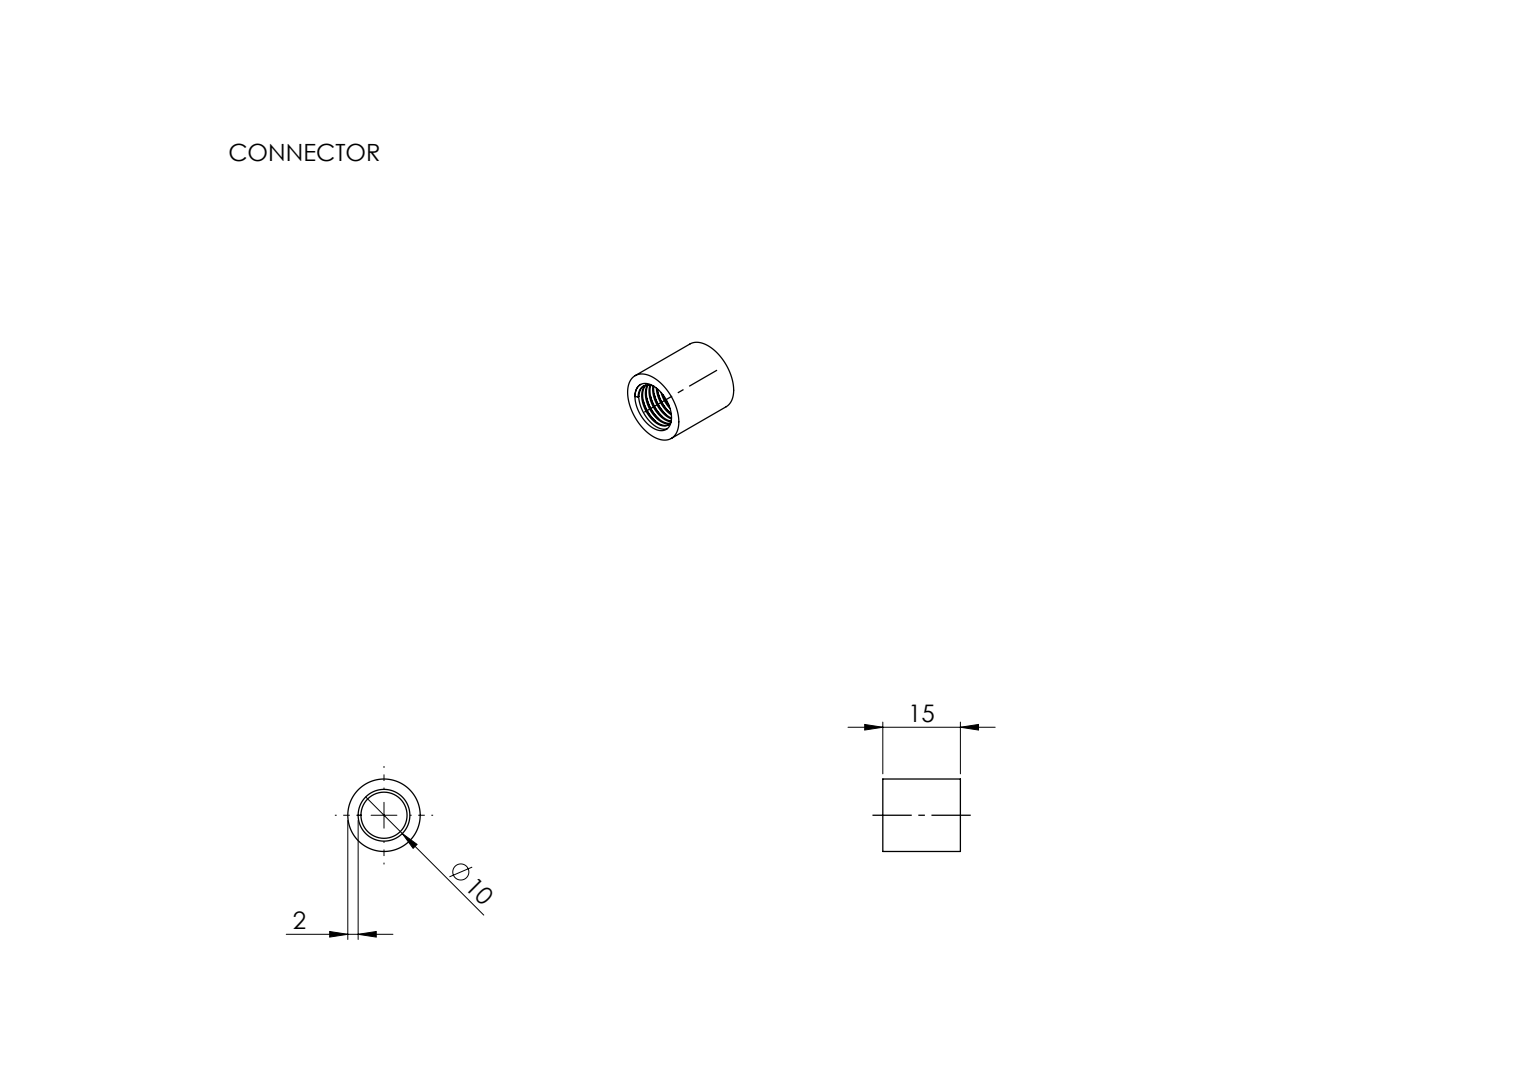
ISO-10303-21;
HEADER;
FILE_DESCRIPTION (('STEP AP214'),
    '1' );
FILE_NAME ('connector.step',
    '2026-10-01T14:18:43',
    ( '' ),
    ( '' ),
    'SwSTEP 2.0',
    'SolidWorks 2026',
    '' );
FILE_SCHEMA (( 'AUTOMOTIVE_DESIGN' ));
ENDSEC;

DATA;
#9=CARTESIAN_POINT ( 'NONE',  ( 101.8468681455906903, 4.458734125000016313, 4.375000001365592084 ) ) ;
#16=CARTESIAN_POINT ( 'NONE',  ( 94.99999999999995737, 1.387778780781445676E-14, 4.999999999999999112 ) ) ;
#25=CARTESIAN_POINT ( 'NONE',  ( 95.54126587499996504, 1.387778780781445676E-14, 10.68750000136559208 ) ) ;
#27=CARTESIAN_POINT ( 'NONE',  ( 99.99999999999995737, -4.458734124999988779, 1.687500001365591418 ) ) ;
#43=CARTESIAN_POINT ( 'NONE',  ( 104.4587341249999781, -1.846868145590721655, 14.12500000136559208 ) ) ;
#52=APPLICATION_CONTEXT ( 'automotive_design' ) ;
#61=CARTESIAN_POINT ( 'NONE',  ( 103.1528011352953342, -3.152801135295355106, 10.06250000136559386 ) ) ;
#74=CARTESIAN_POINT ( 'NONE',  ( 99.99999999999995737, -4.999999999999990230, 1.375000002731184612 ) ) ;
#80=EDGE_CURVE ( 'NONE', #16509, #7689, #8629, .T. ) ;
#91=CARTESIAN_POINT ( 'NONE',  ( 98.15313185440925281, 4.458734125000016313, 7.250000001365591196 ) ) ;
#94=CARTESIAN_POINT ( 'NONE',  ( 101.8468681455906903, -4.458734124999987891, 10.75000000136559208 ) ) ;
#102=CARTESIAN_POINT ( 'NONE',  ( 103.5355339059327093, 3.535533905932755072, 11.62500000000000000 ) ) ;
#104=CARTESIAN_POINT ( 'NONE',  ( 95.54126587499996504, 1.387778780781445676E-14, 0.6875000013655923059 ) ) ;
#107=DIRECTION ( 'NONE',  ( -1.000000000000000000, 0.000000000000000000, 0.000000000000000000 ) ) ;
#115=CARTESIAN_POINT ( 'NONE',  ( 102.0710678118654329, 5.000000000000018652, 4.687500000000000000 ) ) ;
#119=VECTOR ( 'NONE', #9370, 1000.000000000000000 ) ;
#132=CARTESIAN_POINT ( 'NONE',  ( 104.4587341249999781, 1.846868145590750521, 4.000000001365592084 ) ) ;
#150=CARTESIAN_POINT ( 'NONE',  ( 101.8468681455906903, -4.458734124999987891, 3.000000001365592528 ) ) ;
#162=VERTEX_POINT ( 'NONE', #19320 ) ;
#167=CARTESIAN_POINT ( 'NONE',  ( 96.84719886470459471, -3.152801135295355994, 12.81250000136559208 ) ) ;
#170=CARTESIAN_POINT ( 'NONE',  ( 103.1528011352953342, -3.152801135295355106, 0.8125000013655924169 ) ) ;
#172=CARTESIAN_POINT ( 'NONE',  ( 103.1528011352953342, -3.152801135295355106, 1.062500001365592528 ) ) ;
#177=ORIENTED_EDGE ( 'NONE', *, *, #19574, .T. ) ;
#201=CARTESIAN_POINT ( 'NONE',  ( 104.4587341249999781, -1.846868145590721655, 11.12500000136559208 ) ) ;
#207=CARTESIAN_POINT ( 'NONE',  ( 103.5355339059327093, -3.535533905932726206, 12.37499999999999822 ) ) ;
#219=FILL_AREA_STYLE ('',( #13008 ) ) ;
#227=VECTOR ( 'NONE', #13588, 1000.000000000000000 ) ;
#229=CARTESIAN_POINT ( 'NONE',  ( 95.54126587499995082, 1.846868145590750077, 10.37500000136559208 ) ) ;
#231=CARTESIAN_POINT ( 'NONE',  ( 95.54126587499995082, -1.846868145590724986, 13.50000000136559208 ) ) ;
#274=CARTESIAN_POINT ( 'NONE',  ( 99.99999999999995737, -4.458734124999988779, 1.687500001365591418 ) ) ;
#282=ORIENTED_EDGE ( 'NONE', *, *, #1152, .F. ) ;
#293=CARTESIAN_POINT ( 'NONE',  ( 101.8468681455906903, 4.458734125000016313, 3.375000001365592972 ) ) ;
#295=EDGE_LOOP ( 'NONE', ( #18742, #1157, #17267, #23427 ) ) ;
#309=CARTESIAN_POINT ( 'NONE',  ( 101.8468681455906903, -4.458734124999987891, 13.00000000136559386 ) ) ;
#311=CARTESIAN_POINT ( 'NONE',  ( 95.54126587499995082, -1.846868145590724986, 0.5000000013655920839 ) ) ;
#313=CARTESIAN_POINT ( 'NONE',  ( 104.9999999999999716, 1.449011120738813565E-14, 5.625000002731185056 ) ) ;
#328=CARTESIAN_POINT ( 'NONE',  ( 104.4587341249999781, -1.846868145590721655, 13.12500000136559208 ) ) ;
#345=CARTESIAN_POINT ( 'NONE',  ( 98.15313185440923860, -4.458734124999987891, 12.87500000136559208 ) ) ;
#374=ORIENTED_EDGE ( 'NONE', *, *, #22029, .T. ) ;
#375=CARTESIAN_POINT ( 'NONE',  ( 95.54126587499996504, 1.387778780781445676E-14, 7.437500001365592084 ) ) ;
#378=CARTESIAN_POINT ( 'NONE',  ( 95.54126587499995082, 1.846868145590750077, 7.375000001365592084 ) ) ;
#396=CARTESIAN_POINT ( 'NONE',  ( 99.99999999999995737, -4.999999999999990230, 10.37500000273118594 ) ) ;
#418=CARTESIAN_POINT ( 'NONE',  ( 101.8468681455907046, -4.458734124999987891, 3.750000001365591640 ) ) ;
#433=ORIENTED_EDGE ( 'NONE', *, *, #23597, .T. ) ;
#435=CARTESIAN_POINT ( 'NONE',  ( 96.46446609406721961, 3.535533905932755072, 11.87500000000000000 ) ) ;
#442=CARTESIAN_POINT ( 'NONE',  ( 99.99999999999995737, 1.387778780781445676E-14, 34.79898987322334136 ) ) ;
#452=CARTESIAN_POINT ( 'NONE',  ( 103.1528011352953342, 3.152801135295383084, 11.31250000136559386 ) ) ;
#454=CARTESIAN_POINT ( 'NONE',  ( 96.84719886470459471, -3.152801135295355994, 0.5625000013655921949 ) ) ;
#456=CARTESIAN_POINT ( 'NONE',  ( 101.8468681455907046, -4.458734124999987891, 1.000000001365592528 ) ) ;
#469=CARTESIAN_POINT ( 'NONE',  ( 104.4587341249999781, -1.846868145590721655, 12.12500000136559208 ) ) ;
#489=CARTESIAN_POINT ( 'NONE',  ( 98.15313185440923860, -4.458734124999987891, 11.87500000136559208 ) ) ;
#502=ORIENTED_EDGE ( 'NONE', *, *, #15207, .F. ) ;
#507=CARTESIAN_POINT ( 'NONE',  ( 94.99999999999995737, 1.387778780781445676E-14, 34.79898987322334136 ) ) ;
#509=CARTESIAN_POINT ( 'NONE',  ( 99.99999999999995737, -4.999999999999990230, 1.375000002731184612 ) ) ;
#514=DIRECTION ( 'NONE',  ( -1.000000000000000000, 0.000000000000000000, 0.000000000000000000 ) ) ;
#517=CARTESIAN_POINT ( 'NONE',  ( 95.54126587499995082, -1.846868145590724986, 3.500000001365591196 ) ) ;
#520=CARTESIAN_POINT ( 'NONE',  ( 95.54126587499995082, 1.846868145590750077, 9.375000001365592084 ) ) ;
#528=CARTESIAN_POINT ( 'NONE',  ( 104.9999999999999716, 1.449011120738813565E-14, 34.79898987322334136 ) ) ;
#532=ORIENTED_EDGE ( 'NONE', *, *, #5026, .F. ) ;
#537=CARTESIAN_POINT ( 'NONE',  ( 97.92893218813451028, -4.999999999999989342, 8.312500002731185944 ) ) ;
#579=( BOUNDED_SURFACE ( )  B_SPLINE_SURFACE ( 1, 2, ( 
 ( #14484, #7804, #25599, #1404, #3808, #3950, #3385, #8074, #3536, #18775, #16634, #25327, #10196, #25188, #14203, #7938, #27346, #18906, #19188, #18641, #12055, #16494, #27890, #10335, #5676, #23201, #25740, #23333, #27482, #12610, #10063, #23472, #8351, #5813, #14341, #23058, #6085, #12468, #12192, #16770, #12339, #3676, #20921, #27617, #1678, #5949, #25470, #21193, #14616, #9926, #19044, #20781, #1263, #27752, #8213, #16902, #1815, #10480, #17037, #6772, #21759, #11035, #19745, #26021, #26310, #229, #15029, #4507, #1950, #6629, #17754, #23747, #15458, #10757, #24172, #4649, #10620, #17327, #9059, #6223, #10898, #23610, #8915, #14890, #19469, #28029, #17604, #28168, #6492, #21903, #12882, #4087, #8636, #19325, #13164, #21612, #2377, #2088, #12751, #15168, #23887, #4365, #13308, #22035, #2511, #11172, #19606, #19891, #13022, #21474, #8495, #2236, #375, #17180, #4223, #91, #8772, #17461, #26163, #25886, #6355, #15314, #24029, #22176, #948, #26888, #2927, #15602, #3078, #6911, #2792, #20038, #11743, #11459, #18028, #13882, #4935, #24305, #20178, #11316, #24736, #13598, #5217, #22321, #1092, #662, #9335, #26742, #18324, #5359, #24880, #14025, #11597, #9619, #7184, #4791, #9759, #13738, #27031, #22750, #7046, #24598, #15882, #20319, #15744, #26457, #13449, #9475, #7477, #2655, #16172, #7334, #3216, #5077, #18177, #517, #9198, #17892, #11882, #22608, #22462, #20607, #807, #26600, #16023, #24449, #20469, #4163, #12025, #7904, #5778, #15100, #14967, #9896, #23686, #20749, #12688, #12958, #18607, #27442, #2165, #27965, #23026, #17258, #14305, #28103, #4300, #10031, #1233, #27312, #10692, #17111, #7769, #21413, #16599, #18743, #16456, #4022, #6290, #10556, #25151, #8421, #5641, #14170, #12160 ),
 ( #25815, #19398, #14447, #12823, #21549, #25291, #8567, #2023, #3496, #25958, #22888, #19266, #18469, #20886, #6431, #1370, #23822, #21692, #3353, #23545, #27176, #7628, #1892, #16320, #25021, #5502, #9133, #309, #2449, #6702, #167, #15823, #2593, #13095, #24529, #17969, #26243, #13385, #20116, #9273, #8849, #13240, #23964, #11397, #21836, #22257, #17687, #6845, #4872, #11254, #2732, #19973, #2312, #10969, #452, #21972, #4725, #26678, #11110, #4443, #594, #15390, #17826, #7126, #25, #22113, #17539, #24102, #19824, #8994, #26392, #19681, #10828, #4580, #15535, #24243, #5014, #15243, #19544, #26531, #6987, #15682, #24383, #13536, #13679, #22396, #8707, #17399, #26098, #6563, #14386, #7704, #12098, #5720, #9412, #16107, #16253, #7559, #18683, #20402, #5582, #25096, #7413, #22685, #2865, #1030, #24952, #15961, #3431, #20689, #18111, #1172, #24676, #887, #26825, #14247, #9701, #27386, #7271, #5438, #16398, #14106, #20548, #22969, #22829, #3296, #20825, #11966, #5154, #18402, #11535, #13959, #20251, #1302, #9971, #18544, #3155, #9837, #24811, #5295, #9558, #27248, #7845, #16540, #27108, #11825, #738, #25230, #13816, #22539, #3007, #11679, #18260, #26968, #27796, #7977, #23653, #12655, #10103, #21380, #16676, #12378, #18815, #6259, #21237, #10659, #1445, #8253, #27931, #6124, #12508, #14932, #14790, #23513, #4128, #3992, #27522, #1719, #25926, #5990, #3577, #8390, #1992, #10523, #23375, #1859, #8119, #27657, #1585, #19230, #16940, #17076, #10381, #25510, #23103, #25781, #19088, #12794, #25375, #21512, #25641, #5855, #19366, #28069, #14655, #18948, #21097, #8535, #17221, #14525, #6400, #12234, #10239, #20962, #23240, #3717, #16813, #3848, #16312, #15650, #26063, #26498, #21942, #11078, #9101 ) ),
 .UNSPECIFIED., .F., .F., .F. ) 
 B_SPLINE_SURFACE_WITH_KNOTS ( ( 2, 2 ),
 ( 3, 2, 2, 2, 2, 2, 2, 2, 2, 2, 2, 2, 2, 2, 2, 2, 2, 2, 2, 2, 2, 2, 2, 2, 2, 2, 2, 2, 2, 2, 2, 2, 2, 2, 2, 2, 2, 2, 2, 2, 2, 2, 2, 2, 2, 2, 2, 2, 2, 2, 2, 2, 2, 2, 2, 2, 2, 2, 2, 2, 2, 2, 2, 2, 2, 2, 2, 2, 2, 2, 2, 2, 2, 2, 2, 2, 2, 2, 2, 2, 2, 2, 2, 2, 2, 2, 2, 2, 2, 2, 2, 2, 2, 2, 2, 2, 2, 2, 2, 2, 2, 2, 2, 2, 2, 2, 2, 2, 2, 2, 2, 2, 3 ),
 ( 0.000000000000000000, 1.000000000000000000 ),
 ( 0.000000000000000000, 0.008928571428571428076, 0.01785714285714285615, 0.02678571428571428423, 0.03571428571428571230, 0.04464285714285714385, 0.05357142857142856845, 0.06250000000000000000, 0.07142857142857142461, 0.08035714285714286309, 0.08928571428571428770, 0.09821428571428571230, 0.1071428571428571369, 0.1160714285714285754, 0.1250000000000000000, 0.1339285714285714246, 0.1428571428571428492, 0.1517857142857142738, 0.1607142857142857262, 0.1696428571428571508, 0.1785714285714285754, 0.1875000000000000000, 0.1964285714285714246, 0.2053571428571428492, 0.2142857142857142738, 0.2232142857142857262, 0.2321428571428571508, 0.2410714285714285754, 0.2500000000000000000, 0.2589285714285714524, 0.2678571428571428492, 0.2767857142857143016, 0.2857142857142856984, 0.2946428571428571508, 0.3035714285714285476, 0.3125000000000000000, 0.3214285714285714524, 0.3303571428571428492, 0.3392857142857143016, 0.3482142857142856984, 0.3571428571428571508, 0.3660714285714285476, 0.3750000000000000000, 0.3839285714285714524, 0.3928571428571428492, 0.4017857142857143016, 0.4107142857142856984, 0.4196428571428571508, 0.4285714285714285476, 0.4375000000000000000, 0.4464285714285714524, 0.4553571428571428492, 0.4642857142857143016, 0.4732142857142856984, 0.4821428571428571508, 0.4910714285714285476, 0.5000000000000000000, 0.5089285714285713969, 0.5178571428571429047, 0.5267857142857143016, 0.5357142857142856984, 0.5446428571428570953, 0.5535714285714286031, 0.5625000000000000000, 0.5714285714285713969, 0.5803571428571429047, 0.5892857142857143016, 0.5982142857142856984, 0.6071428571428570953, 0.6160714285714286031, 0.6250000000000000000, 0.6339285714285713969, 0.6428571428571429047, 0.6517857142857143016, 0.6607142857142856984, 0.6696428571428570953, 0.6785714285714286031, 0.6875000000000000000, 0.6964285714285713969, 0.7053571428571429047, 0.7142857142857143016, 0.7232142857142856984, 0.7321428571428570953, 0.7410714285714286031, 0.7500000000000000000, 0.7589285714285713969, 0.7678571428571429047, 0.7767857142857143016, 0.7857142857142856984, 0.7946428571428570953, 0.8035714285714286031, 0.8125000000000000000, 0.8214285714285713969, 0.8303571428571429047, 0.8392857142857143016, 0.8482142857142856984, 0.8571428571428570953, 0.8660714285714286031, 0.8750000000000000000, 0.8839285714285713969, 0.8928571428571429047, 0.9017857142857143016, 0.9107142857142856984, 0.9196428571428570953, 0.9285714285714286031, 0.9375000000000000000, 0.9464285714285713969, 0.9553571428571429047, 0.9642857142857143016, 0.9732142857142856984, 0.9821428571428570953, 0.9910714285714286031, 1.000000000000000000 ),
 .UNSPECIFIED. ) 
 GEOMETRIC_REPRESENTATION_ITEM ( )  RATIONAL_B_SPLINE_SURFACE ( (
 ( 1.000000000000000000, 0.9238795325112867385, 1.000000000000000000, 0.9238795325112867385, 1.000000000000000000, 0.9238795325112867385, 1.000000000000000000, 0.9238795325112867385, 1.000000000000000000, 0.9238795325112867385, 1.000000000000000000, 0.9238795325112867385, 1.000000000000000000, 0.9238795325112867385, 1.000000000000000000, 0.9238795325112867385, 1.000000000000000000, 0.9238795325112867385, 1.000000000000000000, 0.9238795325112867385, 1.000000000000000000, 0.9238795325112867385, 1.000000000000000000, 0.9238795325112867385, 1.000000000000000000, 0.9238795325112867385, 1.000000000000000000, 0.9238795325112867385, 1.000000000000000000, 0.9238795325112867385, 1.000000000000000000, 0.9238795325112867385, 1.000000000000000000, 0.9238795325112867385, 1.000000000000000000, 0.9238795325112867385, 1.000000000000000000, 0.9238795325112867385, 1.000000000000000000, 0.9238795325112867385, 1.000000000000000000, 0.9238795325112867385, 1.000000000000000000, 0.9238795325112867385, 1.000000000000000000, 0.9238795325112867385, 1.000000000000000000, 0.9238795325112867385, 1.000000000000000000, 0.9238795325112867385, 1.000000000000000000, 0.9238795325112867385, 1.000000000000000000, 0.9238795325112867385, 1.000000000000000000, 0.9238795325112867385, 1.000000000000000000, 0.9238795325112867385, 1.000000000000000000, 0.9238795325112867385, 1.000000000000000000, 0.9238795325112867385, 1.000000000000000000, 0.9238795325112867385, 1.000000000000000000, 0.9238795325112867385, 1.000000000000000000, 0.9238795325112867385, 1.000000000000000000, 0.9238795325112867385, 1.000000000000000000, 0.9238795325112867385, 1.000000000000000000, 0.9238795325112867385, 1.000000000000000000, 0.9238795325112867385, 1.000000000000000000, 0.9238795325112867385, 1.000000000000000000, 0.9238795325112867385, 1.000000000000000000, 0.9238795325112867385, 1.000000000000000000, 0.9238795325112867385, 1.000000000000000000, 0.9238795325112867385, 1.000000000000000000, 0.9238795325112867385, 1.000000000000000000, 0.9238795325112867385, 1.000000000000000000, 0.9238795325112867385, 1.000000000000000000, 0.9238795325112867385, 1.000000000000000000, 0.9238795325112867385, 1.000000000000000000, 0.9238795325112867385, 1.000000000000000000, 0.9238795325112867385, 1.000000000000000000, 0.9238795325112867385, 1.000000000000000000, 0.9238795325112867385, 1.000000000000000000, 0.9238795325112867385, 1.000000000000000000, 0.9238795325112867385, 1.000000000000000000, 0.9238795325112867385, 1.000000000000000000, 0.9238795325112867385, 1.000000000000000000, 0.9238795325112867385, 1.000000000000000000, 0.9238795325112867385, 1.000000000000000000, 0.9238795325112867385, 1.000000000000000000, 0.9238795325112867385, 1.000000000000000000, 0.9238795325112867385, 1.000000000000000000, 0.9238795325112867385, 1.000000000000000000, 0.9238795325112867385, 1.000000000000000000, 0.9238795325112867385, 1.000000000000000000, 0.9238795325112867385, 1.000000000000000000, 0.9238795325112867385, 1.000000000000000000, 0.9238795325112867385, 1.000000000000000000, 0.9238795325112867385, 1.000000000000000000, 0.9238795325112867385, 1.000000000000000000, 0.9238795325112867385, 1.000000000000000000, 0.9238795325112867385, 1.000000000000000000, 0.9238795325112867385, 1.000000000000000000, 0.9238795325112867385, 1.000000000000000000, 0.9238795325112867385, 1.000000000000000000, 0.9238795325112867385, 1.000000000000000000, 0.9238795325112867385, 1.000000000000000000, 0.9238795325112867385, 1.000000000000000000, 0.9238795325112867385, 1.000000000000000000, 0.9238795325112867385, 1.000000000000000000, 0.9238795325112867385, 1.000000000000000000, 0.9238795325112867385, 1.000000000000000000, 0.9238795325112867385, 1.000000000000000000, 0.9238795325112867385, 1.000000000000000000, 0.9238795325112867385, 1.000000000000000000, 0.9238795325112867385, 1.000000000000000000, 0.9238795325112867385, 1.000000000000000000, 0.9238795325112867385, 1.000000000000000000, 0.9238795325112867385, 1.000000000000000000, 0.9238795325112867385, 1.000000000000000000, 0.9238795325112867385, 1.000000000000000000, 0.9238795325112867385, 1.000000000000000000, 0.9238795325112867385, 1.000000000000000000, 0.9238795325112867385, 1.000000000000000000, 0.9238795325112867385, 1.000000000000000000, 0.9238795325112867385, 1.000000000000000000, 0.9238795325112867385, 1.000000000000000000, 0.9238795325112867385, 1.000000000000000000, 0.9238795325112867385, 1.000000000000000000, 0.9238795325112867385, 1.000000000000000000, 0.9238795325112867385, 1.000000000000000000, 0.9238795325112867385, 1.000000000000000000, 0.9238795325112867385, 1.000000000000000000, 0.9238795325112867385, 1.000000000000000000, 0.9238795325112867385, 1.000000000000000000, 0.9238795325112867385, 1.000000000000000000, 0.9238795325112867385, 1.000000000000000000, 0.9238795325112867385, 1.000000000000000000, 0.9238795325112867385, 1.000000000000000000, 0.9238795325112867385, 1.000000000000000000, 0.9238795325112867385, 1.000000000000000000, 0.9238795325112867385, 1.000000000000000000, 0.9238795325112867385, 1.000000000000000000),
 ( 1.000000000000000000, 0.9238795325112867385, 1.000000000000000000, 0.9238795325112867385, 1.000000000000000000, 0.9238795325112867385, 1.000000000000000000, 0.9238795325112867385, 1.000000000000000000, 0.9238795325112867385, 1.000000000000000000, 0.9238795325112867385, 1.000000000000000000, 0.9238795325112867385, 1.000000000000000000, 0.9238795325112867385, 1.000000000000000000, 0.9238795325112867385, 1.000000000000000000, 0.9238795325112867385, 1.000000000000000000, 0.9238795325112867385, 1.000000000000000000, 0.9238795325112867385, 1.000000000000000000, 0.9238795325112867385, 1.000000000000000000, 0.9238795325112867385, 1.000000000000000000, 0.9238795325112867385, 1.000000000000000000, 0.9238795325112867385, 1.000000000000000000, 0.9238795325112867385, 1.000000000000000000, 0.9238795325112867385, 1.000000000000000000, 0.9238795325112867385, 1.000000000000000000, 0.9238795325112867385, 1.000000000000000000, 0.9238795325112867385, 1.000000000000000000, 0.9238795325112867385, 1.000000000000000000, 0.9238795325112867385, 1.000000000000000000, 0.9238795325112867385, 1.000000000000000000, 0.9238795325112867385, 1.000000000000000000, 0.9238795325112867385, 1.000000000000000000, 0.9238795325112867385, 1.000000000000000000, 0.9238795325112867385, 1.000000000000000000, 0.9238795325112867385, 1.000000000000000000, 0.9238795325112867385, 1.000000000000000000, 0.9238795325112867385, 1.000000000000000000, 0.9238795325112867385, 1.000000000000000000, 0.9238795325112867385, 1.000000000000000000, 0.9238795325112867385, 1.000000000000000000, 0.9238795325112867385, 1.000000000000000000, 0.9238795325112867385, 1.000000000000000000, 0.9238795325112867385, 1.000000000000000000, 0.9238795325112867385, 1.000000000000000000, 0.9238795325112867385, 1.000000000000000000, 0.9238795325112867385, 1.000000000000000000, 0.9238795325112867385, 1.000000000000000000, 0.9238795325112867385, 1.000000000000000000, 0.9238795325112867385, 1.000000000000000000, 0.9238795325112867385, 1.000000000000000000, 0.9238795325112867385, 1.000000000000000000, 0.9238795325112867385, 1.000000000000000000, 0.9238795325112867385, 1.000000000000000000, 0.9238795325112867385, 1.000000000000000000, 0.9238795325112867385, 1.000000000000000000, 0.9238795325112867385, 1.000000000000000000, 0.9238795325112867385, 1.000000000000000000, 0.9238795325112867385, 1.000000000000000000, 0.9238795325112867385, 1.000000000000000000, 0.9238795325112867385, 1.000000000000000000, 0.9238795325112867385, 1.000000000000000000, 0.9238795325112867385, 1.000000000000000000, 0.9238795325112867385, 1.000000000000000000, 0.9238795325112867385, 1.000000000000000000, 0.9238795325112867385, 1.000000000000000000, 0.9238795325112867385, 1.000000000000000000, 0.9238795325112867385, 1.000000000000000000, 0.9238795325112867385, 1.000000000000000000, 0.9238795325112867385, 1.000000000000000000, 0.9238795325112867385, 1.000000000000000000, 0.9238795325112867385, 1.000000000000000000, 0.9238795325112867385, 1.000000000000000000, 0.9238795325112867385, 1.000000000000000000, 0.9238795325112867385, 1.000000000000000000, 0.9238795325112867385, 1.000000000000000000, 0.9238795325112867385, 1.000000000000000000, 0.9238795325112867385, 1.000000000000000000, 0.9238795325112867385, 1.000000000000000000, 0.9238795325112867385, 1.000000000000000000, 0.9238795325112867385, 1.000000000000000000, 0.9238795325112867385, 1.000000000000000000, 0.9238795325112867385, 1.000000000000000000, 0.9238795325112867385, 1.000000000000000000, 0.9238795325112867385, 1.000000000000000000, 0.9238795325112867385, 1.000000000000000000, 0.9238795325112867385, 1.000000000000000000, 0.9238795325112867385, 1.000000000000000000, 0.9238795325112867385, 1.000000000000000000, 0.9238795325112867385, 1.000000000000000000, 0.9238795325112867385, 1.000000000000000000, 0.9238795325112867385, 1.000000000000000000, 0.9238795325112867385, 1.000000000000000000, 0.9238795325112867385, 1.000000000000000000, 0.9238795325112867385, 1.000000000000000000, 0.9238795325112867385, 1.000000000000000000, 0.9238795325112867385, 1.000000000000000000, 0.9238795325112867385, 1.000000000000000000, 0.9238795325112867385, 1.000000000000000000, 0.9238795325112867385, 1.000000000000000000, 0.9238795325112867385, 1.000000000000000000, 0.9238795325112867385, 1.000000000000000000, 0.9238795325112867385, 1.000000000000000000, 0.9238795325112867385, 1.000000000000000000, 0.9238795325112867385, 1.000000000000000000, 0.9238795325112867385, 1.000000000000000000, 0.9238795325112867385, 1.000000000000000000, 0.9238795325112867385, 1.000000000000000000, 0.9238795325112867385, 1.000000000000000000, 0.9238795325112867385, 1.000000000000000000, 0.9238795325112867385, 1.000000000000000000, 0.9238795325112867385, 1.000000000000000000, 0.9238795325112867385, 1.000000000000000000, 0.9238795325112867385, 1.000000000000000000, 0.9238795325112867385, 1.000000000000000000, 0.9238795325112867385, 1.000000000000000000, 0.9238795325112867385, 1.000000000000000000, 0.9238795325112867385, 1.000000000000000000, 0.9238795325112867385, 1.000000000000000000) ) ) 
 REPRESENTATION_ITEM ( '' )  SURFACE ( )  );
#582=CARTESIAN_POINT ( 'NONE',  ( 102.0710678118654329, -4.999999999999989342, 12.31249999999999822 ) ) ;
#594=CARTESIAN_POINT ( 'NONE',  ( 99.99999999999995737, -4.458734124999988779, 10.93750000136559208 ) ) ;
#596=CARTESIAN_POINT ( 'NONE',  ( 98.15313185440923860, 4.458734125000016313, 14.25000000136559208 ) ) ;
#599=FACE_OUTER_BOUND ( 'NONE', #17431, .T. ) ;
#612=CARTESIAN_POINT ( 'NONE',  ( 101.8468681455906903, -4.458734124999987891, 9.000000001365593860 ) ) ;
#630=CARTESIAN_POINT ( 'NONE',  ( 99.99999999999995737, -4.458734124999988779, 7.937500001365592084 ) ) ;
#632=ADVANCED_FACE ( 'NONE', ( #6014 ), #27956, .F. ) ;
#651=CARTESIAN_POINT ( 'NONE',  ( 96.46446609406721961, 3.535533905932755072, 11.00000000273118594 ) ) ;
#653=CARTESIAN_POINT ( 'NONE',  ( 99.99999999999995737, -4.999999999999990230, 5.375000002731185056 ) ) ;
#662=CARTESIAN_POINT ( 'NONE',  ( 95.54126587499995082, 1.846868145590750077, 5.375000001365592972 ) ) ;
#665=CARTESIAN_POINT ( 'NONE',  ( 95.54126587499995082, 1.846868145590750077, 6.375000001365592084 ) ) ;
#668=CYLINDRICAL_SURFACE ( 'NONE', #16059, 5.000000000000004441 ) ;
#682=CARTESIAN_POINT ( 'NONE',  ( 104.9999999999999716, 1.449011120738813565E-14, 9.625000002731184168 ) ) ;
#687=CARTESIAN_POINT ( 'NONE',  ( 99.99999999999995737, 5.000000000000018652, 2.749999999999999112 ) ) ;
#725=CARTESIAN_POINT ( 'NONE',  ( 104.9999999999999716, 1.449011120738813565E-14, 11.50000000000000000 ) ) ;
#738=CARTESIAN_POINT ( 'NONE',  ( 96.84719886470459471, 3.152801135295383084, 5.562500001365592972 ) ) ;
#740=CARTESIAN_POINT ( 'NONE',  ( 96.84719886470459471, 3.152801135295383084, 11.31250000136559208 ) ) ;
#755=CARTESIAN_POINT ( 'NONE',  ( 101.8468681455906903, -4.458734124999987891, 10.00000000136559386 ) ) ;
#773=CARTESIAN_POINT ( 'NONE',  ( 101.8468681455907046, 4.458734125000016313, 6.375000001365592084 ) ) ;
#777=CARTESIAN_POINT ( 'NONE',  ( 94.99999999999994316, -2.071067811865454633, 14.06249999999999645 ) ) ;
#803=FACE_OUTER_BOUND ( 'NONE', #4700, .T. ) ;
#807=CARTESIAN_POINT ( 'NONE',  ( 103.1528011352953342, 3.152801135295383084, 3.062500001365592528 ) ) ;
#810=CARTESIAN_POINT ( 'NONE',  ( 104.4587341249999781, 1.846868145590750299, 10.00000000136559208 ) ) ;
#829=CARTESIAN_POINT ( 'NONE',  ( 97.92893218813451028, -4.999999999999989342, 9.312500002731184168 ) ) ;
#835=CARTESIAN_POINT ( 'NONE',  ( 102.0710678118654329, 5.000000000000018652, 1.687499999999999778 ) ) ;
#843=DIRECTION ( 'NONE',  ( 0.000000000000000000, 0.000000000000000000, 1.000000000000000000 ) ) ;
#844=CARTESIAN_POINT ( 'NONE',  ( 94.99999999999995737, 1.387778780781445676E-14, 34.79898987322334136 ) ) ;
#874=CARTESIAN_POINT ( 'NONE',  ( 103.5355339059327093, -3.535533905932726206, 13.37500000000000000 ) ) ;
#875=EDGE_LOOP ( 'NONE', ( #22304, #6186, #9476, #20532 ) ) ;
#887=CARTESIAN_POINT ( 'NONE',  ( 95.54126587499995082, 1.846868145590750077, 7.625000001365592084 ) ) ;
#889=CARTESIAN_POINT ( 'NONE',  ( 99.99999999999995737, 4.458734125000016313, 9.187500001365592084 ) ) ;
#896=VERTEX_POINT ( 'NONE', #16 ) ;
#901=ORIENTED_EDGE ( 'NONE', *, *, #24657, .T. ) ;
#903=CARTESIAN_POINT ( 'NONE',  ( 99.99999999999995737, -4.458734124999988779, 8.937500001365592084 ) ) ;
#918=CARTESIAN_POINT ( 'NONE',  ( 98.15313185440923860, 4.458734125000016313, 6.500000001365592084 ) ) ;
#929=ORIENTED_EDGE ( 'NONE', *, *, #10839, .T. ) ;
#943=CARTESIAN_POINT ( 'NONE',  ( 96.46446609406721961, -3.535533905932727539, 7.124999999999999112 ) ) ;
#946=AXIS2_PLACEMENT_3D ( 'NONE', #27552, #14136, #5889 ) ;
#948=CARTESIAN_POINT ( 'NONE',  ( 99.99999999999995737, -4.458734124999988779, 6.687500001365592084 ) ) ;
#949=VERTEX_POINT ( 'NONE', #9403 ) ;
#951=CARTESIAN_POINT ( 'NONE',  ( 101.8468681455906903, 4.458734125000016313, 9.125000001365592084 ) ) ;
#965=CARTESIAN_POINT ( 'NONE',  ( 94.99999999999995737, 1.387778780781445676E-14, 8.000000000000000000 ) ) ;
#969=CARTESIAN_POINT ( 'NONE',  ( 99.99999999999995737, -4.999999999999990230, 8.375000002731185944 ) ) ;
#982=CARTESIAN_POINT ( 'NONE',  ( 104.9999999999999716, 1.449011120738813565E-14, 5.625000002731185056 ) ) ;
#1015=DIRECTION ( 'NONE',  ( -0.000000000000000000, -0.000000000000000000, -1.000000000000000000 ) ) ;
#1017=CARTESIAN_POINT ( 'NONE',  ( 103.5355339059327093, 3.535533905932755072, 13.62500000000000000 ) ) ;
#1022=CARTESIAN_POINT ( 'NONE',  ( 94.99999999999995737, 1.387778780781445676E-14, 13.12500000273118417 ) ) ;
#1023=CARTESIAN_POINT ( 'NONE',  ( 97.92893218813451028, -4.999999999999989342, 3.187499999999999556 ) ) ;
#1030=CARTESIAN_POINT ( 'NONE',  ( 104.4587341249999781, -1.846868145590721655, 8.125000001365592084 ) ) ;
#1032=CARTESIAN_POINT ( 'NONE',  ( 103.1528011352953342, 3.152801135295383084, 10.06250000136559208 ) ) ;
#1034=CARTESIAN_POINT ( 'NONE',  ( 104.9999999999999716, 1.449011120738813565E-14, 4.499999999999999112 ) ) ;
#1038=ORIENTED_EDGE ( 'NONE', *, *, #17393, .T. ) ;
#1043=ORIENTED_EDGE ( 'NONE', *, *, #5070, .F. ) ;
#1045=CARTESIAN_POINT ( 'NONE',  ( 98.15313185440925281, 4.458734125000016313, 12.50000000136559208 ) ) ;
#1057=VECTOR ( 'NONE', #15274, 1000.000000000000000 ) ;
#1061=CARTESIAN_POINT ( 'NONE',  ( 101.8468681455907046, 4.458734125000016313, 5.375000001365592972 ) ) ;
#1066=ORIENTED_EDGE ( 'NONE', *, *, #26446, .F. ) ;
#1078=AXIS2_PLACEMENT_3D ( 'NONE', #23281, #14280, #24991 ) ;
#1092=CARTESIAN_POINT ( 'NONE',  ( 95.54126587499996504, 1.387778780781445676E-14, 5.437500001365591196 ) ) ;
#1093=CARTESIAN_POINT ( 'NONE',  ( 102.0710678118654329, 5.000000000000018652, 12.81250000273118772 ) ) ;
#1094=CARTESIAN_POINT ( 'NONE',  ( 101.8468681455906903, -4.458734124999987891, 2.750000001365592084 ) ) ;
#1111=CARTESIAN_POINT ( 'NONE',  ( 99.99999999999995737, -4.999999999999990230, 5.375000002731185056 ) ) ;
#1114=CARTESIAN_POINT ( 'NONE',  ( 104.9999999999999858, 2.071067811865485719, 14.56249999999999822 ) ) ;
#1132=ADVANCED_FACE ( 'NONE', ( #5008 ), #13671, .F. ) ;
#1146=ORIENTED_EDGE ( 'NONE', *, *, #5026, .T. ) ;
#1152=EDGE_CURVE ( 'NONE', #6963, #2879, #8797, .T. ) ;
#1157=ORIENTED_EDGE ( 'NONE', *, *, #6712, .F. ) ;
#1158=CARTESIAN_POINT ( 'NONE',  ( 96.46446609406721961, 3.535533905932755072, 7.875000000000000000 ) ) ;
#1162=CARTESIAN_POINT ( 'NONE',  ( 104.9999999999999858, 2.071067811865485719, 13.68750000273118417 ) ) ;
#1163=CARTESIAN_POINT ( 'NONE',  ( 96.46446609406721961, 3.535533905932755072, 14.00000000273118594 ) ) ;
#1169=ADVANCED_FACE ( 'NONE', ( #7696 ), #11699, .F. ) ;
#1172=CARTESIAN_POINT ( 'NONE',  ( 95.54126587499995082, -1.846868145590724986, 7.750000001365592084 ) ) ;
#1173=CARTESIAN_POINT ( 'NONE',  ( 94.99999999999995737, 1.387778780781445676E-14, 15.00000000000000000 ) ) ;
#1174=CARTESIAN_POINT ( 'NONE',  ( 95.54126587499996504, -1.846868145590724986, 11.50000000136559208 ) ) ;
#1180=EDGE_CURVE ( 'NONE', #27294, #8379, #26712, .T. ) ;
#1181=ORIENTED_EDGE ( 'NONE', *, *, #10839, .F. ) ;
#1188=CARTESIAN_POINT ( 'NONE',  ( 98.15313185440925281, -4.458734124999987891, 5.875000001365591196 ) ) ;
#1202=CARTESIAN_POINT ( 'NONE',  ( 96.84719886470459471, -3.152801135295355994, 5.812500001365591196 ) ) ;
#1204=CARTESIAN_POINT ( 'NONE',  ( 104.9999999999999716, 1.449011120738813565E-14, 6.625000002731185944 ) ) ;
#1212=CARTESIAN_POINT ( 'NONE',  ( 94.99999999999995737, -2.071067811865466624, 3.187500002731184612 ) ) ;
#1219=CARTESIAN_POINT ( 'NONE',  ( 94.99999999999995737, 1.387778780781445676E-14, 0.1250000027311851669 ) ) ;
#1233=CARTESIAN_POINT ( 'NONE',  ( 95.54126587499996504, 1.387778780781445676E-14, 1.437500001365591196 ) ) ;
#1248=CARTESIAN_POINT ( 'NONE',  ( 104.9999999999999574, 2.071067811865491937, 3.687500002731185056 ) ) ;
#1263=CARTESIAN_POINT ( 'NONE',  ( 99.99999999999995737, 4.458734125000016313, 11.18750000136559208 ) ) ;
#1270=CARTESIAN_POINT ( 'NONE',  ( 104.9999999999999716, 1.449011120738813565E-14, 2.625000002731185500 ) ) ;
#1288=CARTESIAN_POINT ( 'NONE',  ( 96.46446609406721961, -3.535533905932727539, 10.12499999999999822 ) ) ;
#1292=CARTESIAN_POINT ( 'NONE',  ( 103.5355339059327093, 3.535533905932755072, 13.75000000273118594 ) ) ;
#1293=CARTESIAN_POINT ( 'NONE',  ( 96.46446609406721961, -3.535533905932727539, 13.25000000273118417 ) ) ;
#1302=CARTESIAN_POINT ( 'NONE',  ( 101.8468681455906903, 4.458734125000016313, 6.375000001365592084 ) ) ;
#1304=CARTESIAN_POINT ( 'NONE',  ( 103.1528011352953342, 3.152801135295383084, 9.062500001365592084 ) ) ;
#1307=CARTESIAN_POINT ( 'NONE',  ( 96.46446609406721961, -3.535533905932727539, 4.124999999999998224 ) ) ;
#1320=CARTESIAN_POINT ( 'NONE',  ( 95.54126587499995082, 1.846868145590750077, 5.625000001365593860 ) ) ;
#1331=VECTOR ( 'NONE', #22313, 1000.000000000000000 ) ;
#1334=EDGE_CURVE ( 'NONE', #22247, #2357, #13649, .T. ) ;
#1338=CARTESIAN_POINT ( 'NONE',  ( 103.1528011352953342, 3.152801135295383084, 2.312500001365592084 ) ) ;
#1347=CARTESIAN_POINT ( 'NONE',  ( 97.92893218813451028, -4.999999999999989342, 3.312500002731184612 ) ) ;
#1350=FACE_OUTER_BOUND ( 'NONE', #4598, .T. ) ;
#1356=CARTESIAN_POINT ( 'NONE',  ( 94.99999999999995737, 1.387778780781445676E-14, 1.999999999999998224 ) ) ;
#1359=ORIENTED_EDGE ( 'NONE', *, *, #24123, .F. ) ;
#1370=CARTESIAN_POINT ( 'NONE',  ( 95.54126587499995082, -1.846868145590724986, 13.75000000136559208 ) ) ;
#1387=CARTESIAN_POINT ( 'NONE',  ( 96.46446609406721961, -3.535533905932727539, 7.250000002731185056 ) ) ;
#1404=CARTESIAN_POINT ( 'NONE',  ( 98.15313185440925281, 4.458734125000016313, 14.25000000136559208 ) ) ;
#1405=CARTESIAN_POINT ( 'NONE',  ( 94.99999999999994316, -2.071067811865454633, 13.18750000273118594 ) ) ;
#1429=CARTESIAN_POINT ( 'NONE',  ( 103.5355339059327093, 3.535533905932755072, 7.624999999999999112 ) ) ;
#1435=CARTESIAN_POINT ( 'NONE',  ( 104.9999999999999716, 1.449011120738813565E-14, 12.62500000273118594 ) ) ;
#1445=CARTESIAN_POINT ( 'NONE',  ( 103.1528011352953342, 3.152801135295383084, 4.312500001365592084 ) ) ;
#1448=CARTESIAN_POINT ( 'NONE',  ( 98.15313185440923860, -4.458734124999987891, 5.625000001365591196 ) ) ;
#1460=CARTESIAN_POINT ( 'NONE',  ( 104.4587341249999639, 1.442382525525748735E-14, 7.187500001365592972 ) ) ;
#1465=CARTESIAN_POINT ( 'NONE',  ( 104.9999999999999716, 1.449011120738813565E-14, 34.79898987322334136 ) ) ;
#1475=CARTESIAN_POINT ( 'NONE',  ( 101.8468681455907046, -4.458734124999987891, 4.000000001365592084 ) ) ;
#1482=EDGE_CURVE ( 'NONE', #4790, #7853, #17201, .T. ) ;
#1489=ORIENTED_EDGE ( 'NONE', *, *, #5307, .T. ) ;
#1501=( BOUNDED_CURVE ( )  B_SPLINE_CURVE ( 2, ( #1852, #10515, #4538, #21934, #6393, #26055, #11071, #23778, #19781 ),
 .UNSPECIFIED., .F., .F. ) 
 B_SPLINE_CURVE_WITH_KNOTS ( ( 3, 2, 2, 2, 3 ),
 ( 0.5714285714285713969, 0.5803571428571429047, 0.5892857142857143016, 0.5982142857142856984, 0.6071428571428570953 ),
 .UNSPECIFIED. ) 
 CURVE ( )  GEOMETRIC_REPRESENTATION_ITEM ( )  RATIONAL_B_SPLINE_CURVE ( ( 1.000000000000000000, 0.9238795325112867385, 1.000000000000000000, 0.9238795325112867385, 1.000000000000000000, 0.9238795325112867385, 1.000000000000000000, 0.9238795325112867385, 1.000000000000000000 ) ) 
 REPRESENTATION_ITEM ( '' )  );
#1507=ORIENTED_EDGE ( 'NONE', *, *, #23758, .T. ) ;
#1521=PRODUCT_DEFINITION_CONTEXT ( 'detailed design', #52, 'design' ) ;
#1525=CARTESIAN_POINT ( 'NONE',  ( 97.92893218813451028, 5.000000000000018652, 5.937500002731185056 ) ) ;
#1544=CARTESIAN_POINT ( 'NONE',  ( 103.5355339059327093, 3.535533905932755072, 12.62499999999999822 ) ) ;
#1552=CARTESIAN_POINT ( 'NONE',  ( 102.0710678118654329, 5.000000000000018652, 2.812500002731185944 ) ) ;
#1571=CARTESIAN_POINT ( 'NONE',  ( 104.9999999999999574, 2.071067811865491937, 9.562499999999998224 ) ) ;
#1578=CARTESIAN_POINT ( 'NONE',  ( 94.99999999999995737, -2.071067811865466624, 11.06250000000000000 ) ) ;
#1580=( BOUNDED_CURVE ( )  B_SPLINE_CURVE ( 2, ( #24727, #5206, #13870, #3204, #7466, #18312, #22597, #22310, #9324 ),
 .UNSPECIFIED., .F., .T. ) 
 B_SPLINE_CURVE_WITH_KNOTS ( ( 3, 2, 2, 2, 3 ),
 ( 0.1071428571428571092, 0.1160714285714285476, 0.1249999999999999861, 0.1339285714285714246, 0.1428571428571428492 ),
 .UNSPECIFIED. ) 
 CURVE ( )  GEOMETRIC_REPRESENTATION_ITEM ( )  RATIONAL_B_SPLINE_CURVE ( ( 1.000000000000000222, 0.9238795325112865164, 1.000000000000000000, 0.9238795325112867385, 1.000000000000000000, 0.9238795325112867385, 1.000000000000000000, 0.9238795325112867385, 1.000000000000000000 ) ) 
 REPRESENTATION_ITEM ( '' )  );
#1585=CARTESIAN_POINT ( 'NONE',  ( 99.99999999999995737, -4.458734124999988779, 2.937500001365592528 ) ) ;
#1587=CARTESIAN_POINT ( 'NONE',  ( 95.54126587499996504, 1.387778780781445676E-14, 4.437500001365592084 ) ) ;
#1599=CARTESIAN_POINT ( 'NONE',  ( 104.4587341249999639, 1.442382525525748735E-14, 8.187500001365592084 ) ) ;
#1613=CARTESIAN_POINT ( 'NONE',  ( 95.54126587499995082, -1.846868145590724986, 5.500000001365591196 ) ) ;
#1615=CARTESIAN_POINT ( 'NONE',  ( 98.15313185440923860, 4.458734125000016313, 2.500000001365592084 ) ) ;
#1624=DIRECTION ( 'NONE',  ( -0.000000000000000000, -0.000000000000000000, -1.000000000000000000 ) ) ;
#1643=CARTESIAN_POINT ( 'NONE',  ( 104.9999999999999716, 1.449011120738813565E-14, 34.79898987322334136 ) ) ;
#1644=CARTESIAN_POINT ( 'NONE',  ( 97.92893218813451028, 5.000000000000018652, 13.81250000000000000 ) ) ;
#1650=CARTESIAN_POINT ( 'NONE',  ( 104.9999999999999716, 1.449011120738813565E-14, 34.79898987322334136 ) ) ;
#1657=CARTESIAN_POINT ( 'NONE',  ( 99.99999999999995737, 5.000000000000018652, 6.875000002731185056 ) ) ;
#1672=CIRCLE ( 'NONE', #19864, 5.000000000000004441 ) ;
#1678=CARTESIAN_POINT ( 'NONE',  ( 99.99999999999995737, -4.458734124999988779, 11.68750000136559208 ) ) ;
#1706=CARTESIAN_POINT ( 'NONE',  ( 104.9999999999999574, 2.071067811865491937, 10.56249999999999822 ) ) ;
#1707=CARTESIAN_POINT ( 'NONE',  ( 103.5355339059327093, 3.535533905932755072, 1.624999999999999778 ) ) ;
#1718=CARTESIAN_POINT ( 'NONE',  ( 94.99999999999995737, -2.071067811865466624, 8.187500002731185944 ) ) ;
#1719=CARTESIAN_POINT ( 'NONE',  ( 95.54126587499995082, 1.846868145590750077, 3.625000001365592972 ) ) ;
#1721=CARTESIAN_POINT ( 'NONE',  ( 103.1528011352953342, 3.152801135295383084, 8.062500001365592084 ) ) ;
#1731=EDGE_LOOP ( 'NONE', ( #25793, #7572, #13083, #7304 ) ) ;
#1736=CARTESIAN_POINT ( 'NONE',  ( 95.54126587499996504, 1.387778780781445676E-14, 5.687500001365591196 ) ) ;
#1752=CARTESIAN_POINT ( 'NONE',  ( 104.4587341249999781, 1.846868145590750299, 6.000000001365591196 ) ) ;
#1754=CARTESIAN_POINT ( 'NONE',  ( 98.15313185440923860, 4.458734125000016313, 4.500000001365592084 ) ) ;
#1774=CARTESIAN_POINT ( 'NONE',  ( 104.9999999999999716, 1.449011120738813565E-14, 3.499999999999999556 ) ) ;
#1791=CARTESIAN_POINT ( 'NONE',  ( 94.99999999999997158, -2.071067811865486608, 6.062500000000000000 ) ) ;
#1798=CARTESIAN_POINT ( 'NONE',  ( 99.99999999999995737, 5.000000000000018652, 1.875000002731185056 ) ) ;
#1802=FACE_OUTER_BOUND ( 'NONE', #21363, .T. ) ;
#1815=CARTESIAN_POINT ( 'NONE',  ( 104.4587341249999639, 1.442382525525748735E-14, 10.93750000136559208 ) ) ;
#1817=DIRECTION ( 'NONE',  ( 0.000000000000000000, 0.000000000000000000, 1.000000000000000000 ) ) ;
#1845=CARTESIAN_POINT ( 'NONE',  ( 99.99999999999995737, 5.000000000000018652, 5.750000000000000000 ) ) ;
#1852=CARTESIAN_POINT ( 'NONE',  ( 94.99999999999995737, 1.387778780781445676E-14, 6.999999999999999112 ) ) ;
#1858=CARTESIAN_POINT ( 'NONE',  ( 96.46446609406721961, -3.535533905932727539, 8.250000002731185944 ) ) ;
#1859=CARTESIAN_POINT ( 'NONE',  ( 104.4587341249999781, -1.846868145590721655, 3.125000001365592528 ) ) ;
#1861=CARTESIAN_POINT ( 'NONE',  ( 104.4587341249999639, 1.442382525525748735E-14, 6.937500001365592972 ) ) ;
#1877=AXIS2_PLACEMENT_3D ( 'NONE', #27298, #24865, #9884 ) ;
#1878=CARTESIAN_POINT ( 'NONE',  ( 101.8468681455906903, -4.458734124999987891, 4.000000001365592084 ) ) ;
#1888=VECTOR ( 'NONE', #18464, 1000.000000000000000 ) ;
#1892=CARTESIAN_POINT ( 'NONE',  ( 103.1528011352953342, 3.152801135295383084, 13.31250000136559386 ) ) ;
#1893=CARTESIAN_POINT ( 'NONE',  ( 104.4587341249999781, -1.846868145590721655, 2.875000001365592084 ) ) ;
#1895=CARTESIAN_POINT ( 'NONE',  ( 95.54126587499996504, -1.846868145590724986, 4.750000001365592084 ) ) ;
#1924=CARTESIAN_POINT ( 'NONE',  ( 104.4587341249999781, -1.846868145590721655, 14.12500000136559208 ) ) ;
#1936=CARTESIAN_POINT ( 'NONE',  ( 104.9999999999999574, 2.071067811865491937, 0.6875000027311858330 ) ) ;
#1950=CARTESIAN_POINT ( 'NONE',  ( 99.99999999999995737, 4.458734125000016313, 10.18750000136559208 ) ) ;
#1954=CARTESIAN_POINT ( 'NONE',  ( 101.8468681455906903, -4.458734124999987891, 11.75000000136559208 ) ) ;
#1965=CARTESIAN_POINT ( 'NONE',  ( 99.99999999999995737, -4.999999999999990230, 11.37500000273118594 ) ) ;
#1977=CARTESIAN_POINT ( 'NONE',  ( 96.46446609406721961, 3.535533905932755072, 4.874999999999999112 ) ) ;
#1984=CARTESIAN_POINT ( 'NONE',  ( 104.9999999999999574, 2.071067811865511032, 4.687500002731188609 ) ) ;
#1987=( BOUNDED_CURVE ( )  B_SPLINE_CURVE ( 2, ( #10735, #19721, #207, #2488, #8892, #28142, #17582, #8609, #17297 ),
 .UNSPECIFIED., .F., .F. ) 
 B_SPLINE_CURVE_WITH_KNOTS ( ( 3, 2, 2, 2, 3 ),
 ( 0.1785714285714286031, 0.1875000000000000000, 0.1964285714285713969, 0.2053571428571428215, 0.2142857142857142183 ),
 .UNSPECIFIED. ) 
 CURVE ( )  GEOMETRIC_REPRESENTATION_ITEM ( )  RATIONAL_B_SPLINE_CURVE ( ( 0.9999999999999997780, 0.9238795325112869605, 1.000000000000000000, 0.9238795325112867385, 1.000000000000000000, 0.9238795325112867385, 1.000000000000000000, 0.9238795325112871826, 0.9999999999999995559 ) ) 
 REPRESENTATION_ITEM ( '' )  );
#1992=CARTESIAN_POINT ( 'NONE',  ( 103.1528011352953342, 3.152801135295383084, 3.312500001365592972 ) ) ;
#1994=CARTESIAN_POINT ( 'NONE',  ( 99.99999999999995737, -4.458734124999988779, 5.687500001365591196 ) ) ;
#2008=CARTESIAN_POINT ( 'NONE',  ( 96.84719886470459471, -3.152801135295355994, 1.812500001365591640 ) ) ;
#2023=CARTESIAN_POINT ( 'NONE',  ( 104.4587341249999781, 1.846868145590750299, 14.25000000136559208 ) ) ;
#2026=CARTESIAN_POINT ( 'NONE',  ( 104.4587341249999781, -1.846868145590721655, 3.875000001365592084 ) ) ;
#2031=CARTESIAN_POINT ( 'NONE',  ( 99.99999999999995737, 5.000000000000018652, 7.875000002731185056 ) ) ;
#2036=( BOUNDED_CURVE ( )  B_SPLINE_CURVE ( 2, ( #5619, #3892, #12554, #27420, #10283, #1347, #27561, #1212, #18447 ),
 .UNSPECIFIED., .F., .F. ) 
 B_SPLINE_CURVE_WITH_KNOTS ( ( 3, 2, 2, 2, 3 ),
 ( 0.7500000000000000000, 0.7589285714285713969, 0.7678571428571429047, 0.7767857142857143016, 0.7857142857142856984 ),
 .UNSPECIFIED. ) 
 CURVE ( )  GEOMETRIC_REPRESENTATION_ITEM ( )  RATIONAL_B_SPLINE_CURVE ( ( 1.000000000000000000, 0.9238795325112867385, 1.000000000000000000, 0.9238795325112867385, 1.000000000000000000, 0.9238795325112867385, 1.000000000000000000, 0.9238795325112867385, 1.000000000000000000 ) ) 
 REPRESENTATION_ITEM ( '' )  );
#2042=CARTESIAN_POINT ( 'NONE',  ( 99.99999999999995737, -4.999999999999990230, 7.375000002731185944 ) ) ;
#2059=CARTESIAN_POINT ( 'NONE',  ( 96.84719886470459471, 3.152801135295383084, 10.56250000136559208 ) ) ;
#2073=CARTESIAN_POINT ( 'NONE',  ( 99.99999999999995737, -4.999999999999990230, 3.375000002731184612 ) ) ;
#2078=CYLINDRICAL_SURFACE ( 'NONE', #4321, 5.000000000000004441 ) ;
#2085=CARTESIAN_POINT ( 'NONE',  ( 99.99999999999995737, 5.000000000000018652, 10.75000000000000000 ) ) ;
#2088=CARTESIAN_POINT ( 'NONE',  ( 95.54126587499995082, 1.846868145590750077, 8.375000001365592084 ) ) ;
#2092=CARTESIAN_POINT ( 'NONE',  ( 99.99999999999995737, -4.458734124999988779, 12.68750000136559208 ) ) ;
#2114=VECTOR ( 'NONE', #17418, 1000.000000000000000 ) ;
#2115=CARTESIAN_POINT ( 'NONE',  ( 94.99999999999995737, 2.071067811865491048, 6.937499999999999112 ) ) ;
#2134=CARTESIAN_POINT ( 'NONE',  ( 104.4587341249999639, 1.442382525525748735E-14, 1.937500001365591640 ) ) ;
#2140=CARTESIAN_POINT ( 'NONE',  ( 94.99999999999995737, 1.387778780781445676E-14, 14.56250000136559208 ) ) ;
#2149=ORIENTED_EDGE ( 'NONE', *, *, #10165, .T. ) ;
#2151=CARTESIAN_POINT ( 'NONE',  ( 104.4587341249999781, 1.846868145590750299, 3.250000001365592528 ) ) ;
#2152=ORIENTED_EDGE ( 'NONE', *, *, #26598, .F. ) ;
#2165=CARTESIAN_POINT ( 'NONE',  ( 104.4587341249999639, 1.442382525525748735E-14, 1.937500001365591640 ) ) ;
#2168=CARTESIAN_POINT ( 'NONE',  ( 99.99999999999995737, -4.458734124999988779, 13.68750000136559208 ) ) ;
#2170=CARTESIAN_POINT ( 'NONE',  ( 98.15313185440923860, -4.458734124999987891, 0.8750000013655925279 ) ) ;
#2181=EDGE_CURVE ( 'NONE', #162, #7211, #22258, .T. ) ;
#2187=CARTESIAN_POINT ( 'NONE',  ( 104.4587341249999781, 1.846868145590750299, 14.25000000136559208 ) ) ;
#2199=VERTEX_POINT ( 'NONE', #7127 ) ;
#2203=CARTESIAN_POINT ( 'NONE',  ( 96.84719886470459471, -3.152801135295355994, 10.81250000136559208 ) ) ;
#2218=CARTESIAN_POINT ( 'NONE',  ( 94.99999999999995737, 2.071067811865491048, 3.062500002731186388 ) ) ;
#2224=SURFACE_SIDE_STYLE ('',( #24019 ) ) ;
#2236=CARTESIAN_POINT ( 'NONE',  ( 95.54126587499995082, -1.846868145590724986, 7.500000001365592084 ) ) ;
#2239=CARTESIAN_POINT ( 'NONE',  ( 101.8468681455906903, 4.458734125000016313, 11.12500000136559386 ) ) ;
#2253=ORIENTED_EDGE ( 'NONE', *, *, #27597, .F. ) ;
#2264=CARTESIAN_POINT ( 'NONE',  ( 97.92893218813451028, -4.999999999999989342, 6.187499999999999112 ) ) ;
#2297=CARTESIAN_POINT ( 'NONE',  ( 96.84719886470459471, 3.152801135295383084, 2.562500001365592084 ) ) ;
#2312=CARTESIAN_POINT ( 'NONE',  ( 99.99999999999995737, 4.458734125000016313, 11.43750000136559208 ) ) ;
#2314=CARTESIAN_POINT ( 'NONE',  ( 103.1528011352953342, -3.152801135295355106, 12.81250000136559208 ) ) ;
#2327=ORIENTED_EDGE ( 'NONE', *, *, #10555, .T. ) ;
#2341=EDGE_LOOP ( 'NONE', ( #8716, #25264, #2913, #16596 ) ) ;
#2347=CARTESIAN_POINT ( 'NONE',  ( 104.4587341249999639, 1.442382525525748735E-14, 11.18750000136559208 ) ) ;
#2357=VERTEX_POINT ( 'NONE', #1173 ) ;
#2360=CARTESIAN_POINT ( 'NONE',  ( 97.92893218813451028, 5.000000000000018652, 2.937500002731185944 ) ) ;
#2377=CARTESIAN_POINT ( 'NONE',  ( 95.54126587499996504, 1.387778780781445676E-14, 8.437500001365592084 ) ) ;
#2378=ORIENTED_EDGE ( 'NONE', *, *, #5307, .F. ) ;
#2380=CARTESIAN_POINT ( 'NONE',  ( 103.1528011352953342, -3.152801135295355106, 13.81250000136559208 ) ) ;
#2395=CARTESIAN_POINT ( 'NONE',  ( 95.54126587499996504, 1.387778780781445676E-14, 0.4375000013655920839 ) ) ;
#2403=CARTESIAN_POINT ( 'NONE',  ( 94.99999999999995737, 1.387778780781445676E-14, 1.999999999999998224 ) ) ;
#2422=CARTESIAN_POINT ( 'NONE',  ( 104.4587341249999781, -1.846868145590721655, 1.875000001365591862 ) ) ;
#2424=CARTESIAN_POINT ( 'NONE',  ( 94.99999999999995737, 1.387778780781445676E-14, 4.999999999999999112 ) ) ;
#2432=MECHANICAL_DESIGN_GEOMETRIC_PRESENTATION_REPRESENTATION('',(#17879),#7891);
#2437=CARTESIAN_POINT ( 'NONE',  ( 95.54126587499995082, 1.846868145590750077, 2.625000001365592084 ) ) ;
#2449=CARTESIAN_POINT ( 'NONE',  ( 99.99999999999995737, -4.458734124999988779, 12.93750000136559208 ) ) ;
#2451=CARTESIAN_POINT ( 'NONE',  ( 101.8468681455907046, -4.458734124999987891, 13.75000000136559208 ) ) ;
#2464=CARTESIAN_POINT ( 'NONE',  ( 104.9999999999999716, -2.071067811865452857, 7.562500002731185944 ) ) ;
#2466=CARTESIAN_POINT ( 'NONE',  ( 98.15313185440925281, 4.458734125000016313, 13.50000000136559208 ) ) ;
#2481=CARTESIAN_POINT ( 'NONE',  ( 104.4587341249999639, 1.442382525525748735E-14, 9.187500001365592084 ) ) ;
#2488=CARTESIAN_POINT ( 'NONE',  ( 102.0710678118654329, -4.999999999999989342, 12.31249999999999822 ) ) ;
#2509=AXIS2_PLACEMENT_3D ( 'NONE', #4496, #13154, #21892 ) ;
#2510=ORIENTED_EDGE ( 'NONE', *, *, #19041, .T. ) ;
#2511=CARTESIAN_POINT ( 'NONE',  ( 104.4587341249999639, 1.442382525525748735E-14, 7.937500001365592084 ) ) ;
#2514=CARTESIAN_POINT ( 'NONE',  ( 98.15313185440925281, -4.458734124999987891, 11.62500000136559031 ) ) ;
#2527=VERTEX_POINT ( 'NONE', #6195 ) ;
#2532=CARTESIAN_POINT ( 'NONE',  ( 99.99999999999995737, -4.999999999999990230, 9.375000002731184168 ) ) ;
#2538=( BOUNDED_CURVE ( )  B_SPLINE_CURVE ( 2, ( #25619, #18520, #9945, #23352, #12629, #3692, #3969, #25347, #14361 ),
 .UNSPECIFIED., .F., .F. ) 
 B_SPLINE_CURVE_WITH_KNOTS ( ( 3, 2, 2, 2, 3 ),
 ( 0.4999999999999998890, 0.5089285714285712858, 0.5178571428571427937, 0.5267857142857143016, 0.5357142857142856984 ),
 .UNSPECIFIED. ) 
 CURVE ( )  GEOMETRIC_REPRESENTATION_ITEM ( )  RATIONAL_B_SPLINE_CURVE ( ( 1.000000000000000888, 0.9238795325112857393, 1.000000000000000000, 0.9238795325112867385, 1.000000000000000000, 0.9238795325112867385, 1.000000000000000000, 0.9238795325112867385, 1.000000000000000000 ) ) 
 REPRESENTATION_ITEM ( '' )  );
#2560=CARTESIAN_POINT ( 'NONE',  ( 104.4587341249999781, -1.846868145590721655, 3.875000001365591640 ) ) ;
#2580=CARTESIAN_POINT ( 'NONE',  ( 99.99999999999995737, 5.000000000000018652, 13.75000000000000000 ) ) ;
#2593=CARTESIAN_POINT ( 'NONE',  ( 95.54126587499996504, 1.387778780781445676E-14, 12.68750000136559208 ) ) ;
#2595=CARTESIAN_POINT ( 'NONE',  ( 99.99999999999995737, 4.458734125000016313, 12.18750000136559208 ) ) ;
#2609=CARTESIAN_POINT ( 'NONE',  ( 99.99999999999995737, 4.458734125000016313, 11.43750000136559208 ) ) ;
#2627=CARTESIAN_POINT ( 'NONE',  ( 104.4587341249999781, 1.846868145590750521, 12.25000000136559208 ) ) ;
#2650=LINE ( 'NONE', #24876, #1888 ) ;
#2652=PRODUCT_DEFINITION ( 'UNKNOWN', '', #23155, #1521 ) ;
#2655=CARTESIAN_POINT ( 'NONE',  ( 104.4587341249999781, -1.846868145590721655, 3.875000001365592084 ) ) ;
#2658=CARTESIAN_POINT ( 'NONE',  ( 104.4587341249999639, 1.442382525525748735E-14, 6.937500001365592972 ) ) ;
#2669=CARTESIAN_POINT ( 'NONE',  ( 104.9999999999999716, 1.449011120738813565E-14, 7.500000000000000000 ) ) ;
#2676=CARTESIAN_POINT ( 'NONE',  ( 97.92893218813451028, -4.999999999999989342, 11.31250000273118594 ) ) ;
#2682=CARTESIAN_POINT ( 'NONE',  ( 104.9999999999999574, -2.071067811865462627, 2.437499999999998668 ) ) ;
#2690=DIRECTION ( 'NONE',  ( -0.000000000000000000, -0.000000000000000000, -1.000000000000000000 ) ) ;
#2691=CARTESIAN_POINT ( 'NONE',  ( 96.46446609406721961, 3.535533905932755072, 12.87500000000000000 ) ) ;
#2699=CARTESIAN_POINT ( 'NONE',  ( 99.99999999999995737, -4.999999999999990230, 4.375000002731185056 ) ) ;
#2703=CARTESIAN_POINT ( 'NONE',  ( 95.54126587499996504, 1.846868145590750077, 3.375000001365592972 ) ) ;
#2705=ORIENTED_EDGE ( 'NONE', *, *, #2887, .F. ) ;
#2709=ORIENTED_EDGE ( 'NONE', *, *, #23068, .F. ) ;
#2721=CARTESIAN_POINT ( 'NONE',  ( 94.99999999999995737, 2.071067811865491048, 13.93749999999999822 ) ) ;
#2732=CARTESIAN_POINT ( 'NONE',  ( 96.84719886470459471, 3.152801135295383084, 11.56250000136559208 ) ) ;
#2733=DIRECTION ( 'NONE',  ( -0.000000000000000000, -0.000000000000000000, -1.000000000000000000 ) ) ;
#2734=CARTESIAN_POINT ( 'NONE',  ( 98.15313185440925281, -4.458734124999987891, 0.6250000013655921949 ) ) ;
#2737=CYLINDRICAL_SURFACE ( 'NONE', #5278, 5.000000000000004441 ) ;
#2745=CARTESIAN_POINT ( 'NONE',  ( 94.99999999999995737, 1.387778780781445676E-14, 4.125000002731185056 ) ) ;
#2746=CARTESIAN_POINT ( 'NONE',  ( 99.99999999999995737, -4.999999999999990230, 1.249999999999999334 ) ) ;
#2750=CARTESIAN_POINT ( 'NONE',  ( 96.84719886470459471, -3.152801135295355994, 11.81250000136559208 ) ) ;
#2752=EDGE_LOOP ( 'NONE', ( #12074, #21349, #19696, #18924 ) ) ;
#2767=CARTESIAN_POINT ( 'NONE',  ( 103.1528011352953342, -3.152801135295355106, 7.062500001365592972 ) ) ;
#2786=CARTESIAN_POINT ( 'NONE',  ( 104.9999999999999858, -2.071067811865442643, 1.562500002731185722 ) ) ;
#2792=CARTESIAN_POINT ( 'NONE',  ( 96.84719886470459471, 3.152801135295383084, 6.312500001365592084 ) ) ;
#2795=CARTESIAN_POINT ( 'NONE',  ( 95.54126587499995082, 1.846868145590750077, 8.375000001365592084 ) ) ;
#2803=LINE ( 'NONE', #528, #6630 ) ;
#2805=DIRECTION ( 'NONE',  ( 0.000000000000000000, 0.000000000000000000, 1.000000000000000000 ) ) ;
#2811=CARTESIAN_POINT ( 'NONE',  ( 104.9999999999999716, 1.449011120738813565E-14, 10.62500000273118594 ) ) ;
#2814=EDGE_CURVE ( 'NONE', #3701, #16509, #21793, .T. ) ;
#2817=CARTESIAN_POINT ( 'NONE',  ( 94.99999999999995737, -2.071067811865466624, 2.062499999999998668 ) ) ;
#2853=CARTESIAN_POINT ( 'NONE',  ( 94.99999999999995737, 2.071067811865491048, 14.93750000000000000 ) ) ;
#2865=CARTESIAN_POINT ( 'NONE',  ( 104.4587341249999639, 1.442382525525748735E-14, 8.187500001365592084 ) ) ;
#2867=CARTESIAN_POINT ( 'NONE',  ( 103.1528011352953342, -3.152801135295355106, 9.812500001365593860 ) ) ;
#2873=COLOUR_RGB ( '', 0.09019608, 0.27058824, 0.51372549) ;
#2879=VERTEX_POINT ( 'NONE', #4910 ) ;
#2880=EDGE_CURVE ( 'NONE', #5815, #6644, #16145, .T. ) ;
#2882=CARTESIAN_POINT ( 'NONE',  ( 101.8468681455906903, -4.458734124999987891, 11.00000000136559208 ) ) ;
#2887=EDGE_CURVE ( 'NONE', #2527, #9281, #14118, .T. ) ;
#2900=CARTESIAN_POINT ( 'NONE',  ( 103.1528011352953342, -3.152801135295355106, 9.062500001365592084 ) ) ;
#2904=CARTESIAN_POINT ( 'NONE',  ( 96.46446609406721961, -3.535533905932727539, 14.12499999999999822 ) ) ;
#2913=ORIENTED_EDGE ( 'NONE', *, *, #11909, .T. ) ;
#2918=CARTESIAN_POINT ( 'NONE',  ( 103.5355339059327093, 3.535533905932755072, 10.75000000273118594 ) ) ;
#2927=CARTESIAN_POINT ( 'NONE',  ( 96.84719886470459471, -3.152801135295355994, 6.562500001365592084 ) ) ;
#2929=CARTESIAN_POINT ( 'NONE',  ( 99.99999999999995737, 5.000000000000018652, 12.87500000273118594 ) ) ;
#2930=CARTESIAN_POINT ( 'NONE',  ( 96.84719886470459471, 3.152801135295383084, 7.312500001365592084 ) ) ;
#2937=VECTOR ( 'NONE', #3164, 1000.000000000000000 ) ;
#2947=CARTESIAN_POINT ( 'NONE',  ( 104.9999999999999574, -2.071067811865462627, 10.56250000273118594 ) ) ;
#2953=CARTESIAN_POINT ( 'NONE',  ( 102.0710678118654329, 5.000000000000018652, 2.687499999999999112 ) ) ;
#2960=CARTESIAN_POINT ( 'NONE',  ( 103.5355339059327093, -3.535533905932726206, 10.50000000273118594 ) ) ;
#2961=CARTESIAN_POINT ( 'NONE',  ( 97.92893218813451028, 5.000000000000018652, 12.81250000000000000 ) ) ;
#2968=CARTESIAN_POINT ( 'NONE',  ( 103.5355339059327093, -3.535533905932726206, 4.500000002731185944 ) ) ;
#2993=CARTESIAN_POINT ( 'NONE',  ( 102.0710678118654329, 5.000000000000018652, 14.68749999999999822 ) ) ;
#3007=CARTESIAN_POINT ( 'NONE',  ( 103.1528011352953342, 3.152801135295383084, 5.312500001365592972 ) ) ;
#3010=CARTESIAN_POINT ( 'NONE',  ( 98.15313185440923860, 4.458734125000016313, 8.250000001365592084 ) ) ;
#3025=CARTESIAN_POINT ( 'NONE',  ( 99.99999999999995737, 4.458734125000016313, 9.437500001365593860 ) ) ;
#3029=VECTOR ( 'NONE', #12708, 1000.000000000000000 ) ;
#3035=EDGE_CURVE ( 'NONE', #2357, #22244, #23661, .T. ) ;
#3042=CARTESIAN_POINT ( 'NONE',  ( 99.99999999999995737, -4.458734124999988779, 8.937500001365592084 ) ) ;
#3061=CARTESIAN_POINT ( 'NONE',  ( 99.99999999999995737, -4.999999999999990230, 0.3750000027311853890 ) ) ;
#3078=CARTESIAN_POINT ( 'NONE',  ( 95.54126587499996504, 1.387778780781445676E-14, 6.437500001365592084 ) ) ;
#3081=CARTESIAN_POINT ( 'NONE',  ( 96.84719886470459471, 3.152801135295383084, 9.312500001365593860 ) ) ;
#3097=CARTESIAN_POINT ( 'NONE',  ( 96.46446609406721961, -3.535533905932727539, 10.25000000273118594 ) ) ;
#3101=CARTESIAN_POINT ( 'NONE',  ( 94.99999999999995737, 2.071067811865491493, 14.93749999999999822 ) ) ;
#3111=CARTESIAN_POINT ( 'NONE',  ( 94.99999999999995737, 1.387778780781445676E-14, 10.12500000273118594 ) ) ;
#3113=CARTESIAN_POINT ( 'NONE',  ( 94.99999999999995737, 2.071067811865491493, 12.93750000000000000 ) ) ;
#3125=CARTESIAN_POINT ( 'NONE',  ( 95.27063293749995410, 1.387778780781445676E-14, 14.84375000068279604 ) ) ;
#3132=VERTEX_POINT ( 'NONE', #15259 ) ;
#3140=AXIS2_PLACEMENT_3D ( 'NONE', #24486, #843, #9516 ) ;
#3144=CARTESIAN_POINT ( 'NONE',  ( 94.99999999999995737, 1.387778780781445676E-14, 12.00000000000000000 ) ) ;
#3150=CARTESIAN_POINT ( 'NONE',  ( 97.92893218813451028, 5.000000000000018652, 0.9375000027311859441 ) ) ;
#3155=CARTESIAN_POINT ( 'NONE',  ( 104.4587341249999639, 1.442382525525748735E-14, 6.187500001365592084 ) ) ;
#3157=CARTESIAN_POINT ( 'NONE',  ( 95.54126587499996504, 1.846868145590750077, 11.37500000136559208 ) ) ;
#3164=DIRECTION ( 'NONE',  ( -0.000000000000000000, -0.000000000000000000, -1.000000000000000000 ) ) ;
#3168=CARTESIAN_POINT ( 'NONE',  ( 104.9999999999999716, 1.449011120738813565E-14, 34.79898987322334136 ) ) ;
#3169=CARTESIAN_POINT ( 'NONE',  ( 104.4587341249999639, 1.442382525525748735E-14, 11.18750000136559208 ) ) ;
#3186=CARTESIAN_POINT ( 'NONE',  ( 99.99999999999995737, -4.458734124999988779, 5.937500001365592084 ) ) ;
#3204=CARTESIAN_POINT ( 'NONE',  ( 102.0710678118654329, -4.999999999999989342, 13.31250000000000000 ) ) ;
#3216=CARTESIAN_POINT ( 'NONE',  ( 99.99999999999995737, -4.458734124999988779, 3.687500001365591640 ) ) ;
#3217=EDGE_LOOP ( 'NONE', ( #4056, #18192, #15839, #9906 ) ) ;
#3218=CARTESIAN_POINT ( 'NONE',  ( 99.99999999999995737, 4.458734125000016313, 5.187500001365592972 ) ) ;
#3235=CARTESIAN_POINT ( 'NONE',  ( 99.99999999999995737, 5.000000000000018652, 5.875000002731185056 ) ) ;
#3281=CARTESIAN_POINT ( 'NONE',  ( 96.46446609406721961, -3.535533905932727539, 9.125000000000000000 ) ) ;
#3287=CARTESIAN_POINT ( 'NONE',  ( 102.0710678118654329, 5.000000000000018652, 11.81250000273118772 ) ) ;
#3290=( BOUNDED_CURVE ( )  B_SPLINE_CURVE ( 2, ( #3682, #23478, #5684, #3393, #8358, #12346, #25607, #3958, #14350 ),
 .UNSPECIFIED., .F., .F. ) 
 B_SPLINE_CURVE_WITH_KNOTS ( ( 3, 2, 2, 2, 3 ),
 ( 0.8571428571428570953, 0.8660714285714286031, 0.8750000000000000000, 0.8839285714285712858, 0.8928571428571427937 ),
 .UNSPECIFIED. ) 
 CURVE ( )  GEOMETRIC_REPRESENTATION_ITEM ( )  RATIONAL_B_SPLINE_CURVE ( ( 1.000000000000000000, 0.9238795325112867385, 1.000000000000000000, 0.9238795325112867385, 1.000000000000000000, 0.9238795325112867385, 1.000000000000000000, 0.9238795325112877377, 0.9999999999999990008 ) ) 
 REPRESENTATION_ITEM ( '' )  );
#3291=CARTESIAN_POINT ( 'NONE',  ( 94.99999999999995737, 1.387778780781445676E-14, 12.12500000273118594 ) ) ;
#3296=CARTESIAN_POINT ( 'NONE',  ( 98.15313185440925281, -4.458734124999987891, 6.875000001365592972 ) ) ;
#3298=CARTESIAN_POINT ( 'NONE',  ( 96.84719886470459471, -3.152801135295355994, 8.562500001365592084 ) ) ;
#3301=CARTESIAN_POINT ( 'NONE',  ( 94.99999999999995737, 1.387778780781445676E-14, 9.000000000000000000 ) ) ;
#3304=ORIENTED_EDGE ( 'NONE', *, *, #1152, .T. ) ;
#3311=CARTESIAN_POINT ( 'NONE',  ( 101.8468681455906903, -4.458734124999987891, 6.000000001365591196 ) ) ;
#3324=CARTESIAN_POINT ( 'NONE',  ( 103.1528011352953342, -3.152801135295355106, 6.062500001365592084 ) ) ;
#3347=CARTESIAN_POINT ( 'NONE',  ( 94.99999999999995737, 1.387778780781445676E-14, 5.125000002731184168 ) ) ;
#3353=CARTESIAN_POINT ( 'NONE',  ( 96.84719886470459471, 3.152801135295383084, 13.56250000136559386 ) ) ;
#3368=CARTESIAN_POINT ( 'NONE',  ( 102.0710678118654329, 5.000000000000018652, 3.812500002731184612 ) ) ;
#3385=CARTESIAN_POINT ( 'NONE',  ( 103.1528011352953342, 3.152801135295383084, 14.06250000136559208 ) ) ;
#3393=CARTESIAN_POINT ( 'NONE',  ( 97.92893218813451028, 5.000000000000018652, 2.812499999999999112 ) ) ;
#3415=ORIENTED_EDGE ( 'NONE', *, *, #18830, .F. ) ;
#3416=CARTESIAN_POINT ( 'NONE',  ( 104.9999999999999716, 1.449011120738813565E-14, 9.500000000000000000 ) ) ;
#3422=CARTESIAN_POINT ( 'NONE',  ( 104.9999999999999574, -2.071067811865462627, 12.56250000273118772 ) ) ;
#3431=CARTESIAN_POINT ( 'NONE',  ( 99.99999999999995737, -4.458734124999988779, 7.937500001365592084 ) ) ;
#3434=CARTESIAN_POINT ( 'NONE',  ( 99.99999999999995737, -4.458734124999988779, 9.687500001365593860 ) ) ;
#3443=EDGE_CURVE ( 'NONE', #7689, #10159, #21963, .T. ) ;
#3450=CARTESIAN_POINT ( 'NONE',  ( 95.54126587499995082, 1.846868145590750077, 7.625000001365592084 ) ) ;
#3464=CARTESIAN_POINT ( 'NONE',  ( 99.99999999999995737, 4.458734125000016313, 4.437500001365592084 ) ) ;
#3478=VECTOR ( 'NONE', #14868, 1000.000000000000000 ) ;
#3491=CARTESIAN_POINT ( 'NONE',  ( 94.99999999999995737, -2.071067811865466624, 7.062499999999999112 ) ) ;
#3496=CARTESIAN_POINT ( 'NONE',  ( 104.4587341249999639, 1.442382525525748735E-14, 14.18750000136559208 ) ) ;
#3506=CARTESIAN_POINT ( 'NONE',  ( 104.9999999999999716, -2.071067811865462627, 6.437499999999999112 ) ) ;
#3516=CARTESIAN_POINT ( 'NONE',  ( 104.9999999999999716, 1.449011120738813565E-14, 4.625000002731185944 ) ) ;
#3536=CARTESIAN_POINT ( 'NONE',  ( 104.4587341249999639, 1.442382525525748735E-14, 13.93750000136559208 ) ) ;
#3537=CARTESIAN_POINT ( 'NONE',  ( 104.9999999999999716, 1.449011120738813565E-14, 13.62500000273118417 ) ) ;
#3538=ORIENTED_EDGE ( 'NONE', *, *, #9856, .T. ) ;
#3561=CARTESIAN_POINT ( 'NONE',  ( 102.0710678118654329, -4.999999999999989342, 8.312500000000000000 ) ) ;
#3562=EDGE_LOOP ( 'NONE', ( #1507, #10424, #14446, #1359, #25329 ) ) ;
#3567=CARTESIAN_POINT ( 'NONE',  ( 94.99999999999995737, 2.071067811865491048, 13.06250000273118772 ) ) ;
#3570=EDGE_CURVE ( 'NONE', #15231, #896, #20412, .T. ) ;
#3571=CARTESIAN_POINT ( 'NONE',  ( 104.9999999999999716, 1.449011120738813565E-14, 11.50000000000000000 ) ) ;
#3577=CARTESIAN_POINT ( 'NONE',  ( 99.99999999999995737, 4.458734125000016313, 3.437500001365592972 ) ) ;
#3579=CARTESIAN_POINT ( 'NONE',  ( 103.1528011352953342, -3.152801135295355106, 5.812500001365591196 ) ) ;
#3594=CARTESIAN_POINT ( 'NONE',  ( 99.99999999999995737, 4.458734125000016313, 7.437500001365592084 ) ) ;
#3610=CARTESIAN_POINT ( 'NONE',  ( 103.1528011352953342, 3.152801135295383084, 3.312500001365592972 ) ) ;
#3647=LINE ( 'NONE', #25859, #24405 ) ;
#3658=CARTESIAN_POINT ( 'NONE',  ( 94.99999999999995737, 1.387778780781445676E-14, 7.125000002731185056 ) ) ;
#3661=ORIENTED_EDGE ( 'NONE', *, *, #2880, .F. ) ;
#3676=CARTESIAN_POINT ( 'NONE',  ( 104.4587341249999781, -1.846868145590721655, 11.87500000136559031 ) ) ;
#3680=CARTESIAN_POINT ( 'NONE',  ( 96.46446609406721961, 3.535533905932755072, 8.875000000000000000 ) ) ;
#3682=CARTESIAN_POINT ( 'NONE',  ( 94.99999999999995737, 1.387778780781445676E-14, 2.999999999999999112 ) ) ;
#3692=CARTESIAN_POINT ( 'NONE',  ( 102.0710678118654329, 5.000000000000018652, 7.687499999999999112 ) ) ;
#3701=VERTEX_POINT ( 'NONE', #24965 ) ;
#3702=CARTESIAN_POINT ( 'NONE',  ( 94.99999999999995737, -2.071067811865466624, 11.06250000000000000 ) ) ;
#3704=( BOUNDED_CURVE ( )  B_SPLINE_CURVE ( 2, ( #19039, #23469, #14888, #21901, #10756, #22033, #10896, #15456, #23746 ),
 .UNSPECIFIED., .F., .F. ) 
 B_SPLINE_CURVE_WITH_KNOTS ( ( 3, 2, 2, 2, 3 ),
 ( 0.3214285714285713969, 0.3303571428571427937, 0.3392857142857143016, 0.3482142857142856984, 0.3571428571428572063 ),
 .UNSPECIFIED. ) 
 CURVE ( )  GEOMETRIC_REPRESENTATION_ITEM ( )  RATIONAL_B_SPLINE_CURVE ( ( 1.000000000000000444, 0.9238795325112862944, 1.000000000000000000, 0.9238795325112867385, 1.000000000000000000, 0.9238795325112867385, 1.000000000000000000, 0.9238795325112862944, 1.000000000000000444 ) ) 
 REPRESENTATION_ITEM ( '' )  );
#3717=CARTESIAN_POINT ( 'NONE',  ( 104.4587341249999781, 1.846868145590750299, 1.250000001365592750 ) ) ;
#3719=CARTESIAN_POINT ( 'NONE',  ( 99.99999999999995737, -4.458734124999988779, 4.687500001365592084 ) ) ;
#3723=CARTESIAN_POINT ( 'NONE',  ( 99.99999999999995737, 1.387778780781445676E-14, 34.79898987322334136 ) ) ;
#3732=CARTESIAN_POINT ( 'NONE',  ( 99.99999999999995737, -4.458734124999988779, 4.937500001365592972 ) ) ;
#3746=CARTESIAN_POINT ( 'NONE',  ( 98.15313185440925281, 4.458734125000016313, 2.250000001365591640 ) ) ;
#3748=CARTESIAN_POINT ( 'NONE',  ( 95.54126587499996504, 1.846868145590750077, 3.625000001365592528 ) ) ;
#3761=DIRECTION ( 'NONE',  ( 0.000000000000000000, 0.000000000000000000, 1.000000000000000000 ) ) ;
#3769=DIRECTION ( 'NONE',  ( -0.000000000000000000, -0.000000000000000000, -1.000000000000000000 ) ) ;
#3778=CARTESIAN_POINT ( 'NONE',  ( 98.15313185440923860, 4.458734125000016313, 13.50000000136559386 ) ) ;
#3791=CARTESIAN_POINT ( 'NONE',  ( 94.99999999999995737, 1.387778780781445676E-14, 4.125000002731185056 ) ) ;
#3807=DIRECTION ( 'NONE',  ( -0.000000000000000000, -0.000000000000000000, -1.000000000000000000 ) ) ;
#3808=CARTESIAN_POINT ( 'NONE',  ( 99.99999999999995737, 4.458734125000016313, 14.18750000136559208 ) ) ;
#3833=CARTESIAN_POINT ( 'NONE',  ( 103.5355339059327093, -3.535533905932726206, 8.375000000000000000 ) ) ;
#3847=CARTESIAN_POINT ( 'NONE',  ( 104.9999999999999716, -2.071067811865462627, 8.562500002731185944 ) ) ;
#3848=CARTESIAN_POINT ( 'NONE',  ( 104.4587341249999781, -1.846868145590721655, 1.125000001365592750 ) ) ;
#3850=CARTESIAN_POINT ( 'NONE',  ( 95.54126587499996504, 1.387778780781445676E-14, 7.437500001365592084 ) ) ;
#3856=ORIENTED_EDGE ( 'NONE', *, *, #7501, .T. ) ;
#3865=CARTESIAN_POINT ( 'NONE',  ( 99.99999999999995737, 4.458734125000016313, 6.437500001365592084 ) ) ;
#3881=CARTESIAN_POINT ( 'NONE',  ( 99.99999999999995737, -4.458734124999988779, 5.687500001365591196 ) ) ;
#3883=CARTESIAN_POINT ( 'NONE',  ( 98.15313185440923860, -4.458734124999987891, 1.875000001365591862 ) ) ;
#3892=CARTESIAN_POINT ( 'NONE',  ( 104.9999999999999716, -2.071067811865462627, 3.562500002731184612 ) ) ;
#3894=CIRCLE ( 'NONE', #23465, 7.000000000000006217 ) ;
#3896=VERTEX_POINT ( 'NONE', #19241 ) ;
#3916=SURFACE_STYLE_FILL_AREA ( #25572 ) ;
#3917=LINE ( 'NONE', #1643, #8440 ) ;
#3920=CARTESIAN_POINT ( 'NONE',  ( 103.5355339059327093, 3.535533905932755072, 13.62500000000000000 ) ) ;
#3922=CARTESIAN_POINT ( 'NONE',  ( 94.99999999999995737, 1.387778780781445676E-14, 34.79898987322334136 ) ) ;
#3925=CARTESIAN_POINT ( 'NONE',  ( 104.9999999999999716, 1.449011120738813565E-14, 6.499999999999999112 ) ) ;
#3932=CARTESIAN_POINT ( 'NONE',  ( 97.92893218813451028, -4.999999999999989342, 3.312500002731184612 ) ) ;
#3950=CARTESIAN_POINT ( 'NONE',  ( 101.8468681455906903, 4.458734125000016313, 14.12500000136559208 ) ) ;
#3958=CARTESIAN_POINT ( 'NONE',  ( 104.9999999999999574, 2.071067811865511032, 2.562499999999999556 ) ) ;
#3964=LINE ( 'NONE', #14903, #24861 ) ;
#3969=CARTESIAN_POINT ( 'NONE',  ( 103.5355339059327093, 3.535533905932755072, 7.624999999999999112 ) ) ;
#3977=CARTESIAN_POINT ( 'NONE',  ( 97.92893218813451028, 5.000000000000018652, 6.812499999999999112 ) ) ;
#3990=SHAPE_DEFINITION_REPRESENTATION ( #8986, #17883 ) ;
#3991=CARTESIAN_POINT ( 'NONE',  ( 104.9999999999999716, 1.449011120738813565E-14, 8.625000002731185944 ) ) ;
#3992=CARTESIAN_POINT ( 'NONE',  ( 95.54126587499995082, -1.846868145590724986, 3.750000001365591640 ) ) ;
#3994=CARTESIAN_POINT ( 'NONE',  ( 96.84719886470459471, 3.152801135295383084, 4.312500001365592084 ) ) ;
#4008=CARTESIAN_POINT ( 'NONE',  ( 98.15313185440925281, 4.458734125000016313, 3.500000001365592528 ) ) ;
#4022=CARTESIAN_POINT ( 'NONE',  ( 104.4587341249999781, -1.846868145590721655, 0.8750000013655926390 ) ) ;
#4024=CARTESIAN_POINT ( 'NONE',  ( 98.15313185440925281, 4.458734125000016313, 3.250000001365592528 ) ) ;
#4027=CARTESIAN_POINT ( 'NONE',  ( 95.54126587499996504, 1.387778780781445676E-14, 4.687500001365592084 ) ) ;
#4035=CARTESIAN_POINT ( 'NONE',  ( 102.0710678118654329, 5.000000000000018652, 5.687500000000000000 ) ) ;
#4045=CARTESIAN_POINT ( 'NONE',  ( 94.99999999999995737, 1.387778780781445676E-14, 34.79898987322334136 ) ) ;
#4056=ORIENTED_EDGE ( 'NONE', *, *, #1334, .T. ) ;
#4058=CARTESIAN_POINT ( 'NONE',  ( 95.54126587499996504, 1.387778780781445676E-14, 14.68750000136559208 ) ) ;
#4069=ORIENTED_EDGE ( 'NONE', *, *, #16974, .F. ) ;
#4072=CARTESIAN_POINT ( 'NONE',  ( 103.5355339059327093, -3.535533905932726206, 1.500000002731184612 ) ) ;
#4079=DIRECTION ( 'NONE',  ( -1.000000000000000000, 0.000000000000000000, 0.000000000000000000 ) ) ;
#4087=CARTESIAN_POINT ( 'NONE',  ( 101.8468681455906903, -4.458734124999987891, 8.750000001365592084 ) ) ;
#4090=CARTESIAN_POINT ( 'NONE',  ( 95.54126587499996504, 1.387778780781445676E-14, 10.43750000136559208 ) ) ;
#4093=AXIS2_PLACEMENT_3D ( 'NONE', #23003, #8022, #18584 ) ;
#4114=CARTESIAN_POINT ( 'NONE',  ( 99.99999999999995737, 5.000000000000018652, 3.750000000000000000 ) ) ;
#4128=CARTESIAN_POINT ( 'NONE',  ( 96.84719886470459471, -3.152801135295355994, 3.812500001365591640 ) ) ;
#4131=CARTESIAN_POINT ( 'NONE',  ( 104.4587341249999781, -1.846868145590721655, 5.875000001365592084 ) ) ;
#4134=CYLINDRICAL_SURFACE ( 'NONE', #9349, 5.000000000000004441 ) ;
#4149=CARTESIAN_POINT ( 'NONE',  ( 101.8468681455906903, 4.458734125000016313, 2.375000001365592084 ) ) ;
#4150=ORIENTED_EDGE ( 'NONE', *, *, #23532, .T. ) ;
#4162=CARTESIAN_POINT ( 'NONE',  ( 97.92893218813451028, 5.000000000000018652, 9.812499999999998224 ) ) ;
#4163=CARTESIAN_POINT ( 'NONE',  ( 101.8468681455906903, -4.458734124999987891, 2.750000001365592084 ) ) ;
#4165=CARTESIAN_POINT ( 'NONE',  ( 98.15313185440925281, -4.458734124999987891, 5.625000001365591196 ) ) ;
#4193=ORIENTED_EDGE ( 'NONE', *, *, #10447, .F. ) ;
#4207=CARTESIAN_POINT ( 'NONE',  ( 96.46446609406721961, 3.535533905932755072, 3.000000002731185944 ) ) ;
#4223=CARTESIAN_POINT ( 'NONE',  ( 96.84719886470459471, 3.152801135295383084, 7.312500001365592084 ) ) ;
#4227=CARTESIAN_POINT ( 'NONE',  ( 96.84719886470459471, 3.152801135295383084, 13.31250000136559386 ) ) ;
#4237=CARTESIAN_POINT ( 'NONE',  ( 97.92893218813451028, -4.999999999999989342, 11.31250000273118772 ) ) ;
#4249=CARTESIAN_POINT ( 'NONE',  ( 104.9999999999999574, -2.071067811865462627, 4.437500000000000000 ) ) ;
#4267=CARTESIAN_POINT ( 'NONE',  ( 103.1528011352953342, 3.152801135295383084, 3.062500001365592528 ) ) ;
#4284=CARTESIAN_POINT ( 'NONE',  ( 98.15313185440925281, 4.458734125000016313, 4.500000001365592084 ) ) ;
#4300=CARTESIAN_POINT ( 'NONE',  ( 96.84719886470459471, -3.152801135295355994, 1.562500001365591418 ) ) ;
#4303=CARTESIAN_POINT ( 'NONE',  ( 99.99999999999995737, 4.458734125000016313, 13.18750000136559208 ) ) ;
#4310=EDGE_CURVE ( 'NONE', #2357, #2527, #14284, .T. ) ;
#4321=AXIS2_PLACEMENT_3D ( 'NONE', #26443, #23594, #13007 ) ;
#4334=CARTESIAN_POINT ( 'NONE',  ( 104.4587341249999781, 1.846868145590750521, 11.25000000136559386 ) ) ;
#4344=ORIENTED_EDGE ( 'NONE', *, *, #18830, .T. ) ;
#4349=CARTESIAN_POINT ( 'NONE',  ( 94.99999999999995737, -2.071067811865466624, 2.187500002731185500 ) ) ;
#4355=CARTESIAN_POINT ( 'NONE',  ( 104.9999999999999716, 1.449011120738813565E-14, 34.79898987322334136 ) ) ;
#4365=CARTESIAN_POINT ( 'NONE',  ( 101.8468681455906903, 4.458734125000016313, 8.125000001365592084 ) ) ;
#4369=CARTESIAN_POINT ( 'NONE',  ( 98.15313185440925281, 4.458734125000016313, 13.25000000136559208 ) ) ;
#4392=CARTESIAN_POINT ( 'NONE',  ( 99.99999999999995737, -4.999999999999990230, 6.249999999999998224 ) ) ;
#4410=CARTESIAN_POINT ( 'NONE',  ( 99.99999999999995737, -4.458734124999988779, 3.687500001365591640 ) ) ;
#4419=VERTEX_POINT ( 'NONE', #18491 ) ;
#4429=CARTESIAN_POINT ( 'NONE',  ( 95.54126587499995082, 1.846868145590750077, 1.625000001365592972 ) ) ;
#4443=CARTESIAN_POINT ( 'NONE',  ( 101.8468681455906903, -4.458734124999987891, 11.00000000136559208 ) ) ;
#4445=CARTESIAN_POINT ( 'NONE',  ( 95.54126587499996504, 1.387778780781445676E-14, 13.43750000136559386 ) ) ;
#4447=DIRECTION ( 'NONE',  ( 1.000000000000000000, 0.000000000000000000, 0.000000000000000000 ) ) ;
#4461=CARTESIAN_POINT ( 'NONE',  ( 103.1528011352953342, 3.152801135295383084, 13.31250000136559386 ) ) ;
#4478=CARTESIAN_POINT ( 'NONE',  ( 95.54126587499996504, 1.387778780781445676E-14, 9.687500001365593860 ) ) ;
#4479=( BOUNDED_CURVE ( )  B_SPLINE_CURVE ( 2, ( #25280, #20738, #25012, #25562, #14576, #7758, #14710, #18861, #27710 ),
 .UNSPECIFIED., .F., .T. ) 
 B_SPLINE_CURVE_WITH_KNOTS ( ( 3, 2, 2, 2, 3 ),
 ( 0.8571428571428570953, 0.8660714285714286031, 0.8750000000000000000, 0.8839285714285712858, 0.8928571428571427937 ),
 .UNSPECIFIED. ) 
 CURVE ( )  GEOMETRIC_REPRESENTATION_ITEM ( )  RATIONAL_B_SPLINE_CURVE ( ( 1.000000000000000000, 0.9238795325112867385, 1.000000000000000000, 0.9238795325112867385, 1.000000000000000000, 0.9238795325112867385, 1.000000000000000000, 0.9238795325112877377, 0.9999999999999990008 ) ) 
 REPRESENTATION_ITEM ( '' )  );
#4491=CARTESIAN_POINT ( 'NONE',  ( 97.92893218813451028, -4.999999999999989342, 1.312500002731184612 ) ) ;
#4495=ORIENTED_EDGE ( 'NONE', *, *, #3570, .T. ) ;
#4496=CARTESIAN_POINT ( 'NONE',  ( 84.99999999999998579, -14.99999999999999467, 15.00000000000000000 ) ) ;
#4507=CARTESIAN_POINT ( 'NONE',  ( 98.15313185440925281, 4.458734125000016313, 10.25000000136559386 ) ) ;
#4510=CARTESIAN_POINT ( 'NONE',  ( 99.99999999999995737, -4.458734124999988779, 11.68750000136559208 ) ) ;
#4531=CARTESIAN_POINT ( 'NONE',  ( 103.5355339059327093, 3.535533905932755072, 6.624999999999999112 ) ) ;
#4538=CARTESIAN_POINT ( 'NONE',  ( 96.46446609406721961, 3.535533905932755072, 6.874999999999999112 ) ) ;
#4549=CARTESIAN_POINT ( 'NONE',  ( 103.1528011352953342, -3.152801135295355106, 1.812500001365591640 ) ) ;
#4565=CARTESIAN_POINT ( 'NONE',  ( 98.15313185440925281, -4.458734124999987891, 1.875000001365591862 ) ) ;
#4580=CARTESIAN_POINT ( 'NONE',  ( 104.4587341249999781, -1.846868145590721655, 10.12500000136559386 ) ) ;
#4582=CARTESIAN_POINT ( 'NONE',  ( 104.4587341249999781, 1.846868145590750299, 2.000000001365591640 ) ) ;
#4585=CARTESIAN_POINT ( 'NONE',  ( 99.99999999999995737, 1.387778780781445676E-14, 34.79898987322334136 ) ) ;
#4595=CARTESIAN_POINT ( 'NONE',  ( 104.9999999999999716, 1.449011120738813565E-14, 7.625000002731185056 ) ) ;
#4597=FACE_OUTER_BOUND ( 'NONE', #20007, .T. ) ;
#4598=EDGE_LOOP ( 'NONE', ( #3415, #23865, #7640, #25561 ) ) ;
#4616=CARTESIAN_POINT ( 'NONE',  ( 104.4587341249999781, 1.846868145590750521, 10.25000000136559031 ) ) ;
#4624=LINE ( 'NONE', #13281, #3478 ) ;
#4628=ORIENTED_EDGE ( 'NONE', *, *, #9306, .T. ) ;
#4637=FACE_OUTER_BOUND ( 'NONE', #3217, .T. ) ;
#4649=CARTESIAN_POINT ( 'NONE',  ( 101.8468681455906903, -4.458734124999987891, 9.750000001365593860 ) ) ;
#4652=CARTESIAN_POINT ( 'NONE',  ( 98.15313185440925281, 4.458734125000016313, 11.25000000136559031 ) ) ;
#4653=CARTESIAN_POINT ( 'NONE',  ( 104.9999999999999574, 2.071067811865501263, 8.562499999999998224 ) ) ;
#4665=ADVANCED_FACE ( 'NONE', ( #1802 ), #25589, .T. ) ;
#4670=CARTESIAN_POINT ( 'NONE',  ( 97.92893218813451028, 5.000000000000018652, 9.937500002731184168 ) ) ;
#4694=CARTESIAN_POINT ( 'NONE',  ( 103.1528011352953342, -3.152801135295355106, 2.812500001365592528 ) ) ;
#4700=EDGE_LOOP ( 'NONE', ( #16748, #15031, #19357, #25768 ) ) ;
#4711=CARTESIAN_POINT ( 'NONE',  ( 102.0710678118654329, 5.000000000000018652, 11.68750000000000000 ) ) ;
#4725=CARTESIAN_POINT ( 'NONE',  ( 104.4587341249999639, 1.442382525525748735E-14, 11.18750000136559208 ) ) ;
#4728=CARTESIAN_POINT ( 'NONE',  ( 95.54126587499996504, 1.846868145590750077, 12.37500000136559208 ) ) ;
#4735=EDGE_LOOP ( 'NONE', ( #23153, #27580, #17982, #2378 ) ) ;
#4738=CARTESIAN_POINT ( 'NONE',  ( 102.0710678118654329, -4.999999999999989342, 12.43750000273118950 ) ) ;
#4751=ORIENTED_EDGE ( 'NONE', *, *, #11675, .T. ) ;
#4760=CARTESIAN_POINT ( 'NONE',  ( 95.54126587499996504, 1.387778780781445676E-14, 12.68750000136559208 ) ) ;
#4770=AXIS2_PLACEMENT_3D ( 'NONE', #19877, #26300, #15445 ) ;
#4790=VERTEX_POINT ( 'NONE', #21600 ) ;
#4791=CARTESIAN_POINT ( 'NONE',  ( 101.8468681455906903, -4.458734124999987891, 4.750000001365592084 ) ) ;
#4794=CARTESIAN_POINT ( 'NONE',  ( 104.4587341249999639, 1.442382525525748735E-14, 9.937500001365592084 ) ) ;
#4803=VECTOR ( 'NONE', #27473, 1000.000000000000000 ) ;
#4805=CARTESIAN_POINT ( 'NONE',  ( 104.9999999999999716, 1.449011120738813565E-14, 11.62500000273118417 ) ) ;
#4812=CARTESIAN_POINT ( 'NONE',  ( 102.0710678118654329, -4.999999999999989342, 9.437500002731182391 ) ) ;
#4815=ADVANCED_FACE ( 'NONE', ( #10609 ), #2078, .F. ) ;
#4828=ADVANCED_FACE ( 'NONE', ( #17742 ), #11162, .F. ) ;
#4842=CARTESIAN_POINT ( 'NONE',  ( 95.54126587499996504, 1.846868145590750077, 2.375000001365592084 ) ) ;
#4856=CARTESIAN_POINT ( 'NONE',  ( 96.46446609406721961, 3.535533905932755072, 12.87500000000000000 ) ) ;
#4872=CARTESIAN_POINT ( 'NONE',  ( 95.54126587499996504, 1.387778780781445676E-14, 11.68750000136559208 ) ) ;
#4874=CARTESIAN_POINT ( 'NONE',  ( 96.84719886470459471, -3.152801135295355994, 1.562500001365591418 ) ) ;
#4877=CARTESIAN_POINT ( 'NONE',  ( 99.99999999999995737, 1.387778780781445676E-14, 34.79898987322334136 ) ) ;
#4889=CARTESIAN_POINT ( 'NONE',  ( 103.1528011352953342, 3.152801135295383084, 9.312500001365593860 ) ) ;
#4906=CARTESIAN_POINT ( 'NONE',  ( 104.4587341249999781, 1.846868145590750521, 7.250000001365592084 ) ) ;
#4910=CARTESIAN_POINT ( 'NONE',  ( 104.9999999999999716, 1.449011120738813565E-14, 0.6250000027311856110 ) ) ;
#4912=ADVANCED_FACE ( 'NONE', ( #4637 ), #25873, .T. ) ;
#4913=ORIENTED_EDGE ( 'NONE', *, *, #20584, .F. ) ;
#4924=VERTEX_POINT ( 'NONE', #11021 ) ;
#4927=DIRECTION ( 'NONE',  ( -1.000000000000000000, 0.000000000000000000, 0.000000000000000000 ) ) ;
#4928=LINE ( 'NONE', #7179, #1331 ) ;
#4935=CARTESIAN_POINT ( 'NONE',  ( 104.4587341249999639, 1.442382525525748735E-14, 5.937500001365592084 ) ) ;
#4938=CARTESIAN_POINT ( 'NONE',  ( 104.4587341249999781, -1.846868145590721655, 7.875000001365591196 ) ) ;
#4954=( BOUNDED_CURVE ( )  B_SPLINE_CURVE ( 2, ( #8009, #14559, #11994, #23274, #23689, #19826, #16977, #17114, #6435 ),
 .UNSPECIFIED., .F., .F. ) 
 B_SPLINE_CURVE_WITH_KNOTS ( ( 3, 2, 2, 2, 3 ),
 ( 0.7142857142857141906, 0.7232142857142855874, 0.7321428571428569843, 0.7410714285714286031, 0.7500000000000000000 ),
 .UNSPECIFIED. ) 
 CURVE ( )  GEOMETRIC_REPRESENTATION_ITEM ( )  RATIONAL_B_SPLINE_CURVE ( ( 1.000000000000000888, 0.9238795325112857393, 1.000000000000000000, 0.9238795325112867385, 1.000000000000000000, 0.9238795325112867385, 1.000000000000000000, 0.9238795325112867385, 1.000000000000000000 ) ) 
 REPRESENTATION_ITEM ( '' )  );
#4957=CARTESIAN_POINT ( 'NONE',  ( 102.0710678118654329, -4.999999999999989342, 11.43750000273118772 ) ) ;
#4974=APPLICATION_CONTEXT ( 'automotive_design' ) ;
#4989=ORIENTED_EDGE ( 'NONE', *, *, #21359, .F. ) ;
#4992=CARTESIAN_POINT ( 'NONE',  ( 96.46446609406721961, 3.535533905932755072, 5.875000000000000000 ) ) ;
#4997=ADVANCED_FACE ( 'NONE', ( #8762, #24018 ), #15302, .T. ) ;
#5002=CARTESIAN_POINT ( 'NONE',  ( 104.9999999999999574, 2.071067811865491937, 11.56249999999999822 ) ) ;
#5008=FACE_OUTER_BOUND ( 'NONE', #10724, .T. ) ;
#5014=CARTESIAN_POINT ( 'NONE',  ( 99.99999999999995737, -4.458734124999988779, 9.937500001365593860 ) ) ;
#5016=CARTESIAN_POINT ( 'NONE',  ( 95.54126587499996504, 1.387778780781445676E-14, 8.437500001365592084 ) ) ;
#5026=EDGE_CURVE ( 'NONE', #17053, #13106, #26884, .T. ) ;
#5030=CARTESIAN_POINT ( 'NONE',  ( 103.1528011352953342, -3.152801135295355106, 9.062500001365592084 ) ) ;
#5046=CARTESIAN_POINT ( 'NONE',  ( 104.4587341249999781, 1.846868145590750521, 8.250000001365592084 ) ) ;
#5070=EDGE_CURVE ( 'NONE', #11095, #14819, #20169, .T. ) ;
#5072=CARTESIAN_POINT ( 'NONE',  ( 102.0710678118654329, -4.999999999999989342, 2.437500002731185056 ) ) ;
#5077=CARTESIAN_POINT ( 'NONE',  ( 98.15313185440925281, -4.458734124999987891, 3.625000001365591640 ) ) ;
#5079=CARTESIAN_POINT ( 'NONE',  ( 101.8468681455906903, -4.458734124999987891, 7.750000001365592084 ) ) ;
#5082=CARTESIAN_POINT ( 'NONE',  ( 99.99999999999995737, 1.387778780781445676E-14, 34.79898987322334136 ) ) ;
#5095=CARTESIAN_POINT ( 'NONE',  ( 104.9999999999999574, -2.071067811865462627, 9.562500002731184168 ) ) ;
#5100=CARTESIAN_POINT ( 'NONE',  ( 99.99999999999995737, -4.999999999999990230, 1.249999999999999334 ) ) ;
#5102=EDGE_CURVE ( 'NONE', #4419, #23118, #1580, .T. ) ;
#5135=CARTESIAN_POINT ( 'NONE',  ( 96.46446609406721961, -3.535533905932727539, 9.250000002731184168 ) ) ;
#5137=CARTESIAN_POINT ( 'NONE',  ( 102.0710678118654329, -4.999999999999989342, 14.31249999999999822 ) ) ;
#5145=CARTESIAN_POINT ( 'NONE',  ( 96.46446609406721961, -3.535533905932727539, 3.124999999999999112 ) ) ;
#5151=EDGE_CURVE ( 'NONE', #2199, #27806, #4479, .T. ) ;
#5154=CARTESIAN_POINT ( 'NONE',  ( 95.54126587499996504, 1.387778780781445676E-14, 6.687500001365592084 ) ) ;
#5155=CARTESIAN_POINT ( 'NONE',  ( 103.1528011352953342, -3.152801135295355106, 8.812500001365592084 ) ) ;
#5169=CARTESIAN_POINT ( 'NONE',  ( 101.8468681455906903, 4.458734125000016313, 11.37500000136559386 ) ) ;
#5178=CIRCLE ( 'NONE', #27037, 5.000000000000004441 ) ;
#5187=CARTESIAN_POINT ( 'NONE',  ( 101.8468681455907046, -4.458734124999987891, 8.000000001365592084 ) ) ;
#5206=CARTESIAN_POINT ( 'NONE',  ( 104.9999999999999858, -2.071067811865457298, 13.43749999999999822 ) ) ;
#5209=EDGE_CURVE ( 'NONE', #24544, #3701, #12014, .T. ) ;
#5217=CARTESIAN_POINT ( 'NONE',  ( 96.84719886470459471, -3.152801135295355994, 5.562500001365591196 ) ) ;
#5220=CARTESIAN_POINT ( 'NONE',  ( 103.1528011352953342, -3.152801135295355106, 6.812500001365592084 ) ) ;
#5236=CARTESIAN_POINT ( 'NONE',  ( 104.9999999999999716, 1.449011120738813565E-14, 11.62500000273118417 ) ) ;
#5241=DIRECTION ( 'NONE',  ( -0.000000000000000000, -0.000000000000000000, -1.000000000000000000 ) ) ;
#5242=CARTESIAN_POINT ( 'NONE',  ( 104.9999999999999716, 1.449011120738813565E-14, 1.499999999999999556 ) ) ;
#5247=CARTESIAN_POINT ( 'NONE',  ( 96.46446609406721961, 3.535533905932755072, 6.000000002731185056 ) ) ;
#5277=VECTOR ( 'NONE', #18537, 1000.000000000000000 ) ;
#5278=AXIS2_PLACEMENT_3D ( 'NONE', #4877, #9563, #13541 ) ;
#5281=CARTESIAN_POINT ( 'NONE',  ( 99.99999999999995737, -4.999999999999990230, 13.25000000000000000 ) ) ;
#5286=CARTESIAN_POINT ( 'NONE',  ( 97.92893218813451028, 5.000000000000018652, 12.93750000273118772 ) ) ;
#5287=CARTESIAN_POINT ( 'NONE',  ( 104.9999999999999716, 1.449011120738813565E-14, 34.79898987322334136 ) ) ;
#5295=CARTESIAN_POINT ( 'NONE',  ( 101.8468681455906903, -4.458734124999987891, 6.000000001365591196 ) ) ;
#5297=CARTESIAN_POINT ( 'NONE',  ( 95.54126587499996504, 1.387778780781445676E-14, 11.43750000136559208 ) ) ;
#5307=EDGE_CURVE ( 'NONE', #9633, #9529, #10293, .T. ) ;
#5313=CARTESIAN_POINT ( 'NONE',  ( 103.1528011352953342, 3.152801135295383084, 11.31250000136559386 ) ) ;
#5326=ORIENTED_EDGE ( 'NONE', *, *, #7051, .F. ) ;
#5328=CARTESIAN_POINT ( 'NONE',  ( 104.4587341249999639, 1.442382525525748735E-14, 7.187500001365592972 ) ) ;
#5331=CARTESIAN_POINT ( 'NONE',  ( 103.5355339059327093, 3.535533905932755072, 6.750000002731185056 ) ) ;
#5350=CARTESIAN_POINT ( 'NONE',  ( 94.99999999999995737, 2.071067811865500818, 9.062500002731182391 ) ) ;
#5359=CARTESIAN_POINT ( 'NONE',  ( 101.8468681455906903, 4.458734125000016313, 5.125000001365592972 ) ) ;
#5362=CARTESIAN_POINT ( 'NONE',  ( 103.1528011352953342, 3.152801135295383084, 8.062500001365592084 ) ) ;
#5366=CARTESIAN_POINT ( 'NONE',  ( 94.99999999999997158, -2.071067811865486608, 5.062499999999999112 ) ) ;
#5370=VECTOR ( 'NONE', #7859, 1000.000000000000000 ) ;
#5373=DIRECTION ( 'NONE',  ( 1.000000000000000000, 0.000000000000000000, -0.000000000000000000 ) ) ;
#5379=CARTESIAN_POINT ( 'NONE',  ( 96.46446609406721961, -3.535533905932727539, 6.250000002731185056 ) ) ;
#5382=EDGE_CURVE ( 'NONE', #25436, #23888, #22103, .T. ) ;
#5414=VERTEX_POINT ( 'NONE', #24904 ) ;
#5425=CARTESIAN_POINT ( 'NONE',  ( 96.46446609406721961, 3.535533905932755072, 9.874999999999998224 ) ) ;
#5430=CARTESIAN_POINT ( 'NONE',  ( 103.5355339059327093, 3.535533905932755072, 11.75000000273118594 ) ) ;
#5438=CARTESIAN_POINT ( 'NONE',  ( 104.4587341249999781, 1.846868145590750299, 7.250000001365591196 ) ) ;
#5440=CARTESIAN_POINT ( 'NONE',  ( 104.4587341249999781, -1.846868145590721655, 8.875000001365592084 ) ) ;
#5453=CARTESIAN_POINT ( 'NONE',  ( 103.1528011352953342, -3.152801135295355106, 12.06250000136559208 ) ) ;
#5467=CYLINDRICAL_SURFACE ( 'NONE', #946, 5.000000000000004441 ) ;
#5468=CARTESIAN_POINT ( 'NONE',  ( 104.4587341249999781, 1.846868145590750521, 6.250000001365592084 ) ) ;
#5502=CARTESIAN_POINT ( 'NONE',  ( 104.4587341249999781, -1.846868145590721655, 13.12500000136559208 ) ) ;
#5520=CARTESIAN_POINT ( 'NONE',  ( 102.0710678118654329, -4.999999999999989342, 4.437500002731185944 ) ) ;
#5540=CARTESIAN_POINT ( 'NONE',  ( 94.99999999999995737, 1.387778780781445676E-14, 13.00000000000000000 ) ) ;
#5549=CARTESIAN_POINT ( 'NONE',  ( 103.5355339059327093, 3.535533905932755072, 2.750000002731185944 ) ) ;
#5569=CARTESIAN_POINT ( 'NONE',  ( 94.99999999999995737, 1.387778780781445676E-14, 9.000000000000000000 ) ) ;
#5574=CARTESIAN_POINT ( 'NONE',  ( 104.9999999999999574, 2.071067811865491937, 11.68750000273118772 ) ) ;
#5577=CARTESIAN_POINT ( 'NONE',  ( 97.92893218813451028, -4.999999999999989342, 11.18750000000000000 ) ) ;
#5582=CARTESIAN_POINT ( 'NONE',  ( 99.99999999999995737, 4.458734125000016313, 8.437500001365592084 ) ) ;
#5584=CARTESIAN_POINT ( 'NONE',  ( 98.15313185440923860, 4.458734125000016313, 11.25000000136559208 ) ) ;
#5590=ORIENTED_EDGE ( 'NONE', *, *, #7501, .F. ) ;
#5595=ORIENTED_EDGE ( 'NONE', *, *, #6007, .F. ) ;
#5597=CARTESIAN_POINT ( 'NONE',  ( 99.99999999999995737, -4.458734124999988779, 7.937500001365592084 ) ) ;
#5610=CARTESIAN_POINT ( 'NONE',  ( 96.84719886470459471, -3.152801135295355994, 4.812500001365592084 ) ) ;
#5619=CARTESIAN_POINT ( 'NONE',  ( 104.9999999999999716, 1.449011120738813565E-14, 3.625000002731184612 ) ) ;
#5625=ORIENTED_EDGE ( 'NONE', *, *, #10165, .F. ) ;
#5634=FACE_OUTER_BOUND ( 'NONE', #15713, .T. ) ;
#5636=CARTESIAN_POINT ( 'NONE',  ( 102.0710678118654329, -4.999999999999989342, 7.312500000000000000 ) ) ;
#5641=CARTESIAN_POINT ( 'NONE',  ( 96.84719886470459471, -3.152801135295355994, 0.5625000013655921949 ) ) ;
#5657=( BOUNDED_CURVE ( )  B_SPLINE_CURVE ( 2, ( #17177, #6350, #15024, #21607, #2085, #11312, #7181, #26450, #8909 ),
 .UNSPECIFIED., .F., .F. ) 
 B_SPLINE_CURVE_WITH_KNOTS ( ( 3, 2, 2, 2, 3 ),
 ( 0.2857142857142856984, 0.2946428571428571508, 0.3035714285714284921, 0.3124999999999999445, 0.3214285714285713969 ),
 .UNSPECIFIED. ) 
 CURVE ( )  GEOMETRIC_REPRESENTATION_ITEM ( )  RATIONAL_B_SPLINE_CURVE ( ( 1.000000000000000000, 0.9238795325112867385, 1.000000000000000000, 0.9238795325112867385, 1.000000000000000000, 0.9238795325112867385, 1.000000000000000000, 0.9238795325112871826, 0.9999999999999995559 ) ) 
 REPRESENTATION_ITEM ( '' )  );
#5658=CARTESIAN_POINT ( 'NONE',  ( 104.9999999999999574, -2.071067811865462627, 6.562500002731185056 ) ) ;
#5676=CARTESIAN_POINT ( 'NONE',  ( 104.4587341249999639, 1.442382525525748735E-14, 12.93750000136559208 ) ) ;
#5678=ORIENTED_EDGE ( 'NONE', *, *, #7373, .T. ) ;
#5684=CARTESIAN_POINT ( 'NONE',  ( 96.46446609406721961, 3.535533905932755072, 2.874999999999999112 ) ) ;
#5705=CARTESIAN_POINT ( 'NONE',  ( 97.92893218813451028, -4.999999999999989342, 11.18749999999999822 ) ) ;
#5711=CARTESIAN_POINT ( 'NONE',  ( 99.99999999999995737, -4.999999999999990230, 13.37500000273118417 ) ) ;
#5720=CARTESIAN_POINT ( 'NONE',  ( 98.15313185440925281, -4.458734124999987891, 8.875000001365593860 ) ) ;
#5723=CARTESIAN_POINT ( 'NONE',  ( 96.84719886470459471, -3.152801135295355994, 5.562500001365591196 ) ) ;
#5736=CARTESIAN_POINT ( 'NONE',  ( 98.15313185440925281, -4.458734124999987891, 8.875000001365593860 ) ) ;
#5750=CARTESIAN_POINT ( 'NONE',  ( 99.99999999999995737, -4.458734124999988779, 4.937500001365592972 ) ) ;
#5755=VERTEX_POINT ( 'NONE', #6575 ) ;
#5773=CARTESIAN_POINT ( 'NONE',  ( 94.99999999999995737, 1.387778780781445676E-14, 34.79898987322334136 ) ) ;
#5778=CARTESIAN_POINT ( 'NONE',  ( 96.84719886470459471, -3.152801135295355994, 2.562500001365592084 ) ) ;
#5780=CARTESIAN_POINT ( 'NONE',  ( 95.54126587499996504, 1.387778780781445676E-14, 13.68750000136559386 ) ) ;
#5797=VECTOR ( 'NONE', #20291, 1000.000000000000000 ) ;
#5798=CARTESIAN_POINT ( 'NONE',  ( 94.99999999999995737, -2.071067811865466624, 6.187500002731184168 ) ) ;
#5813=CARTESIAN_POINT ( 'NONE',  ( 95.54126587499995082, 1.846868145590750077, 12.37500000136559208 ) ) ;
#5815=VERTEX_POINT ( 'NONE', #2745 ) ;
#5818=CARTESIAN_POINT ( 'NONE',  ( 94.99999999999995737, 2.071067811865491493, 8.937500000000000000 ) ) ;
#5839=ORIENTED_EDGE ( 'NONE', *, *, #1180, .T. ) ;
#5840=CARTESIAN_POINT ( 'NONE',  ( 103.5355339059327093, -3.535533905932726206, 9.375000000000000000 ) ) ;
#5844=CARTESIAN_POINT ( 'NONE',  ( 94.99999999999995737, 2.071067811865491493, 14.06250000273118772 ) ) ;
#5846=DIRECTION ( 'NONE',  ( -0.000000000000000000, -0.000000000000000000, -1.000000000000000000 ) ) ;
#5847=CARTESIAN_POINT ( 'NONE',  ( 104.9999999999999716, 1.449011120738813565E-14, 11.62500000273118417 ) ) ;
#5855=CARTESIAN_POINT ( 'NONE',  ( 104.4587341249999781, -1.846868145590721655, 2.125000001365591640 ) ) ;
#5857=CARTESIAN_POINT ( 'NONE',  ( 104.4587341249999781, -1.846868145590721655, 4.875000001365592084 ) ) ;
#5873=CARTESIAN_POINT ( 'NONE',  ( 104.4587341249999781, -1.846868145590721655, 8.125000001365592084 ) ) ;
#5888=CARTESIAN_POINT ( 'NONE',  ( 96.84719886470459471, 3.152801135295383084, 4.312500001365592084 ) ) ;
#5889=DIRECTION ( 'NONE',  ( -1.000000000000000000, 0.000000000000000000, 0.000000000000000000 ) ) ;
#5890=CARTESIAN_POINT ( 'NONE',  ( 104.4587341249999781, -1.846868145590721655, 1.125000001365592750 ) ) ;
#5894=EDGE_CURVE ( 'NONE', #7171, #16160, #14850, .T. ) ;
#5902=LINE ( 'NONE', #16580, #13937 ) ;
#5920=CARTESIAN_POINT ( 'NONE',  ( 104.4587341249999639, 1.442382525525748735E-14, 13.18750000136559208 ) ) ;
#5922=CARTESIAN_POINT ( 'NONE',  ( 99.99999999999995737, 5.000000000000018652, 13.75000000000000000 ) ) ;
#5932=CARTESIAN_POINT ( 'NONE',  ( 94.99999999999995737, -2.071067811865466624, 5.187500002731184168 ) ) ;
#5948=CARTESIAN_POINT ( 'NONE',  ( 99.99999999999995737, 1.387778780781445676E-14, 34.79898987322334136 ) ) ;
#5949=CARTESIAN_POINT ( 'NONE',  ( 98.15313185440925281, -4.458734124999987891, 11.62500000136559031 ) ) ;
#5975=CARTESIAN_POINT ( 'NONE',  ( 104.9999999999999574, 2.071067811865491937, 8.562500000000000000 ) ) ;
#5979=CARTESIAN_POINT ( 'NONE',  ( 97.92893218813451028, 5.000000000000018652, 13.93750000273118772 ) ) ;
#5989=DIRECTION ( 'NONE',  ( -0.000000000000000000, -0.000000000000000000, -1.000000000000000000 ) ) ;
#5990=CARTESIAN_POINT ( 'NONE',  ( 98.15313185440925281, 4.458734125000016313, 3.500000001365592528 ) ) ;
#5992=CARTESIAN_POINT ( 'NONE',  ( 104.4587341249999781, 1.846868145590750521, 8.000000001365592084 ) ) ;
#6006=CARTESIAN_POINT ( 'NONE',  ( 95.54126587499996504, 1.387778780781445676E-14, 8.687500001365592084 ) ) ;
#6007=EDGE_CURVE ( 'NONE', #11095, #10159, #12374, .T. ) ;
#6014=FACE_OUTER_BOUND ( 'NONE', #2341, .T. ) ;
#6023=CARTESIAN_POINT ( 'NONE',  ( 103.1528011352953342, 3.152801135295383084, 2.062500001365591640 ) ) ;
#6025=CARTESIAN_POINT ( 'NONE',  ( 104.4587341249999781, 1.846868145590750521, 3.250000001365592972 ) ) ;
#6057=DIRECTION ( 'NONE',  ( -0.000000000000000000, -0.000000000000000000, -1.000000000000000000 ) ) ;
#6068=CARTESIAN_POINT ( 'NONE',  ( 99.99999999999995737, 4.458734125000016313, 14.18750000136559208 ) ) ;
#6085=CARTESIAN_POINT ( 'NONE',  ( 99.99999999999995737, 4.458734125000016313, 12.18750000136559208 ) ) ;
#6086=CARTESIAN_POINT ( 'NONE',  ( 97.92893218813451028, -4.999999999999989342, 13.31250000273118594 ) ) ;
#6110=CARTESIAN_POINT ( 'NONE',  ( 99.99999999999995737, -4.999999999999990230, 7.249999999999999112 ) ) ;
#6124=CARTESIAN_POINT ( 'NONE',  ( 104.4587341249999781, -1.846868145590721655, 4.125000001365592084 ) ) ;
#6127=CARTESIAN_POINT ( 'NONE',  ( 99.99999999999995737, 4.458734125000016313, 4.187500001365592084 ) ) ;
#6142=CARTESIAN_POINT ( 'NONE',  ( 103.1528011352953342, -3.152801135295355106, 2.062500001365591640 ) ) ;
#6152=VECTOR ( 'NONE', #18596, 1000.000000000000000 ) ;
#6157=CARTESIAN_POINT ( 'NONE',  ( 96.84719886470459471, -3.152801135295355994, 3.562500001365591196 ) ) ;
#6159=CARTESIAN_POINT ( 'NONE',  ( 101.8468681455907046, -4.458734124999987891, 2.000000001365591640 ) ) ;
#6172=DIRECTION ( 'NONE',  ( 1.000000000000000000, 0.000000000000000000, 0.000000000000000000 ) ) ;
#6186=ORIENTED_EDGE ( 'NONE', *, *, #9831, .F. ) ;
#6195=CARTESIAN_POINT ( 'NONE',  ( 104.9999999999999716, 1.449011120738813565E-14, 14.49999999999999822 ) ) ;
#6205=CARTESIAN_POINT ( 'NONE',  ( 96.46446609406721961, 3.535533905932755072, 2.000000002731185056 ) ) ;
#6212=CARTESIAN_POINT ( 'NONE',  ( 99.99999999999995737, 1.387778780781445676E-14, 34.79898987322334136 ) ) ;
#6222=EDGE_LOOP ( 'NONE', ( #28079, #2253, #4495, #177 ) ) ;
#6223=CARTESIAN_POINT ( 'NONE',  ( 95.54126587499995082, -1.846868145590724986, 9.500000001365593860 ) ) ;
#6227=CARTESIAN_POINT ( 'NONE',  ( 104.4587341249999781, 1.846868145590750299, 12.00000000136559208 ) ) ;
#6234=CARTESIAN_POINT ( 'NONE',  ( 94.99999999999995737, 1.387778780781445676E-14, 6.125000002731185056 ) ) ;
#6247=CARTESIAN_POINT ( 'NONE',  ( 94.99999999999995737, -2.071067811865466624, 5.062500000000000888 ) ) ;
#6253=CARTESIAN_POINT ( 'NONE',  ( 94.99999999999997158, 2.071067811865471953, 5.062500002731186832 ) ) ;
#6259=CARTESIAN_POINT ( 'NONE',  ( 98.15313185440925281, 4.458734125000016313, 4.500000001365592084 ) ) ;
#6261=CARTESIAN_POINT ( 'NONE',  ( 99.99999999999995737, 4.458734125000016313, 6.187500001365592084 ) ) ;
#6275=CARTESIAN_POINT ( 'NONE',  ( 103.1528011352953342, 3.152801135295383084, 1.312500001365592750 ) ) ;
#6288=CARTESIAN_POINT ( 'NONE',  ( 94.99999999999995737, 2.071067811865500818, 9.937499999999996447 ) ) ;
#6290=CARTESIAN_POINT ( 'NONE',  ( 103.1528011352953342, -3.152801135295355106, 0.8125000013655924169 ) ) ;
#6292=CARTESIAN_POINT ( 'NONE',  ( 99.99999999999995737, 4.458734125000016313, 2.187500001365592084 ) ) ;
#6310=VECTOR ( 'NONE', #14314, 1000.000000000000000 ) ;
#6324=CARTESIAN_POINT ( 'NONE',  ( 101.8468681455907046, 4.458734125000016313, 14.37500000136559386 ) ) ;
#6338=CARTESIAN_POINT ( 'NONE',  ( 96.46446609406721961, -3.535533905932727539, 0.2500000027311852779 ) ) ;
#6350=CARTESIAN_POINT ( 'NONE',  ( 94.99999999999995737, 2.071067811865491493, 10.93750000000000000 ) ) ;
#6355=CARTESIAN_POINT ( 'NONE',  ( 104.4587341249999639, 1.442382525525748735E-14, 6.937500001365592972 ) ) ;
#6359=CARTESIAN_POINT ( 'NONE',  ( 99.99999999999995737, 4.458734125000016313, 10.18750000136559208 ) ) ;
#6364=CARTESIAN_POINT ( 'NONE',  ( 92.99999999999995737, 1.387778780781445676E-14, 0.000000000000000000 ) ) ;
#6383=CARTESIAN_POINT ( 'NONE',  ( 94.99999999999995737, 2.071067811865491048, 5.937500000000000000 ) ) ;
#6393=CARTESIAN_POINT ( 'NONE',  ( 99.99999999999995737, 5.000000000000018652, 6.749999999999999112 ) ) ;
#6400=CARTESIAN_POINT ( 'NONE',  ( 96.84719886470459471, 3.152801135295383084, 1.562500001365592972 ) ) ;
#6403=CARTESIAN_POINT ( 'NONE',  ( 103.1528011352953342, -3.152801135295355106, 0.8125000013655924169 ) ) ;
#6412=ORIENTED_EDGE ( 'NONE', *, *, #23068, .T. ) ;
#6418=CARTESIAN_POINT ( 'NONE',  ( 103.1528011352953342, 3.152801135295383084, 3.312500001365592972 ) ) ;
#6431=CARTESIAN_POINT ( 'NONE',  ( 96.84719886470459471, -3.152801135295355994, 13.81250000136559208 ) ) ;
#6434=CARTESIAN_POINT ( 'NONE',  ( 95.54126587499995082, 1.846868145590750077, 4.375000001365592084 ) ) ;
#6435=CARTESIAN_POINT ( 'NONE',  ( 104.9999999999999716, 1.449011120738813565E-14, 3.625000002731184612 ) ) ;
#6462=FILL_AREA_STYLE_COLOUR ( '', #12641 ) ;
#6463=CARTESIAN_POINT ( 'NONE',  ( 99.99999999999995737, -4.458734124999988779, 12.93750000136559208 ) ) ;
#6476=CARTESIAN_POINT ( 'NONE',  ( 97.92893218813451028, -4.999999999999989342, 0.3125000027311853890 ) ) ;
#6492=CARTESIAN_POINT ( 'NONE',  ( 104.4587341249999639, 1.442382525525748735E-14, 8.937500001365592084 ) ) ;
#6495=CARTESIAN_POINT ( 'NONE',  ( 103.1528011352953342, 3.152801135295383084, 13.06250000136559208 ) ) ;
#6502=CARTESIAN_POINT ( 'NONE',  ( 94.99999999999995737, 1.387778780781445676E-14, 12.00000000000000000 ) ) ;
#6508=ORIENTED_EDGE ( 'NONE', *, *, #10913, .F. ) ;
#6517=CARTESIAN_POINT ( 'NONE',  ( 97.92893218813451028, 5.000000000000018652, 5.812500000000000000 ) ) ;
#6534=CARTESIAN_POINT ( 'NONE',  ( 96.84719886470459471, -3.152801135295355994, 2.562500001365592084 ) ) ;
#6545=EDGE_CURVE ( 'NONE', #9529, #23888, #3894, .T. ) ;
#6550=CARTESIAN_POINT ( 'NONE',  ( 98.15313185440925281, -4.458734124999987891, 3.875000001365592084 ) ) ;
#6562=CARTESIAN_POINT ( 'NONE',  ( 104.9999999999999716, 2.071067811865491937, 9.562499999999998224 ) ) ;
#6563=CARTESIAN_POINT ( 'NONE',  ( 104.4587341249999781, -1.846868145590721655, 9.125000001365592084 ) ) ;
#6566=CARTESIAN_POINT ( 'NONE',  ( 96.84719886470459471, 3.152801135295383084, 1.312500001365592750 ) ) ;
#6575=CARTESIAN_POINT ( 'NONE',  ( 104.9999999999999716, 1.449011120738813565E-14, 10.49999999999999822 ) ) ;
#6580=CARTESIAN_POINT ( 'NONE',  ( 94.99999999999995737, -2.071067811865466624, 7.187500002731185056 ) ) ;
#6582=CARTESIAN_POINT ( 'NONE',  ( 95.54126587499995082, 1.846868145590750077, 13.62500000136559386 ) ) ;
#6599=CARTESIAN_POINT ( 'NONE',  ( 101.8468681455907046, -4.458734124999987891, 10.00000000136559386 ) ) ;
#6613=CARTESIAN_POINT ( 'NONE',  ( 104.9999999999999716, 1.449011120738813565E-14, 1.625000002731184834 ) ) ;
#6629=CARTESIAN_POINT ( 'NONE',  ( 101.8468681455906903, 4.458734125000016313, 10.12500000136559208 ) ) ;
#6630=VECTOR ( 'NONE', #20480, 1000.000000000000000 ) ;
#6631=ORIENTED_EDGE ( 'NONE', *, *, #9856, .F. ) ;
#6633=CARTESIAN_POINT ( 'NONE',  ( 95.54126587499996504, 1.387778780781445676E-14, 13.43750000136559386 ) ) ;
#6644=VERTEX_POINT ( 'NONE', #24600 ) ;
#6645=CARTESIAN_POINT ( 'NONE',  ( 103.5355339059327093, -3.535533905932726206, 8.375000000000000000 ) ) ;
#6650=ORIENTED_EDGE ( 'NONE', *, *, #18893, .T. ) ;
#6653=CARTESIAN_POINT ( 'NONE',  ( 96.46446609406721961, 3.535533905932755072, 5.875000000000000000 ) ) ;
#6671=CARTESIAN_POINT ( 'NONE',  ( 104.4587341249999781, -1.846868145590721655, 2.875000001365592528 ) ) ;
#6687=CARTESIAN_POINT ( 'NONE',  ( 95.54126587499996504, 1.387778780781445676E-14, 4.687500001365592084 ) ) ;
#6702=CARTESIAN_POINT ( 'NONE',  ( 98.15313185440925281, -4.458734124999987891, 12.87500000136559208 ) ) ;
#6704=CARTESIAN_POINT ( 'NONE',  ( 99.99999999999995737, 4.458734125000016313, 14.18750000136559208 ) ) ;
#6706=CARTESIAN_POINT ( 'NONE',  ( 99.99999999999995737, -4.458734124999988779, 0.9375000013655925279 ) ) ;
#6712=EDGE_CURVE ( 'NONE', #7853, #7171, #15784, .T. ) ;
#6715=DIRECTION ( 'NONE',  ( -0.000000000000000000, -0.000000000000000000, -1.000000000000000000 ) ) ;
#6723=CARTESIAN_POINT ( 'NONE',  ( 101.8468681455906903, -4.458734124999987891, 14.00000000136559208 ) ) ;
#6741=CARTESIAN_POINT ( 'NONE',  ( 101.8468681455907046, 4.458734125000016313, 9.375000001365593860 ) ) ;
#6751=AXIS2_PLACEMENT_3D ( 'NONE', #6212, #17451, #4079 ) ;
#6768=CYLINDRICAL_SURFACE ( 'NONE', #26517, 5.000000000000004441 ) ;
#6772=CARTESIAN_POINT ( 'NONE',  ( 101.8468681455906903, -4.458734124999987891, 10.75000000136559208 ) ) ;
#6774=CARTESIAN_POINT ( 'NONE',  ( 104.4587341249999781, 1.846868145590750299, 13.00000000136559386 ) ) ;
#6784=CARTESIAN_POINT ( 'NONE',  ( 96.46446609406721961, -3.535533905932727539, 11.25000000273118594 ) ) ;
#6791=CARTESIAN_POINT ( 'NONE',  ( 96.46446609406721961, 3.535533905932755072, 9.000000002731184168 ) ) ;
#6797=CARTESIAN_POINT ( 'NONE',  ( 103.5355339059327093, 3.535533905932755072, 1.624999999999999778 ) ) ;
#6815=CARTESIAN_POINT ( 'NONE',  ( 101.8468681455907046, 4.458734125000016313, 1.125000001365592750 ) ) ;
#6818=CARTESIAN_POINT ( 'NONE',  ( 102.0710678118654329, 5.000000000000018652, 4.687500000000000000 ) ) ;
#6832=CARTESIAN_POINT ( 'NONE',  ( 103.5355339059327093, -3.535533905932726206, 12.37499999999999822 ) ) ;
#6845=CARTESIAN_POINT ( 'NONE',  ( 95.54126587499995082, -1.846868145590724986, 11.75000000136559208 ) ) ;
#6848=CARTESIAN_POINT ( 'NONE',  ( 96.84719886470459471, -3.152801135295355994, 12.56250000136559208 ) ) ;
#6857=CARTESIAN_POINT ( 'NONE',  ( 103.5355339059327093, -3.535533905932726206, 12.50000000273118594 ) ) ;
#6867=CARTESIAN_POINT ( 'NONE',  ( 99.99999999999995737, -4.458734124999988779, 12.93750000136559208 ) ) ;
#6868=ORIENTED_EDGE ( 'NONE', *, *, #2814, .F. ) ;
#6884=CARTESIAN_POINT ( 'NONE',  ( 96.84719886470459471, -3.152801135295355994, 12.81250000136559208 ) ) ;
#6887=EDGE_CURVE ( 'NONE', #2879, #22694, #3917, .T. ) ;
#6900=EDGE_CURVE ( 'NONE', #22247, #25944, #22772, .T. ) ;
#6908=CARTESIAN_POINT ( 'NONE',  ( 94.99999999999995737, 1.387778780781445676E-14, 8.125000002731185944 ) ) ;
#6911=CARTESIAN_POINT ( 'NONE',  ( 95.54126587499995082, 1.846868145590750077, 6.375000001365592084 ) ) ;
#6914=CARTESIAN_POINT ( 'NONE',  ( 99.99999999999995737, 4.458734125000016313, 7.187500001365592084 ) ) ;
#6917=CARTESIAN_POINT ( 'NONE',  ( 94.99999999999995737, 2.071067811865491493, 7.062500002731185056 ) ) ;
#6933=CARTESIAN_POINT ( 'NONE',  ( 94.99999999999995737, 1.387778780781445676E-14, 11.12500000273118594 ) ) ;
#6938=CARTESIAN_POINT ( 'NONE',  ( 97.92893218813451028, 5.000000000000018652, 1.812500000000000000 ) ) ;
#6947=CARTESIAN_POINT ( 'NONE',  ( 96.46446609406721961, -3.535533905932727539, 10.25000000273118594 ) ) ;
#6957=CARTESIAN_POINT ( 'NONE',  ( 95.54126587499996504, 1.846868145590750077, 1.375000001365592972 ) ) ;
#6959=EDGE_LOOP ( 'NONE', ( #17524, #21105, #20037, #25056 ) ) ;
#6963=VERTEX_POINT ( 'NONE', #25963 ) ;
#6974=CARTESIAN_POINT ( 'NONE',  ( 103.5355339059327093, -3.535533905932726206, 14.37499999999999822 ) ) ;
#6975=VERTEX_POINT ( 'NONE', #313 ) ;
#6987=CARTESIAN_POINT ( 'NONE',  ( 95.54126587499996504, 1.387778780781445676E-14, 9.687500001365593860 ) ) ;
#6990=CARTESIAN_POINT ( 'NONE',  ( 103.1528011352953342, 3.152801135295383084, 1.062500001365592528 ) ) ;
#7004=CARTESIAN_POINT ( 'NONE',  ( 98.15313185440925281, -4.458734124999987891, 10.87500000136559386 ) ) ;
#7020=CARTESIAN_POINT ( 'NONE',  ( 103.1528011352953342, 3.152801135295383084, 11.31250000136559386 ) ) ;
#7038=CARTESIAN_POINT ( 'NONE',  ( 102.0710678118654329, -4.999999999999989342, 5.437500002731185056 ) ) ;
#7040=CARTESIAN_POINT ( 'NONE',  ( 104.9999999999999716, -2.071067811865462627, 2.562500002731185500 ) ) ;
#7046=CARTESIAN_POINT ( 'NONE',  ( 95.54126587499996504, 1.387778780781445676E-14, 4.437500001365592084 ) ) ;
#7049=CARTESIAN_POINT ( 'NONE',  ( 103.1528011352953342, 3.152801135295383084, 7.062500001365592084 ) ) ;
#7051=EDGE_CURVE ( 'NONE', #23888, #9529, #16819, .T. ) ;
#7070=CARTESIAN_POINT ( 'NONE',  ( 104.9999999999999716, 1.449011120738813565E-14, 8.625000002731185944 ) ) ;
#7076=CARTESIAN_POINT ( 'NONE',  ( 97.92893218813451028, 5.000000000000018652, 2.812499999999999112 ) ) ;
#7080=CARTESIAN_POINT ( 'NONE',  ( 99.99999999999995737, 1.387778780781445676E-14, 15.00000000000000000 ) ) ;
#7095=( BOUNDED_CURVE ( )  B_SPLINE_CURVE ( 2, ( #6502, #21623, #27902, #15178, #12479, #10492, #102, #25481, #8223 ),
 .UNSPECIFIED., .F., .F. ) 
 B_SPLINE_CURVE_WITH_KNOTS ( ( 3, 2, 2, 2, 3 ),
 ( 0.2142857142857142183, 0.2232142857142856707, 0.2321428571428570953, 0.2410714285714285199, 0.2499999999999999445 ),
 .UNSPECIFIED. ) 
 CURVE ( )  GEOMETRIC_REPRESENTATION_ITEM ( )  RATIONAL_B_SPLINE_CURVE ( ( 1.000000000000000444, 0.9238795325112862944, 1.000000000000000000, 0.9238795325112867385, 1.000000000000000000, 0.9238795325112867385, 1.000000000000000000, 0.9238795325112871826, 0.9999999999999995559 ) ) 
 REPRESENTATION_ITEM ( '' )  );
#7111=CARTESIAN_POINT ( 'NONE',  ( 94.99999999999995737, 1.387778780781445676E-14, 13.00000000000000000 ) ) ;
#7119=CARTESIAN_POINT ( 'NONE',  ( 103.5355339059327093, -3.535533905932726206, 3.374999999999999556 ) ) ;
#7126=CARTESIAN_POINT ( 'NONE',  ( 95.54126587499995082, -1.846868145590724986, 10.75000000136559208 ) ) ;
#7127=CARTESIAN_POINT ( 'NONE',  ( 94.99999999999995737, 1.387778780781445676E-14, 2.125000002731185056 ) ) ;
#7128=CARTESIAN_POINT ( 'NONE',  ( 95.54126587499996504, 1.846868145590750077, 13.37500000136559386 ) ) ;
#7131=DIRECTION ( 'NONE',  ( -0.000000000000000000, -0.000000000000000000, -1.000000000000000000 ) ) ;
#7136=VECTOR ( 'NONE', #23795, 1000.000000000000000 ) ;
#7138=CARTESIAN_POINT ( 'NONE',  ( 96.46446609406721961, -3.535533905932727539, 1.124999999999999334 ) ) ;
#7144=CARTESIAN_POINT ( 'NONE',  ( 95.54126587499996504, 1.387778780781445676E-14, 12.68750000136559208 ) ) ;
#7160=CARTESIAN_POINT ( 'NONE',  ( 98.15313185440923860, -4.458734124999987891, 6.875000001365592972 ) ) ;
#7163=CARTESIAN_POINT ( 'NONE',  ( 104.9999999999999716, 1.449011120738813565E-14, 14.49999999999999822 ) ) ;
#7171=VERTEX_POINT ( 'NONE', #19978 ) ;
#7179=CARTESIAN_POINT ( 'NONE',  ( 94.99999999999995737, 1.387778780781445676E-14, 34.79898987322334136 ) ) ;
#7181=CARTESIAN_POINT ( 'NONE',  ( 103.5355339059327093, 3.535533905932755072, 10.62499999999999822 ) ) ;
#7184=CARTESIAN_POINT ( 'NONE',  ( 103.1528011352953342, -3.152801135295355106, 4.812500001365592084 ) ) ;
#7187=CARTESIAN_POINT ( 'NONE',  ( 96.84719886470459471, -3.152801135295355994, 9.562500001365593860 ) ) ;
#7201=ORIENTED_EDGE ( 'NONE', *, *, #13476, .T. ) ;
#7206=CARTESIAN_POINT ( 'NONE',  ( 99.99999999999995737, 5.000000000000018652, 10.87500000273118594 ) ) ;
#7211=VERTEX_POINT ( 'NONE', #1034 ) ;
#7215=CARTESIAN_POINT ( 'NONE',  ( 104.9999999999999574, 2.071067811865491937, 2.562499999999998668 ) ) ;
#7220=CARTESIAN_POINT ( 'NONE',  ( 103.5355339059327093, 3.535533905932755072, 5.750000002731185056 ) ) ;
#7225=CARTESIAN_POINT ( 'NONE',  ( 102.0710678118654329, -4.999999999999989342, 10.43750000273118417 ) ) ;
#7238=ORIENTED_EDGE ( 'NONE', *, *, #19057, .F. ) ;
#7257=CARTESIAN_POINT ( 'NONE',  ( 95.54126587499995082, -1.846868145590724986, 0.7500000013655925279 ) ) ;
#7270=CARTESIAN_POINT ( 'NONE',  ( 94.99999999999995737, 1.387778780781445676E-14, 0.1250000027311851669 ) ) ;
#7271=CARTESIAN_POINT ( 'NONE',  ( 103.1528011352953342, 3.152801135295383084, 7.312500001365592084 ) ) ;
#7273=CARTESIAN_POINT ( 'NONE',  ( 101.8468681455907046, 4.458734125000016313, 10.12500000136559208 ) ) ;
#7283=CARTESIAN_POINT ( 'NONE',  ( 94.99999999999995737, 1.387778780781445676E-14, 0.9999999999999991118 ) ) ;
#7288=CARTESIAN_POINT ( 'NONE',  ( 103.1528011352953342, 3.152801135295383084, 12.31250000136559208 ) ) ;
#7304=ORIENTED_EDGE ( 'NONE', *, *, #6007, .T. ) ;
#7306=CARTESIAN_POINT ( 'NONE',  ( 104.4587341249999639, 1.442382525525748735E-14, 8.187500001365592084 ) ) ;
#7316=EDGE_LOOP ( 'NONE', ( #27150, #532, #901, #4150 ) ) ;
#7326=CARTESIAN_POINT ( 'NONE',  ( 97.92893218813451028, -4.999999999999989342, 5.312500002731184168 ) ) ;
#7334=CARTESIAN_POINT ( 'NONE',  ( 101.8468681455906903, -4.458734124999987891, 3.750000001365591640 ) ) ;
#7337=CARTESIAN_POINT ( 'NONE',  ( 99.99999999999995737, 4.458734125000016313, 6.187500001365592084 ) ) ;
#7346=FACE_OUTER_BOUND ( 'NONE', #20562, .T. ) ;
#7353=CARTESIAN_POINT ( 'NONE',  ( 94.99999999999995737, -2.071067811865466624, 10.18750000273118417 ) ) ;
#7373=EDGE_CURVE ( 'NONE', #26723, #896, #21624, .T. ) ;
#7376=CARTESIAN_POINT ( 'NONE',  ( 94.99999999999995737, 1.387778780781445676E-14, 4.125000002731185056 ) ) ;
#7398=CARTESIAN_POINT ( 'NONE',  ( 94.99999999999995737, 1.387778780781445676E-14, 13.99999999999999822 ) ) ;
#7413=CARTESIAN_POINT ( 'NONE',  ( 103.1528011352953342, 3.152801135295383084, 8.312500001365592084 ) ) ;
#7414=CARTESIAN_POINT ( 'NONE',  ( 95.54126587499996504, -1.846868145590724986, 10.50000000136559208 ) ) ;
#7417=CARTESIAN_POINT ( 'NONE',  ( 104.9999999999999716, 2.071067811865491937, 3.562499999999999556 ) ) ;
#7429=CARTESIAN_POINT ( 'NONE',  ( 101.8468681455906903, 4.458734125000016313, 10.37500000136559208 ) ) ;
#7443=EDGE_LOOP ( 'NONE', ( #21571, #6631, #20758, #23705 ) ) ;
#7446=CARTESIAN_POINT ( 'NONE',  ( 95.54126587499996504, 1.387778780781445676E-14, 5.687500001365591196 ) ) ;
#7451=CARTESIAN_POINT ( 'NONE',  ( 104.9999999999999716, 1.449011120738813565E-14, 2.499999999999998668 ) ) ;
#7466=CARTESIAN_POINT ( 'NONE',  ( 99.99999999999995737, -4.999999999999990230, 13.25000000000000000 ) ) ;
#7472=FACE_OUTER_BOUND ( 'NONE', #2752, .T. ) ;
#7477=CARTESIAN_POINT ( 'NONE',  ( 104.4587341249999639, 1.442382525525748735E-14, 3.937500001365591640 ) ) ;
#7478=ORIENTED_EDGE ( 'NONE', *, *, #2880, .T. ) ;
#7480=CARTESIAN_POINT ( 'NONE',  ( 104.4587341249999781, 1.846868145590750299, 8.000000001365592084 ) ) ;
#7484=CARTESIAN_POINT ( 'NONE',  ( 99.99999999999995737, -4.999999999999990230, 5.249999999999999112 ) ) ;
#7497=CARTESIAN_POINT ( 'NONE',  ( 102.0710678118654329, 5.000000000000018652, 6.812500002731185056 ) ) ;
#7501=EDGE_CURVE ( 'NONE', #27592, #27159, #23444, .T. ) ;
#7502=CARTESIAN_POINT ( 'NONE',  ( 102.0710678118654329, 5.000000000000018652, 14.68749999999999822 ) ) ;
#7526=DIRECTION ( 'NONE',  ( -0.8660254037844404840, 0.000000000000000000, 0.4999999999999967804 ) ) ;
#7545=CARTESIAN_POINT ( 'NONE',  ( 99.99999999999995737, -4.999999999999990230, 9.250000000000000000 ) ) ;
#7551=CARTESIAN_POINT ( 'NONE',  ( 97.92893218813451028, 5.000000000000018652, 11.93750000273118772 ) ) ;
#7553=DIRECTION ( 'NONE',  ( -1.000000000000000000, 0.000000000000000000, 0.000000000000000000 ) ) ;
#7559=CARTESIAN_POINT ( 'NONE',  ( 95.54126587499995082, 1.846868145590750077, 8.625000001365593860 ) ) ;
#7561=CARTESIAN_POINT ( 'NONE',  ( 104.4587341249999781, 1.846868145590750521, 11.00000000136559208 ) ) ;
#7572=ORIENTED_EDGE ( 'NONE', *, *, #21359, .T. ) ;
#7576=CARTESIAN_POINT ( 'NONE',  ( 95.54126587499996504, 1.387778780781445676E-14, 10.68750000136559208 ) ) ;
#7596=CARTESIAN_POINT ( 'NONE',  ( 104.4587341249999781, -1.846868145590721655, 5.125000001365592972 ) ) ;
#7601=CARTESIAN_POINT ( 'NONE',  ( 104.9999999999999858, -2.071067811865442643, 2.437500000000000000 ) ) ;
#7611=ORIENTED_EDGE ( 'NONE', *, *, #20993, .F. ) ;
#7628=CARTESIAN_POINT ( 'NONE',  ( 101.8468681455906903, 4.458734125000016313, 13.37500000136559386 ) ) ;
#7640=ORIENTED_EDGE ( 'NONE', *, *, #21540, .T. ) ;
#7646=CARTESIAN_POINT ( 'NONE',  ( 102.0710678118654329, -4.999999999999989342, 6.437500002731185056 ) ) ;
#7689=VERTEX_POINT ( 'NONE', #12698 ) ;
#7690=CARTESIAN_POINT ( 'NONE',  ( 104.9999999999999716, 1.449011120738813565E-14, 10.49999999999999822 ) ) ;
#7696=FACE_OUTER_BOUND ( 'NONE', #25034, .T. ) ;
#7704=CARTESIAN_POINT ( 'NONE',  ( 101.8468681455906903, -4.458734124999987891, 9.000000001365593860 ) ) ;
#7707=CARTESIAN_POINT ( 'NONE',  ( 95.54126587499996504, -1.846868145590724986, 9.500000001365593860 ) ) ;
#7711=CARTESIAN_POINT ( 'NONE',  ( 99.99999999999995737, -4.999999999999990230, 4.249999999999998224 ) ) ;
#7717=CARTESIAN_POINT ( 'NONE',  ( 94.99999999999995737, 1.387778780781445676E-14, 34.79898987322334136 ) ) ;
#7721=CARTESIAN_POINT ( 'NONE',  ( 103.1528011352953342, 3.152801135295383084, 8.312500001365592084 ) ) ;
#7736=CARTESIAN_POINT ( 'NONE',  ( 95.54126587499996504, 1.846868145590750077, 8.625000001365592084 ) ) ;
#7739=CARTESIAN_POINT ( 'NONE',  ( 94.99999999999995737, 2.071067811865491493, 8.062500002731185944 ) ) ;
#7755=EDGE_CURVE ( 'NONE', #16160, #20673, #26255, .T. ) ;
#7758=CARTESIAN_POINT ( 'NONE',  ( 102.0710678118654329, 5.000000000000018652, 1.812500002731185056 ) ) ;
#7763=CARTESIAN_POINT ( 'NONE',  ( 104.9999999999999716, -2.071067811865462627, 7.437500000000000000 ) ) ;
#7769=CARTESIAN_POINT ( 'NONE',  ( 99.99999999999995737, 4.458734125000016313, 1.187500001365592750 ) ) ;
#7787=CARTESIAN_POINT ( 'NONE',  ( 97.92893218813451028, 5.000000000000018652, 6.937500002731185944 ) ) ;
#7803=FACE_OUTER_BOUND ( 'NONE', #22872, .T. ) ;
#7804=CARTESIAN_POINT ( 'NONE',  ( 95.54126587499995082, 1.846868145590750077, 14.37500000136559386 ) ) ;
#7830=CARTESIAN_POINT ( 'NONE',  ( 103.5355339059327093, 3.535533905932755072, 8.624999999999998224 ) ) ;
#7831=VERTEX_POINT ( 'NONE', #22124 ) ;
#7836=CARTESIAN_POINT ( 'NONE',  ( 94.99999999999995737, 2.071067811865491048, 14.06250000273118772 ) ) ;
#7845=CARTESIAN_POINT ( 'NONE',  ( 96.84719886470459471, -3.152801135295355994, 5.812500001365591196 ) ) ;
#7847=CARTESIAN_POINT ( 'NONE',  ( 95.54126587499996504, -1.846868145590724986, 5.500000001365591196 ) ) ;
#7850=CARTESIAN_POINT ( 'NONE',  ( 97.92893218813451028, -4.999999999999989342, 4.187499999999998224 ) ) ;
#7853=VERTEX_POINT ( 'NONE', #9421 ) ;
#7859=DIRECTION ( 'NONE',  ( -0.000000000000000000, -0.000000000000000000, -1.000000000000000000 ) ) ;
#7860=CARTESIAN_POINT ( 'NONE',  ( 96.84719886470459471, -3.152801135295355994, 7.812500001365592084 ) ) ;
#7873=FACE_OUTER_BOUND ( 'NONE', #7316, .T. ) ;
#7874=CARTESIAN_POINT ( 'NONE',  ( 95.54126587499996504, 1.387778780781445676E-14, 2.687500001365592528 ) ) ;
#7879=ORIENTED_EDGE ( 'NONE', *, *, #17356, .T. ) ;
#7885=CARTESIAN_POINT ( 'NONE',  ( 94.99999999999995737, 1.387778780781445676E-14, 6.125000002731185056 ) ) ;
#7891=( GEOMETRIC_REPRESENTATION_CONTEXT ( 3 ) GLOBAL_UNCERTAINTY_ASSIGNED_CONTEXT ( ( #17530 ) ) GLOBAL_UNIT_ASSIGNED_CONTEXT ( ( #13440, #26151, #22598 ) ) REPRESENTATION_CONTEXT ( 'NONE', 'WORKASPACE' ) );
#7904=CARTESIAN_POINT ( 'NONE',  ( 98.15313185440925281, -4.458734124999987891, 2.625000001365592084 ) ) ;
#7905=CARTESIAN_POINT ( 'NONE',  ( 104.4587341249999781, 1.846868145590750521, 14.25000000136559208 ) ) ;
#7909=CIRCLE ( 'NONE', #18338, 5.000000000000004441 ) ;
#7920=CARTESIAN_POINT ( 'NONE',  ( 104.9999999999999574, 2.071067811865491937, 5.687500002731185056 ) ) ;
#7923=DIRECTION ( 'NONE',  ( -0.000000000000000000, -0.000000000000000000, -1.000000000000000000 ) ) ;
#7937=DIRECTION ( 'NONE',  ( -1.000000000000000000, 0.000000000000000000, 0.000000000000000000 ) ) ;
#7938=CARTESIAN_POINT ( 'NONE',  ( 95.54126587499995082, -1.846868145590724986, 13.50000000136559208 ) ) ;
#7963=CARTESIAN_POINT ( 'NONE',  ( 102.0710678118654329, -4.999999999999989342, 7.312500000000000000 ) ) ;
#7977=CARTESIAN_POINT ( 'NONE',  ( 101.8468681455906903, -4.458734124999987891, 5.000000001365592972 ) ) ;
#7979=VECTOR ( 'NONE', #21231, 1000.000000000000000 ) ;
#7980=CARTESIAN_POINT ( 'NONE',  ( 104.4587341249999639, 1.442382525525748735E-14, 4.937500001365592972 ) ) ;
#7983=CARTESIAN_POINT ( 'NONE',  ( 104.9999999999999716, -2.071067811865462627, 9.437500000000000000 ) ) ;
#7986=ORIENTED_EDGE ( 'NONE', *, *, #11387, .T. ) ;
#7994=CARTESIAN_POINT ( 'NONE',  ( 99.99999999999995737, -4.458734124999988779, 5.937500001365592084 ) ) ;
#8008=CARTESIAN_POINT ( 'NONE',  ( 95.54126587499996504, 1.387778780781445676E-14, 5.437500001365591196 ) ) ;
#8009=CARTESIAN_POINT ( 'NONE',  ( 94.99999999999995737, 1.387778780781445676E-14, 4.125000002731185056 ) ) ;
#8010=CARTESIAN_POINT ( 'NONE',  ( 104.4587341249999781, 1.846868145590750521, 1.250000001365592750 ) ) ;
#8013=CARTESIAN_POINT ( 'NONE',  ( 104.9999999999999716, 1.449011120738813565E-14, 8.625000002731185944 ) ) ;
#8022=DIRECTION ( 'NONE',  ( 0.000000000000000000, 0.000000000000000000, 1.000000000000000000 ) ) ;
#8029=CYLINDRICAL_SURFACE ( 'NONE', #11657, 5.000000000000004441 ) ;
#8042=CARTESIAN_POINT ( 'NONE',  ( 103.1528011352953342, 3.152801135295383084, 13.31250000136559386 ) ) ;
#8053=UNCERTAINTY_MEASURE_WITH_UNIT (LENGTH_MEASURE( 1.000000000000000082E-05 ), #16875, 'distance_accuracy_value', 'NONE');
#8057=CARTESIAN_POINT ( 'NONE',  ( 103.5355339059327093, 3.535533905932755072, 5.750000002731185056 ) ) ;
#8073=CYLINDRICAL_SURFACE ( 'NONE', #10873, 5.000000000000004441 ) ;
#8074=CARTESIAN_POINT ( 'NONE',  ( 104.4587341249999781, 1.846868145590750299, 14.00000000136559208 ) ) ;
#8080=CARTESIAN_POINT ( 'NONE',  ( 99.99999999999995737, 5.000000000000018652, 8.749999999999998224 ) ) ;
#8103=CARTESIAN_POINT ( 'NONE',  ( 102.0710678118654329, -4.999999999999989342, 10.31249999999999822 ) ) ;
#8113=CARTESIAN_POINT ( 'NONE',  ( 97.92893218813451028, -4.999999999999989342, 12.31250000273118950 ) ) ;
#8119=CARTESIAN_POINT ( 'NONE',  ( 103.1528011352953342, -3.152801135295355106, 3.062500001365592528 ) ) ;
#8121=CARTESIAN_POINT ( 'NONE',  ( 104.4587341249999781, -1.846868145590721655, 7.875000001365592084 ) ) ;
#8130=CARTESIAN_POINT ( 'NONE',  ( 95.54126587499996504, -1.846868145590724986, 0.5000000013655920839 ) ) ;
#8137=CARTESIAN_POINT ( 'NONE',  ( 98.15313185440925281, -4.458734124999987891, 6.875000001365592972 ) ) ;
#8147=ORIENTED_EDGE ( 'NONE', *, *, #14871, .T. ) ;
#8148=CIRCLE ( 'NONE', #3140, 7.000000000000006217 ) ;
#8152=CARTESIAN_POINT ( 'NONE',  ( 98.15313185440925281, -4.458734124999987891, 4.625000001365592084 ) ) ;
#8154=CARTESIAN_POINT ( 'NONE',  ( 104.4587341249999781, 1.846868145590750521, 4.250000001365592084 ) ) ;
#8173=CARTESIAN_POINT ( 'NONE',  ( 104.9999999999999716, 1.449011120738813565E-14, 34.79898987322334136 ) ) ;
#8186=CARTESIAN_POINT ( 'NONE',  ( 104.9999999999999716, 1.449011120738813565E-14, 13.50000000000000000 ) ) ;
#8193=ORIENTED_EDGE ( 'NONE', *, *, #5894, .F. ) ;
#8196=CARTESIAN_POINT ( 'NONE',  ( 98.15313185440925281, 4.458734125000016313, 14.25000000136559208 ) ) ;
#8213=CARTESIAN_POINT ( 'NONE',  ( 103.1528011352953342, 3.152801135295383084, 11.06250000136559208 ) ) ;
#8223=CARTESIAN_POINT ( 'NONE',  ( 104.9999999999999716, 1.449011120738813565E-14, 11.50000000000000000 ) ) ;
#8238=CARTESIAN_POINT ( 'NONE',  ( 99.99999999999995737, 5.000000000000018652, 6.749999999999999112 ) ) ;
#8241=EDGE_CURVE ( 'NONE', #12833, #25848, #2538, .T. ) ;
#8246=CARTESIAN_POINT ( 'NONE',  ( 102.0710678118654329, -4.999999999999989342, 11.31249999999999822 ) ) ;
#8253=CARTESIAN_POINT ( 'NONE',  ( 104.4587341249999781, 1.846868145590750299, 4.250000001365592084 ) ) ;
#8255=CARTESIAN_POINT ( 'NONE',  ( 101.8468681455907046, 4.458734125000016313, 6.125000001365592084 ) ) ;
#8270=CARTESIAN_POINT ( 'NONE',  ( 104.4587341249999781, -1.846868145590721655, 5.125000001365592972 ) ) ;
#8285=CARTESIAN_POINT ( 'NONE',  ( 104.4587341249999781, -1.846868145590721655, 5.875000001365591196 ) ) ;
#8287=CARTESIAN_POINT ( 'NONE',  ( 96.84719886470459471, 3.152801135295383084, 3.562500001365592972 ) ) ;
#8300=DIRECTION ( 'NONE',  ( -1.000000000000000000, 0.000000000000000000, 0.000000000000000000 ) ) ;
#8318=ORIENTED_EDGE ( 'NONE', *, *, #20993, .T. ) ;
#8321=CARTESIAN_POINT ( 'NONE',  ( 96.84719886470459471, 3.152801135295383084, 14.56250000136559208 ) ) ;
#8335=CARTESIAN_POINT ( 'NONE',  ( 99.99999999999995737, -4.999999999999990230, 2.375000002731185500 ) ) ;
#8351=CARTESIAN_POINT ( 'NONE',  ( 95.54126587499996504, 1.387778780781445676E-14, 12.43750000136559208 ) ) ;
#8355=CARTESIAN_POINT ( 'NONE',  ( 95.54126587499995082, -1.846868145590724986, 10.50000000136559208 ) ) ;
#8358=CARTESIAN_POINT ( 'NONE',  ( 99.99999999999995737, 5.000000000000018652, 2.749999999999999112 ) ) ;
#8378=CARTESIAN_POINT ( 'NONE',  ( 103.5355339059327093, 3.535533905932755072, 5.625000000000000000 ) ) ;
#8379=VERTEX_POINT ( 'NONE', #2395 ) ;
#8390=CARTESIAN_POINT ( 'NONE',  ( 101.8468681455906903, 4.458734125000016313, 3.375000001365592972 ) ) ;
#8392=CARTESIAN_POINT ( 'NONE',  ( 95.54126587499996504, -1.846868145590724986, 6.500000001365592084 ) ) ;
#8406=LINE ( 'NONE', #25942, #8525 ) ;
#8407=CARTESIAN_POINT ( 'NONE',  ( 96.84719886470459471, -3.152801135295355994, 2.812500001365592528 ) ) ;
#8421=CARTESIAN_POINT ( 'NONE',  ( 98.15313185440925281, -4.458734124999987891, 0.6250000013655921949 ) ) ;
#8422=ADVANCED_FACE ( 'NONE', ( #21775 ), #15047, .F. ) ;
#8424=CARTESIAN_POINT ( 'NONE',  ( 99.99999999999995737, 4.458734125000016313, 4.187500001365592084 ) ) ;
#8426=CARTESIAN_POINT ( 'NONE',  ( 104.4587341249999639, 1.442382525525748735E-14, 4.187500001365592084 ) ) ;
#8440=VECTOR ( 'NONE', #6057, 1000.000000000000000 ) ;
#8454=LINE ( 'NONE', #14715, #1057 ) ;
#8477=CARTESIAN_POINT ( 'NONE',  ( 94.99999999999995737, 1.387778780781445676E-14, 2.125000002731185056 ) ) ;
#8483=DIRECTION ( 'NONE',  ( 0.000000000000000000, -0.000000000000000000, -1.000000000000000000 ) ) ;
#8487=CARTESIAN_POINT ( 'NONE',  ( 102.0710678118654329, 5.000000000000018652, 9.812500002731184168 ) ) ;
#8493=DIRECTION ( 'NONE',  ( -0.000000000000000000, -0.000000000000000000, -1.000000000000000000 ) ) ;
#8495=CARTESIAN_POINT ( 'NONE',  ( 96.84719886470459471, -3.152801135295355994, 7.562500001365592084 ) ) ;
#8499=CARTESIAN_POINT ( 'NONE',  ( 98.15313185440925281, -4.458734124999987891, 10.62500000136559208 ) ) ;
#8510=CARTESIAN_POINT ( 'NONE',  ( 104.9999999999999716, -2.071067811865467956, 11.56250000273118594 ) ) ;
#8521=CARTESIAN_POINT ( 'NONE',  ( 94.99999999999995737, 1.387778780781445676E-14, 5.999999999999998224 ) ) ;
#8522=CARTESIAN_POINT ( 'NONE',  ( 99.99999999999995737, 5.000000000000018652, 1.749999999999999778 ) ) ;
#8525=VECTOR ( 'NONE', #21398, 1000.000000000000000 ) ;
#8529=CARTESIAN_POINT ( 'NONE',  ( 104.9999999999999716, -2.071067811865452857, 10.56250000273118417 ) ) ;
#8535=CARTESIAN_POINT ( 'NONE',  ( 95.54126587499995082, -1.846868145590724986, 1.750000001365591862 ) ) ;
#8537=CARTESIAN_POINT ( 'NONE',  ( 95.54126587499996504, 1.387778780781445676E-14, 1.437500001365591196 ) ) ;
#8552=CARTESIAN_POINT ( 'NONE',  ( 101.8468681455906903, -4.458734124999987891, 1.000000001365592528 ) ) ;
#8563=EDGE_CURVE ( 'NONE', #19876, #12833, #12158, .T. ) ;
#8567=CARTESIAN_POINT ( 'NONE',  ( 103.1528011352953342, 3.152801135295383084, 14.31250000136559208 ) ) ;
#8569=CARTESIAN_POINT ( 'NONE',  ( 101.8468681455906903, -4.458734124999987891, 4.750000001365592084 ) ) ;
#8585=FACE_OUTER_BOUND ( 'NONE', #10412, .T. ) ;
#8603=CARTESIAN_POINT ( 'NONE',  ( 104.4587341249999781, -1.846868145590721655, 10.12500000136559386 ) ) ;
#8609=CARTESIAN_POINT ( 'NONE',  ( 94.99999999999995737, -2.071067811865475949, 12.06249999999999822 ) ) ;
#8610=VECTOR ( 'NONE', #14866, 1000.000000000000000 ) ;
#8617=CARTESIAN_POINT ( 'NONE',  ( 99.99999999999995737, 5.000000000000018652, 0.8750000027311858330 ) ) ;
#8623=FACE_OUTER_BOUND ( 'NONE', #295, .T. ) ;
#8629=( BOUNDED_CURVE ( )  B_SPLINE_CURVE ( 2, ( #10647, #14510, #19353, #28056, #8522, #17208, #1707, #19076, #25913 ),
 .UNSPECIFIED., .F., .T. ) 
 B_SPLINE_CURVE_WITH_KNOTS ( ( 3, 2, 2, 2, 3 ),
 ( 0.9285714285714284921, 0.9374999999999998890, 0.9464285714285712858, 0.9553571428571427937, 0.9642857142857141906 ),
 .UNSPECIFIED. ) 
 CURVE ( )  GEOMETRIC_REPRESENTATION_ITEM ( )  RATIONAL_B_SPLINE_CURVE ( ( 1.000000000000000888, 0.9238795325112857393, 1.000000000000000000, 0.9238795325112867385, 1.000000000000000000, 0.9238795325112867385, 1.000000000000000000, 0.9238795325112877377, 0.9999999999999990008 ) ) 
 REPRESENTATION_ITEM ( '' )  );
#8635=CARTESIAN_POINT ( 'NONE',  ( 0.000000000000000000, 0.000000000000000000, 0.000000000000000000 ) ) ;
#8636=CARTESIAN_POINT ( 'NONE',  ( 99.99999999999995737, -4.458734124999988779, 8.687500001365592084 ) ) ;
#8639=CARTESIAN_POINT ( 'NONE',  ( 98.15313185440925281, 4.458734125000016313, 12.25000000136559208 ) ) ;
#8660=CARTESIAN_POINT ( 'NONE',  ( 103.5355339059327093, 3.535533905932755072, 4.624999999999999112 ) ) ;
#8679=CARTESIAN_POINT ( 'NONE',  ( 95.54126587499996504, 1.387778780781445676E-14, 0.4375000013655920839 ) ) ;
#8685=ORIENTED_EDGE ( 'NONE', *, *, #21200, .F. ) ;
#8689=EDGE_LOOP ( 'NONE', ( #15677, #4344, #2510, #5590 ) ) ;
#8694=CARTESIAN_POINT ( 'NONE',  ( 104.4587341249999639, 1.442382525525748735E-14, 2.187500001365592084 ) ) ;
#8700=CARTESIAN_POINT ( 'NONE',  ( 99.99999999999995737, 1.387778780781445676E-14, 34.79898987322334136 ) ) ;
#8706=CARTESIAN_POINT ( 'NONE',  ( 99.99999999999995737, 5.000000000000018652, 9.749999999999998224 ) ) ;
#8707=CARTESIAN_POINT ( 'NONE',  ( 103.1528011352953342, 3.152801135295383084, 9.312500001365593860 ) ) ;
#8709=CARTESIAN_POINT ( 'NONE',  ( 104.4587341249999639, 1.442382525525748735E-14, 13.93750000136559208 ) ) ;
#8716=ORIENTED_EDGE ( 'NONE', *, *, #5209, .F. ) ;
#8717=CARTESIAN_POINT ( 'NONE',  ( 94.99999999999995737, 1.387778780781445676E-14, 34.79898987322334136 ) ) ;
#8725=DIRECTION ( 'NONE',  ( -1.000000000000000000, 0.000000000000000000, 0.000000000000000000 ) ) ;
#8726=CARTESIAN_POINT ( 'NONE',  ( 95.54126587499996504, 1.387778780781445676E-14, 13.68750000136559386 ) ) ;
#8732=DIRECTION ( 'NONE',  ( -0.000000000000000000, -0.000000000000000000, -1.000000000000000000 ) ) ;
#8742=CARTESIAN_POINT ( 'NONE',  ( 103.1528011352953342, 3.152801135295383084, 12.31250000136559208 ) ) ;
#8755=CARTESIAN_POINT ( 'NONE',  ( 104.9999999999999716, 1.449011120738813565E-14, 3.625000002731184612 ) ) ;
#8762=FACE_BOUND ( 'NONE', #20039, .T. ) ;
#8764=CYLINDRICAL_SURFACE ( 'NONE', #6751, 5.000000000000004441 ) ;
#8772=CARTESIAN_POINT ( 'NONE',  ( 99.99999999999995737, 4.458734125000016313, 7.187500001365592084 ) ) ;
#8775=CARTESIAN_POINT ( 'NONE',  ( 99.99999999999995737, -4.458734124999988779, 10.68750000136559208 ) ) ;
#8777=AXIS2_PLACEMENT_3D ( 'NONE', #24611, #2805, #5373 ) ;
#8789=ORIENTED_EDGE ( 'NONE', *, *, #7373, .F. ) ;
#8797=( BOUNDED_CURVE ( )  B_SPLINE_CURVE ( 2, ( #20953, #9963, #18675, #3150, #11958, #27376, #11817, #20680, #9829 ),
 .UNSPECIFIED., .F., .F. ) 
 B_SPLINE_CURVE_WITH_KNOTS ( ( 3, 2, 2, 2, 3 ),
 ( 0.9285714285714284921, 0.9374999999999998890, 0.9464285714285712858, 0.9553571428571427937, 0.9642857142857141906 ),
 .UNSPECIFIED. ) 
 CURVE ( )  GEOMETRIC_REPRESENTATION_ITEM ( )  RATIONAL_B_SPLINE_CURVE ( ( 1.000000000000000888, 0.9238795325112857393, 1.000000000000000000, 0.9238795325112867385, 1.000000000000000000, 0.9238795325112867385, 1.000000000000000000, 0.9238795325112877377, 0.9999999999999990008 ) ) 
 REPRESENTATION_ITEM ( '' )  );
#8799=CARTESIAN_POINT ( 'NONE',  ( 96.46446609406721961, -3.535533905932727539, 5.124999999999999112 ) ) ;
#8805=ORIENTED_EDGE ( 'NONE', *, *, #5209, .T. ) ;
#8818=CARTESIAN_POINT ( 'NONE',  ( 101.8468681455907046, -4.458734124999987891, 2.750000001365592528 ) ) ;
#8836=CARTESIAN_POINT ( 'NONE',  ( 99.99999999999995737, -4.458734124999988779, 3.937500001365591640 ) ) ;
#8849=CARTESIAN_POINT ( 'NONE',  ( 104.4587341249999639, 1.442382525525748735E-14, 12.18750000136559208 ) ) ;
#8852=CARTESIAN_POINT ( 'NONE',  ( 95.54126587499996504, 1.387778780781445676E-14, 0.4375000013655920839 ) ) ;
#8866=DIRECTION ( 'NONE',  ( -0.000000000000000000, -0.000000000000000000, -1.000000000000000000 ) ) ;
#8868=EDGE_LOOP ( 'NONE', ( #17289, #2152, #3856, #18967 ) ) ;
#8884=CARTESIAN_POINT ( 'NONE',  ( 99.99999999999995737, 4.458734125000016313, 10.43750000136559208 ) ) ;
#8892=CARTESIAN_POINT ( 'NONE',  ( 99.99999999999995737, -4.999999999999990230, 12.25000000000000000 ) ) ;
#8898=VECTOR ( 'NONE', #8732, 1000.000000000000000 ) ;
#8909=CARTESIAN_POINT ( 'NONE',  ( 104.9999999999999716, 1.449011120738813565E-14, 10.49999999999999822 ) ) ;
#8915=CARTESIAN_POINT ( 'NONE',  ( 96.84719886470459471, 3.152801135295383084, 9.312500001365593860 ) ) ;
#8918=CARTESIAN_POINT ( 'NONE',  ( 103.1528011352953342, -3.152801135295355106, 12.81250000136559208 ) ) ;
#8940=CARTESIAN_POINT ( 'NONE',  ( 94.99999999999995737, 2.071067811865491048, 2.937499999999999112 ) ) ;
#8961=CARTESIAN_POINT ( 'NONE',  ( 95.54126587499996504, 1.387778780781445676E-14, 3.437500001365592972 ) ) ;
#8978=CARTESIAN_POINT ( 'NONE',  ( 104.4587341249999781, 1.846868145590750299, 4.250000001365592084 ) ) ;
#8986=PRODUCT_DEFINITION_SHAPE ( 'NONE', 'NONE',  #2652 ) ;
#8994=CARTESIAN_POINT ( 'NONE',  ( 101.8468681455906903, 4.458734125000016313, 10.37500000136559208 ) ) ;
#8995=CARTESIAN_POINT ( 'NONE',  ( 104.9999999999999716, 1.449011120738813565E-14, 34.79898987322334136 ) ) ;
#8996=CARTESIAN_POINT ( 'NONE',  ( 104.4587341249999639, 1.442382525525748735E-14, 12.93750000136559208 ) ) ;
#9004=EDGE_CURVE ( 'NONE', #162, #5815, #13064, .T. ) ;
#9014=CARTESIAN_POINT ( 'NONE',  ( 103.1528011352953342, -3.152801135295355106, 13.06250000136559208 ) ) ;
#9022=( GEOMETRIC_REPRESENTATION_CONTEXT ( 3 ) GLOBAL_UNCERTAINTY_ASSIGNED_CONTEXT ( ( #25449 ) ) GLOBAL_UNIT_ASSIGNED_CONTEXT ( ( #27860, #21159, #10450 ) ) REPRESENTATION_CONTEXT ( 'NONE', 'WORKASPACE' ) );
#9032=CARTESIAN_POINT ( 'NONE',  ( 95.54126587499996504, 1.846868145590750077, 12.62500000136559208 ) ) ;
#9041=ORIENTED_EDGE ( 'NONE', *, *, #5070, .T. ) ;
#9052=( BOUNDED_CURVE ( )  B_SPLINE_CURVE ( 2, ( #15752, #6917, #15610, #20722, #24312, #24455, #5331, #13996, #1204 ),
 .UNSPECIFIED., .F., .F. ) 
 B_SPLINE_CURVE_WITH_KNOTS ( ( 3, 2, 2, 2, 3 ),
 ( 0.5000000000000000000, 0.5089285714285713969, 0.5178571428571429047, 0.5267857142857143016, 0.5357142857142856984 ),
 .UNSPECIFIED. ) 
 CURVE ( )  GEOMETRIC_REPRESENTATION_ITEM ( )  RATIONAL_B_SPLINE_CURVE ( ( 1.000000000000000000, 0.9238795325112867385, 1.000000000000000000, 0.9238795325112867385, 1.000000000000000000, 0.9238795325112867385, 1.000000000000000000, 0.9238795325112867385, 1.000000000000000000 ) ) 
 REPRESENTATION_ITEM ( '' )  );
#9056=CARTESIAN_POINT ( 'NONE',  ( 94.99999999999995737, -2.071067811865466624, 2.187500002731185056 ) ) ;
#9059=CARTESIAN_POINT ( 'NONE',  ( 96.84719886470459471, -3.152801135295355994, 9.562500001365593860 ) ) ;
#9062=CARTESIAN_POINT ( 'NONE',  ( 98.15313185440925281, -4.458734124999987891, 7.625000001365592084 ) ) ;
#9075=CARTESIAN_POINT ( 'NONE',  ( 97.92893218813451028, -4.999999999999989342, 8.187500000000000000 ) ) ;
#9078=CARTESIAN_POINT ( 'NONE',  ( 103.5355339059327093, -3.535533905932726206, 9.500000002731184168 ) ) ;
#9101=CARTESIAN_POINT ( 'NONE',  ( 95.54126587499996504, 1.387778780781445676E-14, 0.6875000013655923059 ) ) ;
#9104=CARTESIAN_POINT ( 'NONE',  ( 103.1528011352953342, 3.152801135295383084, 2.062500001365591640 ) ) ;
#9120=CARTESIAN_POINT ( 'NONE',  ( 96.84719886470459471, -3.152801135295355994, 0.8125000013655924169 ) ) ;
#9130=FACE_OUTER_BOUND ( 'NONE', #16005, .T. ) ;
#9133=CARTESIAN_POINT ( 'NONE',  ( 103.1528011352953342, -3.152801135295355106, 13.06250000136559208 ) ) ;
#9136=CARTESIAN_POINT ( 'NONE',  ( 104.4587341249999639, 1.442382525525748735E-14, 1.937500001365591640 ) ) ;
#9143=ORIENTED_EDGE ( 'NONE', *, *, #6712, .T. ) ;
#9153=CARTESIAN_POINT ( 'NONE',  ( 98.15313185440925281, -4.458734124999987891, 9.875000001365593860 ) ) ;
#9171=CARTESIAN_POINT ( 'NONE',  ( 95.54126587499996504, 1.846868145590750077, 11.62500000136559031 ) ) ;
#9174=CARTESIAN_POINT ( 'NONE',  ( 99.99999999999995737, -4.999999999999990230, 2.249999999999998668 ) ) ;
#9191=EDGE_CURVE ( 'NONE', #15219, #3701, #3290, .T. ) ;
#9198=CARTESIAN_POINT ( 'NONE',  ( 95.54126587499996504, 1.387778780781445676E-14, 3.437500001365592972 ) ) ;
#9201=CARTESIAN_POINT ( 'NONE',  ( 95.54126587499996504, 1.387778780781445676E-14, 7.437500001365592084 ) ) ;
#9220=CARTESIAN_POINT ( 'NONE',  ( 102.0710678118654329, 5.000000000000018652, 8.812500002731182391 ) ) ;
#9234=CARTESIAN_POINT ( 'NONE',  ( 94.99999999999995737, 1.387778780781445676E-14, 10.12500000273118594 ) ) ;
#9260=CARTESIAN_POINT ( 'NONE',  ( 102.0710678118654329, 5.000000000000018652, 13.68750000000000000 ) ) ;
#9273=CARTESIAN_POINT ( 'NONE',  ( 104.4587341249999781, 1.846868145590750299, 12.25000000136559208 ) ) ;
#9276=CARTESIAN_POINT ( 'NONE',  ( 101.8468681455907046, 4.458734125000016313, 14.12500000136559208 ) ) ;
#9281=VERTEX_POINT ( 'NONE', #20789 ) ;
#9288=CARTESIAN_POINT ( 'NONE',  ( 98.15313185440925281, -4.458734124999987891, 12.87500000136559208 ) ) ;
#9305=CARTESIAN_POINT ( 'NONE',  ( 101.8468681455907046, -4.458734124999987891, 9.000000001365592084 ) ) ;
#9306=EDGE_CURVE ( 'NONE', #3132, #24544, #15999, .T. ) ;
#9323=ORIENTED_EDGE ( 'NONE', *, *, #80, .F. ) ;
#9324=CARTESIAN_POINT ( 'NONE',  ( 94.99999999999995737, 1.387778780781445676E-14, 13.00000000000000000 ) ) ;
#9335=CARTESIAN_POINT ( 'NONE',  ( 96.84719886470459471, 3.152801135295383084, 5.312500001365592972 ) ) ;
#9338=CARTESIAN_POINT ( 'NONE',  ( 104.4587341249999781, -1.846868145590721655, 9.875000001365593860 ) ) ;
#9349=AXIS2_PLACEMENT_3D ( 'NONE', #3723, #21243, #23381 ) ;
#9357=CARTESIAN_POINT ( 'NONE',  ( 99.99999999999995737, -4.999999999999990230, 11.37500000273118594 ) ) ;
#9362=CARTESIAN_POINT ( 'NONE',  ( 97.92893218813451028, -4.999999999999989342, 2.187499999999998224 ) ) ;
#9370=DIRECTION ( 'NONE',  ( -0.000000000000000000, -0.000000000000000000, -1.000000000000000000 ) ) ;
#9397=CARTESIAN_POINT ( 'NONE',  ( 104.9999999999999574, -2.071067811865462627, 11.43750000000000000 ) ) ;
#9403=CARTESIAN_POINT ( 'NONE',  ( 104.9999999999999716, 1.449011120738813565E-14, 11.50000000000000000 ) ) ;
#9412=CARTESIAN_POINT ( 'NONE',  ( 96.84719886470459471, -3.152801135295355994, 8.812500001365592084 ) ) ;
#9414=CARTESIAN_POINT ( 'NONE',  ( 104.4587341249999639, 1.442382525525748735E-14, 10.93750000136559208 ) ) ;
#9421=CARTESIAN_POINT ( 'NONE',  ( 94.99999999999995737, 1.387778780781445676E-14, 13.12500000273118417 ) ) ;
#9427=CARTESIAN_POINT ( 'NONE',  ( 101.8468681455906903, -4.458734124999987891, 12.00000000136559208 ) ) ;
#9446=CARTESIAN_POINT ( 'NONE',  ( 95.54126587499996504, 1.387778780781445676E-14, 7.687500001365592084 ) ) ;
#9463=ORIENTED_EDGE ( 'NONE', *, *, #8241, .F. ) ;
#9472=CARTESIAN_POINT ( 'NONE',  ( 99.99999999999995737, 1.387778780781445676E-14, 34.79898987322334136 ) ) ;
#9475=CARTESIAN_POINT ( 'NONE',  ( 104.4587341249999781, 1.846868145590750299, 4.000000001365592084 ) ) ;
#9476=ORIENTED_EDGE ( 'NONE', *, *, #16974, .T. ) ;
#9478=CARTESIAN_POINT ( 'NONE',  ( 96.84719886470459471, 3.152801135295383084, 6.312500001365592084 ) ) ;
#9491=ORIENTED_EDGE ( 'NONE', *, *, #17393, .F. ) ;
#9496=CARTESIAN_POINT ( 'NONE',  ( 97.92893218813451028, 5.000000000000018652, 7.937500002731185056 ) ) ;
#9504=CARTESIAN_POINT ( 'NONE',  ( 96.46446609406721961, -3.535533905932727539, 1.124999999999999334 ) ) ;
#9516=DIRECTION ( 'NONE',  ( 1.000000000000000000, 0.000000000000000000, 0.000000000000000000 ) ) ;
#9529=VERTEX_POINT ( 'NONE', #6364 ) ;
#9544=CYLINDRICAL_SURFACE ( 'NONE', #18156, 5.000000000000004441 ) ;
#9545=CARTESIAN_POINT ( 'NONE',  ( 96.46446609406721961, -3.535533905932727539, 13.12500000000000000 ) ) ;
#9551=CARTESIAN_POINT ( 'NONE',  ( 99.99999999999995737, 5.000000000000018652, 13.87500000273118594 ) ) ;
#9558=CARTESIAN_POINT ( 'NONE',  ( 99.99999999999995737, -4.458734124999988779, 5.937500001365592084 ) ) ;
#9560=CARTESIAN_POINT ( 'NONE',  ( 104.4587341249999639, 1.442382525525748735E-14, 8.937500001365592084 ) ) ;
#9563=DIRECTION ( 'NONE',  ( -0.000000000000000000, -0.000000000000000000, -1.000000000000000000 ) ) ;
#9573=CARTESIAN_POINT ( 'NONE',  ( 103.1528011352953342, 3.152801135295383084, 10.31250000136559208 ) ) ;
#9589=CARTESIAN_POINT ( 'NONE',  ( 98.15313185440923860, 4.458734125000016313, 7.500000001365592084 ) ) ;
#9592=CARTESIAN_POINT ( 'NONE',  ( 96.46446609406721961, -3.535533905932727539, 2.124999999999998224 ) ) ;
#9610=CARTESIAN_POINT ( 'NONE',  ( 97.92893218813451028, 5.000000000000018652, 8.937500002731184168 ) ) ;
#9611=CARTESIAN_POINT ( 'NONE',  ( 97.92893218813451028, -4.999999999999989342, 1.312500002731184612 ) ) ;
#9615=CARTESIAN_POINT ( 'NONE',  ( 99.99999999999995737, 1.387778780781445676E-14, 34.79898987322334136 ) ) ;
#9619=CARTESIAN_POINT ( 'NONE',  ( 104.4587341249999781, -1.846868145590721655, 4.875000001365592084 ) ) ;
#9622=CARTESIAN_POINT ( 'NONE',  ( 96.84719886470459471, -3.152801135295355994, 7.562500001365592084 ) ) ;
#9633=VERTEX_POINT ( 'NONE', #12758 ) ;
#9639=CARTESIAN_POINT ( 'NONE',  ( 99.99999999999995737, 5.000000000000018652, 7.875000002731185056 ) ) ;
#9642=CARTESIAN_POINT ( 'NONE',  ( 99.99999999999995737, 5.000000000000018652, 14.75000000000000000 ) ) ;
#9686=CARTESIAN_POINT ( 'NONE',  ( 96.46446609406721961, -3.535533905932727539, 14.12499999999999822 ) ) ;
#9688=ORIENTED_EDGE ( 'NONE', *, *, #10913, .T. ) ;
#9693=CARTESIAN_POINT ( 'NONE',  ( 103.5355339059327093, -3.535533905932726206, 13.50000000273118417 ) ) ;
#9701=CARTESIAN_POINT ( 'NONE',  ( 99.99999999999995737, 4.458734125000016313, 7.437500001365592084 ) ) ;
#9703=CARTESIAN_POINT ( 'NONE',  ( 101.8468681455907046, -4.458734124999987891, 11.75000000136559208 ) ) ;
#9717=CARTESIAN_POINT ( 'NONE',  ( 101.8468681455906903, 4.458734125000016313, 12.37500000136559208 ) ) ;
#9731=CARTESIAN_POINT ( 'NONE',  ( 103.1528011352953342, 3.152801135295383084, 5.312500001365592972 ) ) ;
#9745=CARTESIAN_POINT ( 'NONE',  ( 104.9999999999999716, 1.449011120738813565E-14, 0.6250000027311856110 ) ) ;
#9746=CYLINDRICAL_SURFACE ( 'NONE', #1877, 5.000000000000004441 ) ;
#9753=CARTESIAN_POINT ( 'NONE',  ( 99.99999999999995737, -4.999999999999990230, 7.249999999999999112 ) ) ;
#9759=CARTESIAN_POINT ( 'NONE',  ( 99.99999999999995737, -4.458734124999988779, 4.687500001365592084 ) ) ;
#9760=CARTESIAN_POINT ( 'NONE',  ( 103.5355339059327093, 3.535533905932755072, 12.75000000273118594 ) ) ;
#9761=CARTESIAN_POINT ( 'NONE',  ( 96.84719886470459471, 3.152801135295383084, 3.312500001365592972 ) ) ;
#9765=CARTESIAN_POINT ( 'NONE',  ( 94.99999999999995737, 1.387778780781445676E-14, 4.999999999999999112 ) ) ;
#9778=CARTESIAN_POINT ( 'NONE',  ( 104.9999999999999574, 2.071067811865491937, 6.687500002731185056 ) ) ;
#9788=VECTOR ( 'NONE', #16310, 1000.000000000000000 ) ;
#9813=ORIENTED_EDGE ( 'NONE', *, *, #14399, .F. ) ;
#9823=CARTESIAN_POINT ( 'NONE',  ( 104.9999999999999716, 1.449011120738813565E-14, 7.500000000000000000 ) ) ;
#9829=CARTESIAN_POINT ( 'NONE',  ( 104.9999999999999716, 1.449011120738813565E-14, 0.6250000027311856110 ) ) ;
#9830=CARTESIAN_POINT ( 'NONE',  ( 104.9999999999999716, 1.449011120738813565E-14, 3.499999999999999556 ) ) ;
#9831=EDGE_CURVE ( 'NONE', #25528, #3896, #9052, .T. ) ;
#9832=CARTESIAN_POINT ( 'NONE',  ( 102.0710678118654329, 5.000000000000018652, 11.81250000273118950 ) ) ;
#9837=CARTESIAN_POINT ( 'NONE',  ( 104.4587341249999781, -1.846868145590721655, 6.125000001365591196 ) ) ;
#9839=CARTESIAN_POINT ( 'NONE',  ( 103.1528011352953342, 3.152801135295383084, 11.06250000136559208 ) ) ;
#9855=CARTESIAN_POINT ( 'NONE',  ( 98.15313185440925281, -4.458734124999987891, 7.875000001365591196 ) ) ;
#9856=EDGE_CURVE ( 'NONE', #23574, #26438, #11956, .T. ) ;
#9857=VERTEX_POINT ( 'NONE', #8013 ) ;
#9870=CARTESIAN_POINT ( 'NONE',  ( 95.54126587499996504, -1.846868145590724986, 7.750000001365592084 ) ) ;
#9884=DIRECTION ( 'NONE',  ( -1.000000000000000000, 0.000000000000000000, 0.000000000000000000 ) ) ;
#9888=CARTESIAN_POINT ( 'NONE',  ( 94.99999999999995737, 1.387778780781445676E-14, 9.125000002731184168 ) ) ;
#9896=CARTESIAN_POINT ( 'NONE',  ( 95.54126587499995082, 1.846868145590750077, 2.375000001365592084 ) ) ;
#9906=ORIENTED_EDGE ( 'NONE', *, *, #16925, .T. ) ;
#9910=CARTESIAN_POINT ( 'NONE',  ( 104.9999999999999716, 1.449011120738813565E-14, 7.625000002731185056 ) ) ;
#9926=CARTESIAN_POINT ( 'NONE',  ( 95.54126587499995082, 1.846868145590750077, 11.37500000136559208 ) ) ;
#9945=CARTESIAN_POINT ( 'NONE',  ( 96.46446609406721961, 3.535533905932755072, 7.875000000000000000 ) ) ;
#9952=AXIS2_PLACEMENT_3D ( 'NONE', #25224, #5846, #7553 ) ;
#9954=AXIS2_PLACEMENT_3D ( 'NONE', #13954, #24525, #20247 ) ;
#9957=CARTESIAN_POINT ( 'NONE',  ( 94.99999999999995737, 1.387778780781445676E-14, 11.00000000000000000 ) ) ;
#9963=CARTESIAN_POINT ( 'NONE',  ( 94.99999999999997158, 2.071067811865471953, 1.062500002731186832 ) ) ;
#9964=FACE_OUTER_BOUND ( 'NONE', #1731, .T. ) ;
#9970=CARTESIAN_POINT ( 'NONE',  ( 104.9999999999999716, 1.449011120738813565E-14, 9.500000000000000000 ) ) ;
#9971=CARTESIAN_POINT ( 'NONE',  ( 103.1528011352953342, 3.152801135295383084, 6.312500001365592084 ) ) ;
#9973=CARTESIAN_POINT ( 'NONE',  ( 95.54126587499996504, 1.387778780781445676E-14, 9.437500001365593860 ) ) ;
#9988=CARTESIAN_POINT ( 'NONE',  ( 101.8468681455906903, 4.458734125000016313, 5.375000001365592972 ) ) ;
#10002=CARTESIAN_POINT ( 'NONE',  ( 104.4587341249999781, 1.846868145590750521, 2.250000001365592084 ) ) ;
#10013=CARTESIAN_POINT ( 'NONE',  ( 104.9999999999999716, 1.449011120738813565E-14, 34.79898987322334136 ) ) ;
#10031=CARTESIAN_POINT ( 'NONE',  ( 95.54126587499995082, -1.846868145590724986, 1.500000001365591418 ) ) ;
#10032=CARTESIAN_POINT ( 'NONE',  ( 95.54126587499996504, 1.846868145590750077, 14.62500000136559208 ) ) ;
#10048=CARTESIAN_POINT ( 'NONE',  ( 94.99999999999995737, 2.071067811865491048, 7.062500002731185944 ) ) ;
#10063=CARTESIAN_POINT ( 'NONE',  ( 96.84719886470459471, -3.152801135295355994, 12.56250000136559208 ) ) ;
#10064=CARTESIAN_POINT ( 'NONE',  ( 94.99999999999995737, 1.387778780781445676E-14, 13.12500000273118417 ) ) ;
#10065=ORIENTED_EDGE ( 'NONE', *, *, #12967, .T. ) ;
#10087=ORIENTED_EDGE ( 'NONE', *, *, #25360, .F. ) ;
#10088=CARTESIAN_POINT ( 'NONE',  ( 104.9999999999999574, 2.071067811865491937, 7.562499999999999112 ) ) ;
#10093=CARTESIAN_POINT ( 'NONE',  ( 97.92893218813451028, 5.000000000000018652, 13.93750000273118772 ) ) ;
#10103=CARTESIAN_POINT ( 'NONE',  ( 96.84719886470459471, -3.152801135295355994, 4.812500001365592084 ) ) ;
#10104=CARTESIAN_POINT ( 'NONE',  ( 103.1528011352953342, 3.152801135295383084, 7.062500001365592084 ) ) ;
#10117=CARTESIAN_POINT ( 'NONE',  ( 95.54126587499995082, -1.846868145590724986, 5.750000001365591196 ) ) ;
#10118=ORIENTED_EDGE ( 'NONE', *, *, #6887, .T. ) ;
#10132=CARTESIAN_POINT ( 'NONE',  ( 101.8468681455907046, -4.458734124999987891, 3.000000001365592528 ) ) ;
#10141=CARTESIAN_POINT ( 'NONE',  ( 95.27063293749995410, 1.387778780781445676E-14, 0.8437500006827957089 ) ) ;
#10143=DIRECTION ( 'NONE',  ( -0.000000000000000000, -0.000000000000000000, -1.000000000000000000 ) ) ;
#10157=FACE_OUTER_BOUND ( 'NONE', #25274, .T. ) ;
#10159=VERTEX_POINT ( 'NONE', #19481 ) ;
#10165=EDGE_CURVE ( 'NONE', #9633, #25436, #17685, .T. ) ;
#10177=CARTESIAN_POINT ( 'NONE',  ( 104.9999999999999716, 1.449011120738813565E-14, 6.625000002731185944 ) ) ;
#10194=EDGE_CURVE ( 'NONE', #18726, #17053, #22602, .T. ) ;
#10196=CARTESIAN_POINT ( 'NONE',  ( 99.99999999999995737, -4.458734124999988779, 13.68750000136559208 ) ) ;
#10200=( BOUNDED_CURVE ( )  B_SPLINE_CURVE ( 2, ( #19559, #2464, #14985, #13255, #2042, #10711, #21986, #6580, #21710 ),
 .UNSPECIFIED., .F., .F. ) 
 B_SPLINE_CURVE_WITH_KNOTS ( ( 3, 2, 2, 2, 3 ),
 ( 0.4642857142857142461, 0.4732142857142856429, 0.4821428571428570953, 0.4910714285714285476, 0.5000000000000000000 ),
 .UNSPECIFIED. ) 
 CURVE ( )  GEOMETRIC_REPRESENTATION_ITEM ( )  RATIONAL_B_SPLINE_CURVE ( ( 1.000000000000000444, 0.9238795325112862944, 1.000000000000000000, 0.9238795325112867385, 1.000000000000000000, 0.9238795325112867385, 1.000000000000000000, 0.9238795325112867385, 1.000000000000000000 ) ) 
 REPRESENTATION_ITEM ( '' )  );
#10214=ORIENTED_EDGE ( 'NONE', *, *, #19041, .F. ) ;
#10224=CARTESIAN_POINT ( 'NONE',  ( 94.99999999999995737, 2.071067811865491048, 10.93749999999999822 ) ) ;
#10238=FACE_OUTER_BOUND ( 'NONE', #23359, .T. ) ;
#10239=CARTESIAN_POINT ( 'NONE',  ( 99.99999999999995737, 4.458734125000016313, 1.437500001365592972 ) ) ;
#10242=CARTESIAN_POINT ( 'NONE',  ( 95.54126587499996504, 1.846868145590750077, 4.375000001365592084 ) ) ;
#10256=CARTESIAN_POINT ( 'NONE',  ( 95.54126587499995082, -1.846868145590724986, 6.750000001365592972 ) ) ;
#10271=CARTESIAN_POINT ( 'NONE',  ( 104.4587341249999639, 1.442382525525748735E-14, 4.937500001365592972 ) ) ;
#10273=CARTESIAN_POINT ( 'NONE',  ( 104.4587341249999639, 1.442382525525748735E-14, 2.187500001365592084 ) ) ;
#10283=CARTESIAN_POINT ( 'NONE',  ( 99.99999999999995737, -4.999999999999990230, 3.375000002731184612 ) ) ;
#10293=LINE ( 'NONE', #25427, #9788 ) ;
#10303=CARTESIAN_POINT ( 'NONE',  ( 95.54126587499996504, 1.846868145590750077, 13.62500000136559386 ) ) ;
#10312=ORIENTED_EDGE ( 'NONE', *, *, #27597, .T. ) ;
#10316=CARTESIAN_POINT ( 'NONE',  ( 104.9999999999999716, 1.449011120738813565E-14, 5.625000002731185056 ) ) ;
#10324=DIRECTION ( 'NONE',  ( -1.000000000000000000, 0.000000000000000000, 0.000000000000000000 ) ) ;
#10335=CARTESIAN_POINT ( 'NONE',  ( 104.4587341249999781, 1.846868145590750299, 13.00000000136559386 ) ) ;
#10365=CARTESIAN_POINT ( 'NONE',  ( 102.0710678118654329, 5.000000000000018652, 3.687499999999999556 ) ) ;
#10380=CARTESIAN_POINT ( 'NONE',  ( 94.99999999999995737, 1.387778780781445676E-14, 8.125000002731185944 ) ) ;
#10381=CARTESIAN_POINT ( 'NONE',  ( 95.54126587499996504, 1.387778780781445676E-14, 2.687500001365592528 ) ) ;
#10383=CARTESIAN_POINT ( 'NONE',  ( 98.15313185440923860, -4.458734124999987891, 4.625000001365592084 ) ) ;
#10402=CARTESIAN_POINT ( 'NONE',  ( 103.1528011352953342, 3.152801135295383084, 5.312500001365592972 ) ) ;
#10412=EDGE_LOOP ( 'NONE', ( #26229, #15584, #11241, #14538 ) ) ;
#10418=CARTESIAN_POINT ( 'NONE',  ( 98.15313185440925281, 4.458734125000016313, 5.250000001365592972 ) ) ;
#10420=CARTESIAN_POINT ( 'NONE',  ( 103.1528011352953342, 3.152801135295383084, 4.312500001365592084 ) ) ;
#10424=ORIENTED_EDGE ( 'NONE', *, *, #14399, .T. ) ;
#10430=CARTESIAN_POINT ( 'NONE',  ( 102.0710678118654329, -4.999999999999989342, 6.437500002731185944 ) ) ;
#10444=CYLINDRICAL_SURFACE ( 'NONE', #24625, 5.000000000000004441 ) ;
#10447=EDGE_CURVE ( 'NONE', #4790, #4419, #18752, .T. ) ;
#10450=( NAMED_UNIT ( * ) SI_UNIT ( $, .STERADIAN. ) SOLID_ANGLE_UNIT ( ) );
#10451=CARTESIAN_POINT ( 'NONE',  ( 104.4587341249999639, 1.442382525525748735E-14, 14.18750000136559208 ) ) ;
#10456=FACE_OUTER_BOUND ( 'NONE', #11088, .T. ) ;
#10457=CARTESIAN_POINT ( 'NONE',  ( 94.99999999999995737, 1.387778780781445676E-14, 5.999999999999998224 ) ) ;
#10463=CARTESIAN_POINT ( 'NONE',  ( 102.0710678118654329, 5.000000000000018652, 1.812500002731185278 ) ) ;
#10469=CARTESIAN_POINT ( 'NONE',  ( 97.92893218813451028, -4.999999999999989342, 9.312500002731184168 ) ) ;
#10470=LINE ( 'NONE', #4355, #23518 ) ;
#10480=CARTESIAN_POINT ( 'NONE',  ( 104.4587341249999781, -1.846868145590721655, 10.87500000136559386 ) ) ;
#10485=CARTESIAN_POINT ( 'NONE',  ( 103.5355339059327093, 3.535533905932755072, 8.624999999999998224 ) ) ;
#10492=CARTESIAN_POINT ( 'NONE',  ( 102.0710678118654329, 5.000000000000018652, 11.68750000000000000 ) ) ;
#10508=CARTESIAN_POINT ( 'NONE',  ( 104.9999999999999574, 2.071067811865491937, 4.562500000000000000 ) ) ;
#10515=CARTESIAN_POINT ( 'NONE',  ( 94.99999999999995737, 2.071067811865491493, 6.937499999999999112 ) ) ;
#10523=CARTESIAN_POINT ( 'NONE',  ( 104.4587341249999781, 1.846868145590750299, 3.250000001365592528 ) ) ;
#10526=CARTESIAN_POINT ( 'NONE',  ( 104.4587341249999781, -1.846868145590721655, 6.875000001365592972 ) ) ;
#10541=CARTESIAN_POINT ( 'NONE',  ( 104.4587341249999781, 1.846868145590750299, 1.250000001365592750 ) ) ;
#10555=EDGE_CURVE ( 'NONE', #7171, #4924, #18880, .T. ) ;
#10556=CARTESIAN_POINT ( 'NONE',  ( 101.8468681455906903, -4.458734124999987891, 0.7500000013655925279 ) ) ;
#10558=CARTESIAN_POINT ( 'NONE',  ( 104.4587341249999639, 1.442382525525748735E-14, 5.937500001365592084 ) ) ;
#10561=CARTESIAN_POINT ( 'NONE',  ( 104.4587341249999781, -1.846868145590721655, 3.125000001365592528 ) ) ;
#10570=CARTESIAN_POINT ( 'NONE',  ( 104.9999999999999574, 2.071067811865511032, 5.562500000000000888 ) ) ;
#10576=DIRECTION ( 'NONE',  ( -0.000000000000000000, -0.000000000000000000, -1.000000000000000000 ) ) ;
#10597=CARTESIAN_POINT ( 'NONE',  ( 99.99999999999995737, 1.387778780781445676E-14, 34.79898987322334136 ) ) ;
#10605=CARTESIAN_POINT ( 'NONE',  ( 94.99999999999995737, 1.387778780781445676E-14, 0.1250000027311851669 ) ) ;
#10609=FACE_OUTER_BOUND ( 'NONE', #26507, .T. ) ;
#10619=CARTESIAN_POINT ( 'NONE',  ( 94.99999999999995737, 1.387778780781445676E-14, 34.79898987322334136 ) ) ;
#10620=CARTESIAN_POINT ( 'NONE',  ( 99.99999999999995737, -4.458734124999988779, 9.687500001365593860 ) ) ;
#10621=CARTESIAN_POINT ( 'NONE',  ( 99.99999999999995737, -4.999999999999990230, 13.37500000273118417 ) ) ;
#10624=CARTESIAN_POINT ( 'NONE',  ( 96.84719886470459471, 3.152801135295383084, 12.31250000136559208 ) ) ;
#10646=CARTESIAN_POINT ( 'NONE',  ( 104.9999999999999574, 2.071067811865491937, 6.562499999999998224 ) ) ;
#10647=CARTESIAN_POINT ( 'NONE',  ( 94.99999999999995737, 1.387778780781445676E-14, 1.999999999999998224 ) ) ;
#10659=CARTESIAN_POINT ( 'NONE',  ( 101.8468681455906903, 4.458734125000016313, 4.375000001365592084 ) ) ;
#10661=CARTESIAN_POINT ( 'NONE',  ( 101.8468681455907046, 4.458734125000016313, 7.125000001365592084 ) ) ;
#10676=CARTESIAN_POINT ( 'NONE',  ( 99.99999999999995737, -4.458734124999988779, 1.937500001365591640 ) ) ;
#10692=CARTESIAN_POINT ( 'NONE',  ( 96.84719886470459471, 3.152801135295383084, 1.312500001365592750 ) ) ;
#10694=CARTESIAN_POINT ( 'NONE',  ( 99.99999999999995737, -4.458734124999988779, 3.687500001365591640 ) ) ;
#10711=CARTESIAN_POINT ( 'NONE',  ( 97.92893218813451028, -4.999999999999989342, 7.312500002731185056 ) ) ;
#10724=EDGE_LOOP ( 'NONE', ( #17087, #23388, #24045, #8318 ) ) ;
#10728=SHAPE_REPRESENTATION_RELATIONSHIP ( 'NONE' , 'NONE' ,  #17883, #26371 ) ;
#10729=CARTESIAN_POINT ( 'NONE',  ( 98.15313185440923860, 4.458734125000016313, 10.50000000136559208 ) ) ;
#10735=CARTESIAN_POINT ( 'NONE',  ( 104.9999999999999716, 1.449011120738813565E-14, 12.49999999999999822 ) ) ;
#10741=CARTESIAN_POINT ( 'NONE',  ( 103.5355339059327093, 3.535533905932755072, 2.750000002731185944 ) ) ;
#10756=CARTESIAN_POINT ( 'NONE',  ( 99.99999999999995737, -4.999999999999990230, 10.24999999999999822 ) ) ;
#10757=CARTESIAN_POINT ( 'NONE',  ( 104.4587341249999781, -1.846868145590721655, 9.875000001365593860 ) ) ;
#10760=CARTESIAN_POINT ( 'NONE',  ( 101.8468681455906903, 4.458734125000016313, 12.12500000136559208 ) ) ;
#10770=CARTESIAN_POINT ( 'NONE',  ( 103.5355339059327093, -3.535533905932726206, 11.50000000273118417 ) ) ;
#10782=CARTESIAN_POINT ( 'NONE',  ( 96.46446609406721961, -3.535533905932727539, 7.124999999999999112 ) ) ;
#10788=CARTESIAN_POINT ( 'NONE',  ( 104.9999999999999716, 1.449011120738813565E-14, 4.625000002731185944 ) ) ;
#10798=EDGE_CURVE ( 'NONE', #10159, #25944, #16576, .T. ) ;
#10799=CARTESIAN_POINT ( 'NONE',  ( 96.84719886470459471, 3.152801135295383084, 1.312500001365592750 ) ) ;
#10813=CARTESIAN_POINT ( 'NONE',  ( 95.54126587499996504, 1.387778780781445676E-14, 2.687500001365592528 ) ) ;
#10828=CARTESIAN_POINT ( 'NONE',  ( 104.4587341249999639, 1.442382525525748735E-14, 10.18750000136559208 ) ) ;
#10830=CARTESIAN_POINT ( 'NONE',  ( 95.54126587499996504, -1.846868145590724986, 13.50000000136559386 ) ) ;
#10839=EDGE_CURVE ( 'NONE', #14819, #22694, #17739, .T. ) ;
#10846=CYLINDRICAL_SURFACE ( 'NONE', #26191, 5.000000000000004441 ) ;
#10847=AXIS2_PLACEMENT_3D ( 'NONE', #18314, #27023, #4927 ) ;
#10861=ORIENTED_EDGE ( 'NONE', *, *, #22564, .F. ) ;
#10865=CARTESIAN_POINT ( 'NONE',  ( 104.4587341249999781, -1.846868145590721655, 12.12500000136559208 ) ) ;
#10866=( BOUNDED_CURVE ( )  B_SPLINE_CURVE ( 2, ( #2424, #11084, #24354, #26360, #13506, #6818, #17372, #26068, #13358 ),
 .UNSPECIFIED., .F., .F. ) 
 B_SPLINE_CURVE_WITH_KNOTS ( ( 3, 2, 2, 2, 3 ),
 ( 0.7142857142857141906, 0.7232142857142855874, 0.7321428571428569843, 0.7410714285714286031, 0.7500000000000000000 ),
 .UNSPECIFIED. ) 
 CURVE ( )  GEOMETRIC_REPRESENTATION_ITEM ( )  RATIONAL_B_SPLINE_CURVE ( ( 1.000000000000000888, 0.9238795325112857393, 1.000000000000000000, 0.9238795325112867385, 1.000000000000000000, 0.9238795325112867385, 1.000000000000000000, 0.9238795325112867385, 1.000000000000000000 ) ) 
 REPRESENTATION_ITEM ( '' )  );
#10873=AXIS2_PLACEMENT_3D ( 'NONE', #16209, #14483, #24912 ) ;
#10878=EDGE_CURVE ( 'NONE', #12008, #26730, #20728, .T. ) ;
#10882=CARTESIAN_POINT ( 'NONE',  ( 104.9999999999999574, 2.071067811865491937, 1.687500002731185056 ) ) ;
#10888=SURFACE_STYLE_USAGE ( .BOTH. , #2224 ) ;
#10890=DIRECTION ( 'NONE',  ( -0.000000000000000000, -0.000000000000000000, -1.000000000000000000 ) ) ;
#10896=CARTESIAN_POINT ( 'NONE',  ( 96.46446609406721961, -3.535533905932727539, 10.12499999999999822 ) ) ;
#10898=CARTESIAN_POINT ( 'NONE',  ( 95.54126587499996504, 1.387778780781445676E-14, 9.437500001365593860 ) ) ;
#10901=CARTESIAN_POINT ( 'NONE',  ( 104.4587341249999781, -1.846868145590721655, 10.87500000136559386 ) ) ;
#10913=EDGE_CURVE ( 'NONE', #12008, #3132, #2036, .T. ) ;
#10921=AXIS2_PLACEMENT_3D ( 'NONE', #10597, #21166, #27728 ) ;
#10924=CARTESIAN_POINT ( 'NONE',  ( 96.46446609406721961, -3.535533905932727539, 6.124999999999998224 ) ) ;
#10938=CARTESIAN_POINT ( 'NONE',  ( 104.4587341249999781, 1.846868145590750521, 3.000000001365592528 ) ) ;
#10956=CARTESIAN_POINT ( 'NONE',  ( 99.99999999999995737, 4.458734125000016313, 2.437500001365592084 ) ) ;
#10969=CARTESIAN_POINT ( 'NONE',  ( 101.8468681455906903, 4.458734125000016313, 11.37500000136559386 ) ) ;
#10971=CARTESIAN_POINT ( 'NONE',  ( 95.54126587499996504, -1.846868145590724986, 12.50000000136559208 ) ) ;
#11000=ORIENTED_EDGE ( 'NONE', *, *, #19768, .F. ) ;
#11003=CARTESIAN_POINT ( 'NONE',  ( 98.15313185440923860, -4.458734124999987891, 10.87500000136559208 ) ) ;
#11021=CARTESIAN_POINT ( 'NONE',  ( 104.9999999999999716, 1.449011120738813565E-14, 12.49999999999999822 ) ) ;
#11035=CARTESIAN_POINT ( 'NONE',  ( 98.15313185440925281, -4.458734124999987891, 10.62500000136559208 ) ) ;
#11038=CARTESIAN_POINT ( 'NONE',  ( 101.8468681455906903, -4.458734124999987891, 13.75000000136559208 ) ) ;
#11052=EDGE_LOOP ( 'NONE', ( #502, #25173, #5678, #28090 ) ) ;
#11061=CARTESIAN_POINT ( 'NONE',  ( 96.46446609406721961, -3.535533905932727539, 3.124999999999999112 ) ) ;
#11071=CARTESIAN_POINT ( 'NONE',  ( 103.5355339059327093, 3.535533905932755072, 6.624999999999999112 ) ) ;
#11078=CARTESIAN_POINT ( 'NONE',  ( 95.54126587499995082, -1.846868145590724986, 0.7500000013655925279 ) ) ;
#11081=CARTESIAN_POINT ( 'NONE',  ( 96.84719886470459471, 3.152801135295383084, 3.312500001365592972 ) ) ;
#11084=CARTESIAN_POINT ( 'NONE',  ( 94.99999999999997158, 2.071067811865471953, 4.937500000000000000 ) ) ;
#11088=EDGE_LOOP ( 'NONE', ( #8193, #2327, #17952, #18279 ) ) ;
#11095=VERTEX_POINT ( 'NONE', #7270 ) ;
#11097=CARTESIAN_POINT ( 'NONE',  ( 99.99999999999995737, 4.458734125000016313, 1.437500001365592972 ) ) ;
#11110=CARTESIAN_POINT ( 'NONE',  ( 103.1528011352953342, -3.152801135295355106, 11.06250000136559208 ) ) ;
#11112=CARTESIAN_POINT ( 'NONE',  ( 101.8468681455906903, -4.458734124999987891, 1.750000001365591862 ) ) ;
#11119=ORIENTED_EDGE ( 'NONE', *, *, #1334, .F. ) ;
#11121=CARTESIAN_POINT ( 'NONE',  ( 104.9999999999999716, 1.449011120738813565E-14, 12.62500000273118594 ) ) ;
#11124=ORIENTED_EDGE ( 'NONE', *, *, #14556, .F. ) ;
#11127=CARTESIAN_POINT ( 'NONE',  ( 101.8468681455906903, 4.458734125000016313, 13.37500000136559386 ) ) ;
#11142=CARTESIAN_POINT ( 'NONE',  ( 99.99999999999995737, 4.458734125000016313, 9.437500001365593860 ) ) ;
#11162=CYLINDRICAL_SURFACE ( 'NONE', #4770, 5.000000000000004441 ) ;
#11172=CARTESIAN_POINT ( 'NONE',  ( 104.4587341249999781, -1.846868145590721655, 7.875000001365591196 ) ) ;
#11176=CARTESIAN_POINT ( 'NONE',  ( 104.4587341249999639, 1.442382525525748735E-14, 7.937500001365592084 ) ) ;
#11195=AXIS2_PLACEMENT_3D ( 'NONE', #442, #17819, #22387 ) ;
#11196=CARTESIAN_POINT ( 'NONE',  ( 104.9999999999999574, 2.071067811865491937, 7.687500002731185944 ) ) ;
#11203=CARTESIAN_POINT ( 'NONE',  ( 99.99999999999995737, -4.999999999999990230, 2.249999999999998668 ) ) ;
#11207=CARTESIAN_POINT ( 'NONE',  ( 102.0710678118654329, 5.000000000000018652, 5.812500002731185056 ) ) ;
#11209=CARTESIAN_POINT ( 'NONE',  ( 94.99999999999995737, -2.071067811865466624, 10.18750000273118417 ) ) ;
#11221=CARTESIAN_POINT ( 'NONE',  ( 103.1528011352953342, -3.152801135295355106, 3.812500001365591640 ) ) ;
#11228=VERTEX_POINT ( 'NONE', #9970 ) ;
#11239=CARTESIAN_POINT ( 'NONE',  ( 102.0710678118654329, 5.000000000000018652, 12.68749999999999822 ) ) ;
#11241=ORIENTED_EDGE ( 'NONE', *, *, #20642, .T. ) ;
#11254=CARTESIAN_POINT ( 'NONE',  ( 95.54126587499995082, 1.846868145590750077, 11.62500000136559031 ) ) ;
#11256=CARTESIAN_POINT ( 'NONE',  ( 95.54126587499996504, 1.387778780781445676E-14, 1.437500001365591196 ) ) ;
#11259=CARTESIAN_POINT ( 'NONE',  ( 104.9999999999999716, 1.449011120738813565E-14, 11.62500000273118417 ) ) ;
#11270=CYLINDRICAL_SURFACE ( 'NONE', #14441, 5.000000000000004441 ) ;
#11271=CARTESIAN_POINT ( 'NONE',  ( 104.4587341249999781, -1.846868145590721655, 10.12500000136559386 ) ) ;
#11284=ORIENTED_EDGE ( 'NONE', *, *, #6545, .T. ) ;
#11288=CARTESIAN_POINT ( 'NONE',  ( 101.8468681455907046, 4.458734125000016313, 12.37500000136559208 ) ) ;
#11305=ORIENTED_EDGE ( 'NONE', *, *, #21558, .F. ) ;
#11306=CARTESIAN_POINT ( 'NONE',  ( 99.99999999999995737, 5.000000000000018652, 10.87500000273118594 ) ) ;
#11308=CARTESIAN_POINT ( 'NONE',  ( 104.9999999999999716, 1.449011120738813565E-14, 5.625000002731185056 ) ) ;
#11312=CARTESIAN_POINT ( 'NONE',  ( 102.0710678118654329, 5.000000000000018652, 10.68749999999999822 ) ) ;
#11313=CYLINDRICAL_SURFACE ( 'NONE', #13218, 5.000000000000004441 ) ;
#11316=CARTESIAN_POINT ( 'NONE',  ( 101.8468681455906903, -4.458734124999987891, 5.750000001365591196 ) ) ;
#11319=CARTESIAN_POINT ( 'NONE',  ( 104.4587341249999781, -1.846868145590721655, 6.875000001365592972 ) ) ;
#11337=CARTESIAN_POINT ( 'NONE',  ( 104.9999999999999574, 2.071067811865491937, 9.687500002731184168 ) ) ;
#11340=CARTESIAN_POINT ( 'NONE',  ( 97.92893218813451028, 5.000000000000018652, 14.81249999999999822 ) ) ;
#11343=CARTESIAN_POINT ( 'NONE',  ( 94.99999999999995737, 1.387778780781445676E-14, 2.999999999999999112 ) ) ;
#11362=CARTESIAN_POINT ( 'NONE',  ( 104.4587341249999781, 1.846868145590750521, 2.000000001365591640 ) ) ;
#11376=ADVANCED_FACE ( 'NONE', ( #10238 ), #23512, .F. ) ;
#11382=CARTESIAN_POINT ( 'NONE',  ( 94.99999999999995737, -2.071067811865466624, 13.06250000000000000 ) ) ;
#11387=EDGE_CURVE ( 'NONE', #9857, #23574, #22429, .T. ) ;
#11397=CARTESIAN_POINT ( 'NONE',  ( 101.8468681455906903, -4.458734124999987891, 12.00000000136559208 ) ) ;
#11399=CARTESIAN_POINT ( 'NONE',  ( 95.54126587499996504, 1.387778780781445676E-14, 14.43750000136559208 ) ) ;
#11408=CARTESIAN_POINT ( 'NONE',  ( 97.92893218813451028, -4.999999999999989342, 1.187499999999999334 ) ) ;
#11413=CARTESIAN_POINT ( 'NONE',  ( 96.84719886470459471, 3.152801135295383084, 11.56250000136559208 ) ) ;
#11431=CARTESIAN_POINT ( 'NONE',  ( 95.54126587499996504, -1.846868145590724986, 8.750000001365592084 ) ) ;
#11455=CARTESIAN_POINT ( 'NONE',  ( 94.99999999999995737, 1.387778780781445676E-14, 6.999999999999999112 ) ) ;
#11459=CARTESIAN_POINT ( 'NONE',  ( 101.8468681455906903, 4.458734125000016313, 6.125000001365591196 ) ) ;
#11462=CARTESIAN_POINT ( 'NONE',  ( 95.54126587499996504, 1.387778780781445676E-14, 6.437500001365592084 ) ) ;
#11480=CARTESIAN_POINT ( 'NONE',  ( 97.92893218813451028, -4.999999999999989342, 10.31250000273118594 ) ) ;
#11489=CARTESIAN_POINT ( 'NONE',  ( 94.99999999999995737, 1.387778780781445676E-14, 13.00000000000000000 ) ) ;
#11493=( BOUNDED_CURVE ( )  B_SPLINE_CURVE ( 2, ( #9830, #13810, #7119, #24523, #24805, #1023, #5145, #15954, #27241 ),
 .UNSPECIFIED., .F., .F. ) 
 B_SPLINE_CURVE_WITH_KNOTS ( ( 3, 2, 2, 2, 3 ),
 ( 0.8214285714285713969, 0.8303571428571429047, 0.8392857142857143016, 0.8482142857142856984, 0.8571428571428570953 ),
 .UNSPECIFIED. ) 
 CURVE ( )  GEOMETRIC_REPRESENTATION_ITEM ( )  RATIONAL_B_SPLINE_CURVE ( ( 1.000000000000000000, 0.9238795325112867385, 1.000000000000000000, 0.9238795325112867385, 1.000000000000000000, 0.9238795325112867385, 1.000000000000000000, 0.9238795325112867385, 1.000000000000000000 ) ) 
 REPRESENTATION_ITEM ( '' )  );
#11521=CARTESIAN_POINT ( 'NONE',  ( 104.9999999999999716, 1.449011120738813565E-14, 13.50000000000000000 ) ) ;
#11535=CARTESIAN_POINT ( 'NONE',  ( 96.84719886470459471, 3.152801135295383084, 6.562500001365592084 ) ) ;
#11538=CARTESIAN_POINT ( 'NONE',  ( 96.84719886470459471, 3.152801135295383084, 8.312500001365592084 ) ) ;
#11548=CARTESIAN_POINT ( 'NONE',  ( 103.5355339059327093, -3.535533905932726206, 1.374999999999999556 ) ) ;
#11553=CARTESIAN_POINT ( 'NONE',  ( 99.99999999999995737, 4.458734125000016313, 10.43750000136559208 ) ) ;
#11566=EDGE_LOOP ( 'NONE', ( #24322, #13753, #16173, #7201 ) ) ;
#11570=CARTESIAN_POINT ( 'NONE',  ( 101.8468681455907046, 4.458734125000016313, 7.375000001365592084 ) ) ;
#11591=CARTESIAN_POINT ( 'NONE',  ( 94.99999999999997158, -2.071067811865486608, 5.187500002731184168 ) ) ;
#11594=CARTESIAN_POINT ( 'NONE',  ( 97.92893218813451028, -4.999999999999989342, 2.312500002731185500 ) ) ;
#11597=CARTESIAN_POINT ( 'NONE',  ( 104.4587341249999639, 1.442382525525748735E-14, 4.937500001365592972 ) ) ;
#11598=ORIENTED_EDGE ( 'NONE', *, *, #17878, .F. ) ;
#11599=CARTESIAN_POINT ( 'NONE',  ( 94.99999999999997158, 2.071067811865503483, 13.06250000273118239 ) ) ;
#11600=CARTESIAN_POINT ( 'NONE',  ( 96.84719886470459471, -3.152801135295355994, 6.562500001365592084 ) ) ;
#11618=CARTESIAN_POINT ( 'NONE',  ( 103.5355339059327093, -3.535533905932726206, 10.50000000273118594 ) ) ;
#11621=ADVANCED_FACE ( 'NONE', ( #7472 ), #11313, .F. ) ;
#11626=CARTESIAN_POINT ( 'NONE',  ( 96.46446609406721961, 3.535533905932755072, 1.875000000000000000 ) ) ;
#11657=AXIS2_PLACEMENT_3D ( 'NONE', #27569, #27427, #23291 ) ;
#11664=CARTESIAN_POINT ( 'NONE',  ( 94.99999999999995737, 1.387778780781445676E-14, 9.125000002731184168 ) ) ;
#11665=CARTESIAN_POINT ( 'NONE',  ( 103.5355339059327093, 3.535533905932755072, 14.62500000000000000 ) ) ;
#11675=EDGE_CURVE ( 'NONE', #3896, #14666, #2650, .T. ) ;
#11679=CARTESIAN_POINT ( 'NONE',  ( 104.4587341249999781, 1.846868145590750299, 5.250000001365592972 ) ) ;
#11681=CARTESIAN_POINT ( 'NONE',  ( 99.99999999999995737, 4.458734125000016313, 8.187500001365592084 ) ) ;
#11694=CARTESIAN_POINT ( 'NONE',  ( 101.8468681455906903, 4.458734125000016313, 9.375000001365592084 ) ) ;
#11699=( BOUNDED_SURFACE ( )  B_SPLINE_SURFACE ( 1, 2, ( 
 ( #25086, #7836, #1163, #10093, #9551, #25222, #20540, #16529, #18536, #16097, #9693, #24804, #5711, #18252, #1293, #14377, #1022, #3567, #23093, #5286, #22960, #12225, #14239, #26960, #1435, #3422, #22818, #16247, #24944, #20815, #18393, #12089, #18806, #27240, #27099, #7551, #16388, #3287, #5430, #5574, #5236, #15765, #24328, #4957, #9357, #2676, #13901, #24754, #6933, #24472, #22482, #13619, #7206, #22341, #19913, #22628, #2811, #2947, #11618, #18050, #396, #11480, #3097, #7353, #18196, #20197, #18343, #4670, #11764, #26763, #15627, #11337, #682, #5095, #9078, #4812, #2532, #829, #20343, #15900, #24617, #22197, #6791, #17773, #26477, #9220, #26907, #20488, #7070, #20058, #13472, #16044, #969, #537, #17912, #26623, #15476, #24191, #13757, #9496, #9639, #13332, #22058, #11196, #9910, #16751, #25169, #27463, #20627, #14048, #1387, #27328, #3658, #10048, #12319, #7787, #1657, #7497, #27595, #9778, #10177, #5658, #16192, #7646, #24899, #18886, #5379, #5798, #21040, #22769, #25452, #1525, #3235, #18759, #8057, #7920, #10316, #16616, #18625, #11902, #1111, #18486, #16474, #5932, #14322, #25309, #27195, #27048, #20763, #16338, #25038, #23043, #3516, #14600, #12175, #5520, #20905, #14464, #22905, #23318, #3791, #14187, #23182, #12450, #21176, #3368, #12039, #1248, #8755, #28013, #15151, #23870, #2073, #3932, #15012, #15297, #19591, #2218, #4207, #2360, #16886, #17447, #10741, #19171, #23590, #12866, #17305, #12591, #8335, #14734, #13003, #4349, #8477, #17166, #6205, #19024, #1798, #10463, #21458, #10882, #6613, #19312, #4072, #25722, #74, #4491, #12734, #19451, #27873, #23734, #28150, #17019, #8617, #21886, #26005, #1936, #25869, #25585, #27736, #14875, #26146, #6476, #6338, #24013, #10605 ),
 ( #21596, #13148, #21743, #8196, #6068, #23454, #21315, #19471, #13167, #21906, #2380, #11038, #23750, #13311, #19609, #231, #6633, #23890, #4227, #4369, #21476, #28170, #6495, #6774, #19748, #17464, #8918, #24031, #2092, #17606, #13025, #17184, #23614, #17329, #10624, #8639, #25745, #10760, #22038, #6227, #28033, #26313, #19192, #1954, #4510, #2514, #21762, #15460, #26024, #15033, #17041, #4652, #15171, #2239, #14893, #24175, #27894, #10901, #26166, #94, #8775, #8499, #15317, #8355, #4090, #25890, #12755, #19329, #6359, #12886, #21616, #810, #4794, #9338, #17895, #20323, #18032, #16175, #7187, #15748, #27034, #520, #3081, #14028, #13453, #951, #16026, #11746, #22753, #26603, #22465, #20472, #19894, #24739, #18327, #20041, #26745, #2795, #24883, #15885, #17757, #24601, #5362, #7480, #11176, #4938, #20181, #5079, #22179, #9062, #9622, #26891, #9201, #378, #2930, #26460, #6914, #15605, #7049, #24308, #2658, #11319, #5220, #24452, #13741, #13601, #11600, #22324, #11462, #665, #9478, #18180, #7337, #13885, #22611, #1752, #10558, #8285, #23406, #12407, #3881, #4165, #25817, #1613, #8008, #14687, #25676, #10418, #3218, #21415, #25406, #19124, #10271, #12690, #27831, #8569, #16976, #8152, #19401, #21127, #23688, #6434, #5888, #21551, #8424, #12825, #15102, #18980, #14824, #2026, #11885, #17113, #10694, #27689, #6157, #12542, #17260, #23547, #9761, #4024, #25961, #28105, #20610, #25543, #21268, #1893, #14558, #1094, #18471, #19268, #16845, #27551, #27967, #16708, #23273, #3746, #6292, #14969, #6023, #4582, #9136, #17401, #13242, #11112, #27, #26533, #4874, #26101, #11256, #17829, #6566, #15684, #19975, #24105, #6990, #24385, #13538, #22259, #170, #17972, #24245, #2734, #454, #311, #8852 ) ),
 .UNSPECIFIED., .F., .F., .F. ) 
 B_SPLINE_SURFACE_WITH_KNOTS ( ( 2, 2 ),
 ( 3, 2, 2, 2, 2, 2, 2, 2, 2, 2, 2, 2, 2, 2, 2, 2, 2, 2, 2, 2, 2, 2, 2, 2, 2, 2, 2, 2, 2, 2, 2, 2, 2, 2, 2, 2, 2, 2, 2, 2, 2, 2, 2, 2, 2, 2, 2, 2, 2, 2, 2, 2, 2, 2, 2, 2, 2, 2, 2, 2, 2, 2, 2, 2, 2, 2, 2, 2, 2, 2, 2, 2, 2, 2, 2, 2, 2, 2, 2, 2, 2, 2, 2, 2, 2, 2, 2, 2, 2, 2, 2, 2, 2, 2, 2, 2, 2, 2, 2, 2, 2, 2, 2, 2, 2, 2, 2, 2, 2, 2, 2, 2, 3 ),
 ( 0.000000000000000000, 1.000000000000000000 ),
 ( 0.000000000000000000, 0.008928571428571428076, 0.01785714285714285615, 0.02678571428571428423, 0.03571428571428571230, 0.04464285714285714385, 0.05357142857142856845, 0.06250000000000000000, 0.07142857142857142461, 0.08035714285714286309, 0.08928571428571428770, 0.09821428571428571230, 0.1071428571428571369, 0.1160714285714285754, 0.1250000000000000000, 0.1339285714285714246, 0.1428571428571428492, 0.1517857142857142738, 0.1607142857142857262, 0.1696428571428571508, 0.1785714285714285754, 0.1875000000000000000, 0.1964285714285714246, 0.2053571428571428492, 0.2142857142857142738, 0.2232142857142857262, 0.2321428571428571508, 0.2410714285714285754, 0.2500000000000000000, 0.2589285714285714524, 0.2678571428571428492, 0.2767857142857143016, 0.2857142857142856984, 0.2946428571428571508, 0.3035714285714285476, 0.3125000000000000000, 0.3214285714285714524, 0.3303571428571428492, 0.3392857142857143016, 0.3482142857142856984, 0.3571428571428571508, 0.3660714285714285476, 0.3750000000000000000, 0.3839285714285714524, 0.3928571428571428492, 0.4017857142857143016, 0.4107142857142856984, 0.4196428571428571508, 0.4285714285714285476, 0.4375000000000000000, 0.4464285714285714524, 0.4553571428571428492, 0.4642857142857143016, 0.4732142857142856984, 0.4821428571428571508, 0.4910714285714285476, 0.5000000000000000000, 0.5089285714285713969, 0.5178571428571429047, 0.5267857142857143016, 0.5357142857142856984, 0.5446428571428570953, 0.5535714285714286031, 0.5625000000000000000, 0.5714285714285713969, 0.5803571428571429047, 0.5892857142857143016, 0.5982142857142856984, 0.6071428571428570953, 0.6160714285714286031, 0.6250000000000000000, 0.6339285714285713969, 0.6428571428571429047, 0.6517857142857143016, 0.6607142857142856984, 0.6696428571428570953, 0.6785714285714286031, 0.6875000000000000000, 0.6964285714285713969, 0.7053571428571429047, 0.7142857142857143016, 0.7232142857142856984, 0.7321428571428570953, 0.7410714285714286031, 0.7500000000000000000, 0.7589285714285713969, 0.7678571428571429047, 0.7767857142857143016, 0.7857142857142856984, 0.7946428571428570953, 0.8035714285714286031, 0.8125000000000000000, 0.8214285714285713969, 0.8303571428571429047, 0.8392857142857143016, 0.8482142857142856984, 0.8571428571428570953, 0.8660714285714286031, 0.8750000000000000000, 0.8839285714285713969, 0.8928571428571429047, 0.9017857142857143016, 0.9107142857142856984, 0.9196428571428570953, 0.9285714285714286031, 0.9375000000000000000, 0.9464285714285713969, 0.9553571428571429047, 0.9642857142857143016, 0.9732142857142856984, 0.9821428571428570953, 0.9910714285714286031, 1.000000000000000000 ),
 .UNSPECIFIED. ) 
 GEOMETRIC_REPRESENTATION_ITEM ( )  RATIONAL_B_SPLINE_SURFACE ( (
 ( 1.000000000000000000, 0.9238795325112867385, 1.000000000000000000, 0.9238795325112867385, 1.000000000000000000, 0.9238795325112867385, 1.000000000000000000, 0.9238795325112867385, 1.000000000000000000, 0.9238795325112867385, 1.000000000000000000, 0.9238795325112867385, 1.000000000000000000, 0.9238795325112867385, 1.000000000000000000, 0.9238795325112867385, 1.000000000000000000, 0.9238795325112867385, 1.000000000000000000, 0.9238795325112867385, 1.000000000000000000, 0.9238795325112867385, 1.000000000000000000, 0.9238795325112867385, 1.000000000000000000, 0.9238795325112867385, 1.000000000000000000, 0.9238795325112867385, 1.000000000000000000, 0.9238795325112867385, 1.000000000000000000, 0.9238795325112867385, 1.000000000000000000, 0.9238795325112867385, 1.000000000000000000, 0.9238795325112867385, 1.000000000000000000, 0.9238795325112867385, 1.000000000000000000, 0.9238795325112867385, 1.000000000000000000, 0.9238795325112867385, 1.000000000000000000, 0.9238795325112867385, 1.000000000000000000, 0.9238795325112867385, 1.000000000000000000, 0.9238795325112867385, 1.000000000000000000, 0.9238795325112867385, 1.000000000000000000, 0.9238795325112867385, 1.000000000000000000, 0.9238795325112867385, 1.000000000000000000, 0.9238795325112867385, 1.000000000000000000, 0.9238795325112867385, 1.000000000000000000, 0.9238795325112867385, 1.000000000000000000, 0.9238795325112867385, 1.000000000000000000, 0.9238795325112867385, 1.000000000000000000, 0.9238795325112867385, 1.000000000000000000, 0.9238795325112867385, 1.000000000000000000, 0.9238795325112867385, 1.000000000000000000, 0.9238795325112867385, 1.000000000000000000, 0.9238795325112867385, 1.000000000000000000, 0.9238795325112867385, 1.000000000000000000, 0.9238795325112867385, 1.000000000000000000, 0.9238795325112867385, 1.000000000000000000, 0.9238795325112867385, 1.000000000000000000, 0.9238795325112867385, 1.000000000000000000, 0.9238795325112867385, 1.000000000000000000, 0.9238795325112867385, 1.000000000000000000, 0.9238795325112867385, 1.000000000000000000, 0.9238795325112867385, 1.000000000000000000, 0.9238795325112867385, 1.000000000000000000, 0.9238795325112867385, 1.000000000000000000, 0.9238795325112867385, 1.000000000000000000, 0.9238795325112867385, 1.000000000000000000, 0.9238795325112867385, 1.000000000000000000, 0.9238795325112867385, 1.000000000000000000, 0.9238795325112867385, 1.000000000000000000, 0.9238795325112867385, 1.000000000000000000, 0.9238795325112867385, 1.000000000000000000, 0.9238795325112867385, 1.000000000000000000, 0.9238795325112867385, 1.000000000000000000, 0.9238795325112867385, 1.000000000000000000, 0.9238795325112867385, 1.000000000000000000, 0.9238795325112867385, 1.000000000000000000, 0.9238795325112867385, 1.000000000000000000, 0.9238795325112867385, 1.000000000000000000, 0.9238795325112867385, 1.000000000000000000, 0.9238795325112867385, 1.000000000000000000, 0.9238795325112867385, 1.000000000000000000, 0.9238795325112867385, 1.000000000000000000, 0.9238795325112867385, 1.000000000000000000, 0.9238795325112867385, 1.000000000000000000, 0.9238795325112867385, 1.000000000000000000, 0.9238795325112867385, 1.000000000000000000, 0.9238795325112867385, 1.000000000000000000, 0.9238795325112867385, 1.000000000000000000, 0.9238795325112867385, 1.000000000000000000, 0.9238795325112867385, 1.000000000000000000, 0.9238795325112867385, 1.000000000000000000, 0.9238795325112867385, 1.000000000000000000, 0.9238795325112867385, 1.000000000000000000, 0.9238795325112867385, 1.000000000000000000, 0.9238795325112867385, 1.000000000000000000, 0.9238795325112867385, 1.000000000000000000, 0.9238795325112867385, 1.000000000000000000, 0.9238795325112867385, 1.000000000000000000, 0.9238795325112867385, 1.000000000000000000, 0.9238795325112867385, 1.000000000000000000, 0.9238795325112867385, 1.000000000000000000, 0.9238795325112867385, 1.000000000000000000, 0.9238795325112867385, 1.000000000000000000, 0.9238795325112867385, 1.000000000000000000, 0.9238795325112867385, 1.000000000000000000, 0.9238795325112867385, 1.000000000000000000, 0.9238795325112867385, 1.000000000000000000, 0.9238795325112867385, 1.000000000000000000, 0.9238795325112867385, 1.000000000000000000, 0.9238795325112867385, 1.000000000000000000, 0.9238795325112867385, 1.000000000000000000, 0.9238795325112867385, 1.000000000000000000, 0.9238795325112867385, 1.000000000000000000, 0.9238795325112867385, 1.000000000000000000, 0.9238795325112867385, 1.000000000000000000, 0.9238795325112867385, 1.000000000000000000, 0.9238795325112867385, 1.000000000000000000, 0.9238795325112867385, 1.000000000000000000, 0.9238795325112867385, 1.000000000000000000, 0.9238795325112867385, 1.000000000000000000, 0.9238795325112867385, 1.000000000000000000, 0.9238795325112867385, 1.000000000000000000, 0.9238795325112867385, 1.000000000000000000, 0.9238795325112867385, 1.000000000000000000, 0.9238795325112867385, 1.000000000000000000, 0.9238795325112867385, 1.000000000000000000, 0.9238795325112867385, 1.000000000000000000, 0.9238795325112867385, 1.000000000000000000),
 ( 1.000000000000000000, 0.9238795325112867385, 1.000000000000000000, 0.9238795325112867385, 1.000000000000000000, 0.9238795325112867385, 1.000000000000000000, 0.9238795325112867385, 1.000000000000000000, 0.9238795325112867385, 1.000000000000000000, 0.9238795325112867385, 1.000000000000000000, 0.9238795325112867385, 1.000000000000000000, 0.9238795325112867385, 1.000000000000000000, 0.9238795325112867385, 1.000000000000000000, 0.9238795325112867385, 1.000000000000000000, 0.9238795325112867385, 1.000000000000000000, 0.9238795325112867385, 1.000000000000000000, 0.9238795325112867385, 1.000000000000000000, 0.9238795325112867385, 1.000000000000000000, 0.9238795325112867385, 1.000000000000000000, 0.9238795325112867385, 1.000000000000000000, 0.9238795325112867385, 1.000000000000000000, 0.9238795325112867385, 1.000000000000000000, 0.9238795325112867385, 1.000000000000000000, 0.9238795325112867385, 1.000000000000000000, 0.9238795325112867385, 1.000000000000000000, 0.9238795325112867385, 1.000000000000000000, 0.9238795325112867385, 1.000000000000000000, 0.9238795325112867385, 1.000000000000000000, 0.9238795325112867385, 1.000000000000000000, 0.9238795325112867385, 1.000000000000000000, 0.9238795325112867385, 1.000000000000000000, 0.9238795325112867385, 1.000000000000000000, 0.9238795325112867385, 1.000000000000000000, 0.9238795325112867385, 1.000000000000000000, 0.9238795325112867385, 1.000000000000000000, 0.9238795325112867385, 1.000000000000000000, 0.9238795325112867385, 1.000000000000000000, 0.9238795325112867385, 1.000000000000000000, 0.9238795325112867385, 1.000000000000000000, 0.9238795325112867385, 1.000000000000000000, 0.9238795325112867385, 1.000000000000000000, 0.9238795325112867385, 1.000000000000000000, 0.9238795325112867385, 1.000000000000000000, 0.9238795325112867385, 1.000000000000000000, 0.9238795325112867385, 1.000000000000000000, 0.9238795325112867385, 1.000000000000000000, 0.9238795325112867385, 1.000000000000000000, 0.9238795325112867385, 1.000000000000000000, 0.9238795325112867385, 1.000000000000000000, 0.9238795325112867385, 1.000000000000000000, 0.9238795325112867385, 1.000000000000000000, 0.9238795325112867385, 1.000000000000000000, 0.9238795325112867385, 1.000000000000000000, 0.9238795325112867385, 1.000000000000000000, 0.9238795325112867385, 1.000000000000000000, 0.9238795325112867385, 1.000000000000000000, 0.9238795325112867385, 1.000000000000000000, 0.9238795325112867385, 1.000000000000000000, 0.9238795325112867385, 1.000000000000000000, 0.9238795325112867385, 1.000000000000000000, 0.9238795325112867385, 1.000000000000000000, 0.9238795325112867385, 1.000000000000000000, 0.9238795325112867385, 1.000000000000000000, 0.9238795325112867385, 1.000000000000000000, 0.9238795325112867385, 1.000000000000000000, 0.9238795325112867385, 1.000000000000000000, 0.9238795325112867385, 1.000000000000000000, 0.9238795325112867385, 1.000000000000000000, 0.9238795325112867385, 1.000000000000000000, 0.9238795325112867385, 1.000000000000000000, 0.9238795325112867385, 1.000000000000000000, 0.9238795325112867385, 1.000000000000000000, 0.9238795325112867385, 1.000000000000000000, 0.9238795325112867385, 1.000000000000000000, 0.9238795325112867385, 1.000000000000000000, 0.9238795325112867385, 1.000000000000000000, 0.9238795325112867385, 1.000000000000000000, 0.9238795325112867385, 1.000000000000000000, 0.9238795325112867385, 1.000000000000000000, 0.9238795325112867385, 1.000000000000000000, 0.9238795325112867385, 1.000000000000000000, 0.9238795325112867385, 1.000000000000000000, 0.9238795325112867385, 1.000000000000000000, 0.9238795325112867385, 1.000000000000000000, 0.9238795325112867385, 1.000000000000000000, 0.9238795325112867385, 1.000000000000000000, 0.9238795325112867385, 1.000000000000000000, 0.9238795325112867385, 1.000000000000000000, 0.9238795325112867385, 1.000000000000000000, 0.9238795325112867385, 1.000000000000000000, 0.9238795325112867385, 1.000000000000000000, 0.9238795325112867385, 1.000000000000000000, 0.9238795325112867385, 1.000000000000000000, 0.9238795325112867385, 1.000000000000000000, 0.9238795325112867385, 1.000000000000000000, 0.9238795325112867385, 1.000000000000000000, 0.9238795325112867385, 1.000000000000000000, 0.9238795325112867385, 1.000000000000000000, 0.9238795325112867385, 1.000000000000000000, 0.9238795325112867385, 1.000000000000000000, 0.9238795325112867385, 1.000000000000000000, 0.9238795325112867385, 1.000000000000000000, 0.9238795325112867385, 1.000000000000000000, 0.9238795325112867385, 1.000000000000000000, 0.9238795325112867385, 1.000000000000000000, 0.9238795325112867385, 1.000000000000000000, 0.9238795325112867385, 1.000000000000000000, 0.9238795325112867385, 1.000000000000000000, 0.9238795325112867385, 1.000000000000000000, 0.9238795325112867385, 1.000000000000000000, 0.9238795325112867385, 1.000000000000000000, 0.9238795325112867385, 1.000000000000000000, 0.9238795325112867385, 1.000000000000000000, 0.9238795325112867385, 1.000000000000000000, 0.9238795325112867385, 1.000000000000000000, 0.9238795325112867385, 1.000000000000000000) ) ) 
 REPRESENTATION_ITEM ( '' )  SURFACE ( )  );
#11712=CARTESIAN_POINT ( 'NONE',  ( 104.4587341249999781, -1.846868145590721655, 7.125000001365593860 ) ) ;
#11741=ORIENTED_EDGE ( 'NONE', *, *, #10447, .T. ) ;
#11743=CARTESIAN_POINT ( 'NONE',  ( 99.99999999999995737, 4.458734125000016313, 6.187500001365592084 ) ) ;
#11744=VERTEX_POINT ( 'NONE', #11455 ) ;
#11746=CARTESIAN_POINT ( 'NONE',  ( 104.4587341249999781, 1.846868145590750299, 9.000000001365593860 ) ) ;
#11759=ADVANCED_FACE ( 'NONE', ( #803 ), #13877, .F. ) ;
#11764=CARTESIAN_POINT ( 'NONE',  ( 99.99999999999995737, 5.000000000000018652, 9.875000002731185944 ) ) ;
#11793=( BOUNDED_SURFACE ( )  B_SPLINE_SURFACE ( 1, 2, ( 
 ( #19561, #19699, #28121, #25978, #17135, #15120, #12977, #2187, #26117, #43, #15409, #6723, #24125, #21988, #13257, #21713, #8726, #6582, #26408, #2466, #23983, #11127, #4461, #13117, #19841, #328, #9014, #17706, #6867, #9288, #24969, #26693, #7144, #17984, #13974, #1045, #20565, #9717, #7288, #24829, #15838, #469, #5453, #9427, #22702, #18419, #2750, #20269, #13696, #15978, #11413, #22130, #2609, #5169, #5313, #17846, #3169, #22558, #11841, #2882, #13833, #7004, #15698, #19991, #7576, #16271, #22412, #18128, #11553, #7429, #9573, #16123, #27125, #11271, #24401, #755, #26840, #9153, #18278, #13552, #26984, #20133, #26549, #24692, #3025, #11694, #4889, #20417, #24547, #22276, #5030, #612, #903, #5736, #16413, #22983, #6006, #12392, #14263, #16693, #12252, #14403, #7721, #27537, #1599, #5873, #25109, #23257, #5597, #9855, #7860, #25659, #22844, #3450, #23120, #20706, #3594, #18829, #21113, #14671, #1460, #18966, #27673, #20980, #23392, #8137, #12116, #10256, #18562, #14542, #14121, #20842, #3865, #18697, #12526, #21255, #27265, #25246, #16959, #3311, #7994, #1188, #16831, #10117, #1736, #1320, #25527, #27400, #16555, #9988, #10402, #19108, #27816, #8270, #25392, #11982, #3732, #12674, #17667, #21675, #6687, #13226, #14952, #4284, #25943, #9, #23671, #8978, #14807, #17384, #17526, #1878, #8836, #6550, #26228, #15087, #26083, #19248, #27949, #4008, #19810, #293, #6418, #2151, #23806, #19667, #21821, #150, #15374, #24090, #8407, #12941, #10813, #2437, #2297, #25799, #10956, #4149, #21400, #19528, #8694, #15230, #6142, #23948, #10676, #4565, #2008, #21958, #23531, #4429, #17096, #12809, #11097, #13082, #6275, #10541, #21532, #19384, #28089, #8552, #17240, #18096, #9120, #7257, #17814 ),
 ( #17954, #2853, #24662, #26954, #13665, #2993, #11665, #26665, #18247, #20387, #6974, #5137, #22100, #26808, #9686, #15669, #7398, #2721, #16091, #24798, #2580, #9260, #1017, #26375, #11521, #13371, #874, #22380, #5281, #19958, #9545, #11382, #7111, #13802, #4856, #15522, #20103, #11239, #22526, #13523, #13945, #22242, #6832, #582, #20240, #22672, #15946, #26518, #3144, #24369, #435, #15811, #24230, #4711, #24516, #5002, #725, #9397, #11812, #20534, #18934, #5705, #23226, #3702, #9957, #10224, #12364, #27235, #16664, #14094, #18801, #1706, #7690, #27643, #22955, #8103, #16797, #22813, #1288, #21222, #18387, #23087, #5425, #21083, #14371, #25495, #11952, #1571, #3416, #18670, #5840, #25081, #7545, #12085, #3281, #25359, #5569, #14509, #14233, #27093, #20808, #27371, #7830, #5975, #14642, #23361, #3833, #3561, #12495, #16524, #24939, #16242, #12220, #20674, #1158, #16382, #25216, #20948, #1429, #10088, #9823, #18530, #27507, #7963, #6110, #13048, #10782, #21784, #19352, #2115, #23498, #3977, #8238, #24054, #4531, #10646, #25912, #28055, #23911, #26048, #4392, #2264, #10924, #12638, #8521, #6383, #6653, #6517, #1845, #15193, #8378, #16929, #17207, #15056, #23772, #21927, #19494, #14917, #8799, #6247, #19633, #13191, #1977, #21366, #19214, #115, #8660, #10508, #12908, #4249, #21641, #27918, #17063, #25767, #17488, #17351, #23638, #28193, #26187, #15339, #4114, #10365, #19074, #27779, #12779, #25629, #21495, #14777, #24334, #13907, #11061, #22065, #11343, #8940, #22203, #7076, #687, #2953, #17917, #7215, #15905, #2682, #22487, #24623, #11203, #9362, #26339, #2817, #2403, #19918, #11626, #6938, #20350, #835, #6797, #13481, #5242, #19773, #15772, #17629, #5100, #26628, #9504, #24197, #13764 ) ),
 .UNSPECIFIED., .F., .F., .F. ) 
 B_SPLINE_SURFACE_WITH_KNOTS ( ( 2, 2 ),
 ( 3, 2, 2, 2, 2, 2, 2, 2, 2, 2, 2, 2, 2, 2, 2, 2, 2, 2, 2, 2, 2, 2, 2, 2, 2, 2, 2, 2, 2, 2, 2, 2, 2, 2, 2, 2, 2, 2, 2, 2, 2, 2, 2, 2, 2, 2, 2, 2, 2, 2, 2, 2, 2, 2, 2, 2, 2, 2, 2, 2, 2, 2, 2, 2, 2, 2, 2, 2, 2, 2, 2, 2, 2, 2, 2, 2, 2, 2, 2, 2, 2, 2, 2, 2, 2, 2, 2, 2, 2, 2, 2, 2, 2, 2, 2, 2, 2, 2, 2, 2, 2, 2, 2, 2, 2, 2, 2, 2, 2, 2, 2, 2, 3 ),
 ( 0.000000000000000000, 1.000000000000000000 ),
 ( 0.000000000000000000, 0.008928571428571428076, 0.01785714285714285615, 0.02678571428571428423, 0.03571428571428571230, 0.04464285714285714385, 0.05357142857142856845, 0.06250000000000000000, 0.07142857142857142461, 0.08035714285714286309, 0.08928571428571428770, 0.09821428571428571230, 0.1071428571428571369, 0.1160714285714285754, 0.1250000000000000000, 0.1339285714285714246, 0.1428571428571428492, 0.1517857142857142738, 0.1607142857142857262, 0.1696428571428571508, 0.1785714285714285754, 0.1875000000000000000, 0.1964285714285714246, 0.2053571428571428492, 0.2142857142857142738, 0.2232142857142857262, 0.2321428571428571508, 0.2410714285714285754, 0.2500000000000000000, 0.2589285714285714524, 0.2678571428571428492, 0.2767857142857143016, 0.2857142857142856984, 0.2946428571428571508, 0.3035714285714285476, 0.3125000000000000000, 0.3214285714285714524, 0.3303571428571428492, 0.3392857142857143016, 0.3482142857142856984, 0.3571428571428571508, 0.3660714285714285476, 0.3750000000000000000, 0.3839285714285714524, 0.3928571428571428492, 0.4017857142857143016, 0.4107142857142856984, 0.4196428571428571508, 0.4285714285714285476, 0.4375000000000000000, 0.4464285714285714524, 0.4553571428571428492, 0.4642857142857143016, 0.4732142857142856984, 0.4821428571428571508, 0.4910714285714285476, 0.5000000000000000000, 0.5089285714285713969, 0.5178571428571429047, 0.5267857142857143016, 0.5357142857142856984, 0.5446428571428570953, 0.5535714285714286031, 0.5625000000000000000, 0.5714285714285713969, 0.5803571428571429047, 0.5892857142857143016, 0.5982142857142856984, 0.6071428571428570953, 0.6160714285714286031, 0.6250000000000000000, 0.6339285714285713969, 0.6428571428571429047, 0.6517857142857143016, 0.6607142857142856984, 0.6696428571428570953, 0.6785714285714286031, 0.6875000000000000000, 0.6964285714285713969, 0.7053571428571429047, 0.7142857142857143016, 0.7232142857142856984, 0.7321428571428570953, 0.7410714285714286031, 0.7500000000000000000, 0.7589285714285713969, 0.7678571428571429047, 0.7767857142857143016, 0.7857142857142856984, 0.7946428571428570953, 0.8035714285714286031, 0.8125000000000000000, 0.8214285714285713969, 0.8303571428571429047, 0.8392857142857143016, 0.8482142857142856984, 0.8571428571428570953, 0.8660714285714286031, 0.8750000000000000000, 0.8839285714285713969, 0.8928571428571429047, 0.9017857142857143016, 0.9107142857142856984, 0.9196428571428570953, 0.9285714285714286031, 0.9375000000000000000, 0.9464285714285713969, 0.9553571428571429047, 0.9642857142857143016, 0.9732142857142856984, 0.9821428571428570953, 0.9910714285714286031, 1.000000000000000000 ),
 .UNSPECIFIED. ) 
 GEOMETRIC_REPRESENTATION_ITEM ( )  RATIONAL_B_SPLINE_SURFACE ( (
 ( 1.000000000000000000, 0.9238795325112867385, 1.000000000000000000, 0.9238795325112867385, 1.000000000000000000, 0.9238795325112867385, 1.000000000000000000, 0.9238795325112867385, 1.000000000000000000, 0.9238795325112867385, 1.000000000000000000, 0.9238795325112867385, 1.000000000000000000, 0.9238795325112867385, 1.000000000000000000, 0.9238795325112867385, 1.000000000000000000, 0.9238795325112867385, 1.000000000000000000, 0.9238795325112867385, 1.000000000000000000, 0.9238795325112867385, 1.000000000000000000, 0.9238795325112867385, 1.000000000000000000, 0.9238795325112867385, 1.000000000000000000, 0.9238795325112867385, 1.000000000000000000, 0.9238795325112867385, 1.000000000000000000, 0.9238795325112867385, 1.000000000000000000, 0.9238795325112867385, 1.000000000000000000, 0.9238795325112867385, 1.000000000000000000, 0.9238795325112867385, 1.000000000000000000, 0.9238795325112867385, 1.000000000000000000, 0.9238795325112867385, 1.000000000000000000, 0.9238795325112867385, 1.000000000000000000, 0.9238795325112867385, 1.000000000000000000, 0.9238795325112867385, 1.000000000000000000, 0.9238795325112867385, 1.000000000000000000, 0.9238795325112867385, 1.000000000000000000, 0.9238795325112867385, 1.000000000000000000, 0.9238795325112867385, 1.000000000000000000, 0.9238795325112867385, 1.000000000000000000, 0.9238795325112867385, 1.000000000000000000, 0.9238795325112867385, 1.000000000000000000, 0.9238795325112867385, 1.000000000000000000, 0.9238795325112867385, 1.000000000000000000, 0.9238795325112867385, 1.000000000000000000, 0.9238795325112867385, 1.000000000000000000, 0.9238795325112867385, 1.000000000000000000, 0.9238795325112867385, 1.000000000000000000, 0.9238795325112867385, 1.000000000000000000, 0.9238795325112867385, 1.000000000000000000, 0.9238795325112867385, 1.000000000000000000, 0.9238795325112867385, 1.000000000000000000, 0.9238795325112867385, 1.000000000000000000, 0.9238795325112867385, 1.000000000000000000, 0.9238795325112867385, 1.000000000000000000, 0.9238795325112867385, 1.000000000000000000, 0.9238795325112867385, 1.000000000000000000, 0.9238795325112867385, 1.000000000000000000, 0.9238795325112867385, 1.000000000000000000, 0.9238795325112867385, 1.000000000000000000, 0.9238795325112867385, 1.000000000000000000, 0.9238795325112867385, 1.000000000000000000, 0.9238795325112867385, 1.000000000000000000, 0.9238795325112867385, 1.000000000000000000, 0.9238795325112867385, 1.000000000000000000, 0.9238795325112867385, 1.000000000000000000, 0.9238795325112867385, 1.000000000000000000, 0.9238795325112867385, 1.000000000000000000, 0.9238795325112867385, 1.000000000000000000, 0.9238795325112867385, 1.000000000000000000, 0.9238795325112867385, 1.000000000000000000, 0.9238795325112867385, 1.000000000000000000, 0.9238795325112867385, 1.000000000000000000, 0.9238795325112867385, 1.000000000000000000, 0.9238795325112867385, 1.000000000000000000, 0.9238795325112867385, 1.000000000000000000, 0.9238795325112867385, 1.000000000000000000, 0.9238795325112867385, 1.000000000000000000, 0.9238795325112867385, 1.000000000000000000, 0.9238795325112867385, 1.000000000000000000, 0.9238795325112867385, 1.000000000000000000, 0.9238795325112867385, 1.000000000000000000, 0.9238795325112867385, 1.000000000000000000, 0.9238795325112867385, 1.000000000000000000, 0.9238795325112867385, 1.000000000000000000, 0.9238795325112867385, 1.000000000000000000, 0.9238795325112867385, 1.000000000000000000, 0.9238795325112867385, 1.000000000000000000, 0.9238795325112867385, 1.000000000000000000, 0.9238795325112867385, 1.000000000000000000, 0.9238795325112867385, 1.000000000000000000, 0.9238795325112867385, 1.000000000000000000, 0.9238795325112867385, 1.000000000000000000, 0.9238795325112867385, 1.000000000000000000, 0.9238795325112867385, 1.000000000000000000, 0.9238795325112867385, 1.000000000000000000, 0.9238795325112867385, 1.000000000000000000, 0.9238795325112867385, 1.000000000000000000, 0.9238795325112867385, 1.000000000000000000, 0.9238795325112867385, 1.000000000000000000, 0.9238795325112867385, 1.000000000000000000, 0.9238795325112867385, 1.000000000000000000, 0.9238795325112867385, 1.000000000000000000, 0.9238795325112867385, 1.000000000000000000, 0.9238795325112867385, 1.000000000000000000, 0.9238795325112867385, 1.000000000000000000, 0.9238795325112867385, 1.000000000000000000, 0.9238795325112867385, 1.000000000000000000, 0.9238795325112867385, 1.000000000000000000, 0.9238795325112867385, 1.000000000000000000, 0.9238795325112867385, 1.000000000000000000, 0.9238795325112867385, 1.000000000000000000, 0.9238795325112867385, 1.000000000000000000, 0.9238795325112867385, 1.000000000000000000, 0.9238795325112867385, 1.000000000000000000, 0.9238795325112867385, 1.000000000000000000, 0.9238795325112867385, 1.000000000000000000, 0.9238795325112867385, 1.000000000000000000, 0.9238795325112867385, 1.000000000000000000, 0.9238795325112867385, 1.000000000000000000, 0.9238795325112867385, 1.000000000000000000, 0.9238795325112867385, 1.000000000000000000, 0.9238795325112867385, 1.000000000000000000),
 ( 1.000000000000000000, 0.9238795325112867385, 1.000000000000000000, 0.9238795325112867385, 1.000000000000000000, 0.9238795325112867385, 1.000000000000000000, 0.9238795325112867385, 1.000000000000000000, 0.9238795325112867385, 1.000000000000000000, 0.9238795325112867385, 1.000000000000000000, 0.9238795325112867385, 1.000000000000000000, 0.9238795325112867385, 1.000000000000000000, 0.9238795325112867385, 1.000000000000000000, 0.9238795325112867385, 1.000000000000000000, 0.9238795325112867385, 1.000000000000000000, 0.9238795325112867385, 1.000000000000000000, 0.9238795325112867385, 1.000000000000000000, 0.9238795325112867385, 1.000000000000000000, 0.9238795325112867385, 1.000000000000000000, 0.9238795325112867385, 1.000000000000000000, 0.9238795325112867385, 1.000000000000000000, 0.9238795325112867385, 1.000000000000000000, 0.9238795325112867385, 1.000000000000000000, 0.9238795325112867385, 1.000000000000000000, 0.9238795325112867385, 1.000000000000000000, 0.9238795325112867385, 1.000000000000000000, 0.9238795325112867385, 1.000000000000000000, 0.9238795325112867385, 1.000000000000000000, 0.9238795325112867385, 1.000000000000000000, 0.9238795325112867385, 1.000000000000000000, 0.9238795325112867385, 1.000000000000000000, 0.9238795325112867385, 1.000000000000000000, 0.9238795325112867385, 1.000000000000000000, 0.9238795325112867385, 1.000000000000000000, 0.9238795325112867385, 1.000000000000000000, 0.9238795325112867385, 1.000000000000000000, 0.9238795325112867385, 1.000000000000000000, 0.9238795325112867385, 1.000000000000000000, 0.9238795325112867385, 1.000000000000000000, 0.9238795325112867385, 1.000000000000000000, 0.9238795325112867385, 1.000000000000000000, 0.9238795325112867385, 1.000000000000000000, 0.9238795325112867385, 1.000000000000000000, 0.9238795325112867385, 1.000000000000000000, 0.9238795325112867385, 1.000000000000000000, 0.9238795325112867385, 1.000000000000000000, 0.9238795325112867385, 1.000000000000000000, 0.9238795325112867385, 1.000000000000000000, 0.9238795325112867385, 1.000000000000000000, 0.9238795325112867385, 1.000000000000000000, 0.9238795325112867385, 1.000000000000000000, 0.9238795325112867385, 1.000000000000000000, 0.9238795325112867385, 1.000000000000000000, 0.9238795325112867385, 1.000000000000000000, 0.9238795325112867385, 1.000000000000000000, 0.9238795325112867385, 1.000000000000000000, 0.9238795325112867385, 1.000000000000000000, 0.9238795325112867385, 1.000000000000000000, 0.9238795325112867385, 1.000000000000000000, 0.9238795325112867385, 1.000000000000000000, 0.9238795325112867385, 1.000000000000000000, 0.9238795325112867385, 1.000000000000000000, 0.9238795325112867385, 1.000000000000000000, 0.9238795325112867385, 1.000000000000000000, 0.9238795325112867385, 1.000000000000000000, 0.9238795325112867385, 1.000000000000000000, 0.9238795325112867385, 1.000000000000000000, 0.9238795325112867385, 1.000000000000000000, 0.9238795325112867385, 1.000000000000000000, 0.9238795325112867385, 1.000000000000000000, 0.9238795325112867385, 1.000000000000000000, 0.9238795325112867385, 1.000000000000000000, 0.9238795325112867385, 1.000000000000000000, 0.9238795325112867385, 1.000000000000000000, 0.9238795325112867385, 1.000000000000000000, 0.9238795325112867385, 1.000000000000000000, 0.9238795325112867385, 1.000000000000000000, 0.9238795325112867385, 1.000000000000000000, 0.9238795325112867385, 1.000000000000000000, 0.9238795325112867385, 1.000000000000000000, 0.9238795325112867385, 1.000000000000000000, 0.9238795325112867385, 1.000000000000000000, 0.9238795325112867385, 1.000000000000000000, 0.9238795325112867385, 1.000000000000000000, 0.9238795325112867385, 1.000000000000000000, 0.9238795325112867385, 1.000000000000000000, 0.9238795325112867385, 1.000000000000000000, 0.9238795325112867385, 1.000000000000000000, 0.9238795325112867385, 1.000000000000000000, 0.9238795325112867385, 1.000000000000000000, 0.9238795325112867385, 1.000000000000000000, 0.9238795325112867385, 1.000000000000000000, 0.9238795325112867385, 1.000000000000000000, 0.9238795325112867385, 1.000000000000000000, 0.9238795325112867385, 1.000000000000000000, 0.9238795325112867385, 1.000000000000000000, 0.9238795325112867385, 1.000000000000000000, 0.9238795325112867385, 1.000000000000000000, 0.9238795325112867385, 1.000000000000000000, 0.9238795325112867385, 1.000000000000000000, 0.9238795325112867385, 1.000000000000000000, 0.9238795325112867385, 1.000000000000000000, 0.9238795325112867385, 1.000000000000000000, 0.9238795325112867385, 1.000000000000000000, 0.9238795325112867385, 1.000000000000000000, 0.9238795325112867385, 1.000000000000000000, 0.9238795325112867385, 1.000000000000000000, 0.9238795325112867385, 1.000000000000000000, 0.9238795325112867385, 1.000000000000000000, 0.9238795325112867385, 1.000000000000000000, 0.9238795325112867385, 1.000000000000000000, 0.9238795325112867385, 1.000000000000000000, 0.9238795325112867385, 1.000000000000000000, 0.9238795325112867385, 1.000000000000000000, 0.9238795325112867385, 1.000000000000000000, 0.9238795325112867385, 1.000000000000000000) ) ) 
 REPRESENTATION_ITEM ( '' )  SURFACE ( )  );
#11800=AXIS2_PLACEMENT_3D ( 'NONE', #5948, #3807, #7937 ) ;
#11812=CARTESIAN_POINT ( 'NONE',  ( 103.5355339059327093, -3.535533905932726206, 11.37500000000000000 ) ) ;
#11817=CARTESIAN_POINT ( 'NONE',  ( 103.5355339059327093, 3.535533905932755072, 0.7500000027311857220 ) ) ;
#11818=DIRECTION ( 'NONE',  ( 0.000000000000000000, 1.000000000000000000, 0.000000000000000000 ) ) ;
#11825=CARTESIAN_POINT ( 'NONE',  ( 95.54126587499995082, 1.846868145590750077, 5.625000001365593860 ) ) ;
#11827=CARTESIAN_POINT ( 'NONE',  ( 104.4587341249999781, -1.846868145590721655, 10.87500000136559208 ) ) ;
#11841=CARTESIAN_POINT ( 'NONE',  ( 103.1528011352953342, -3.152801135295355106, 11.06250000136559208 ) ) ;
#11846=LINE ( 'NONE', #1465, #28165 ) ;
#11847=CARTESIAN_POINT ( 'NONE',  ( 94.99999999999995737, 1.387778780781445676E-14, 14.12500000273118594 ) ) ;
#11856=CARTESIAN_POINT ( 'NONE',  ( 98.15313185440923860, 4.458734125000016313, 5.500000001365592972 ) ) ;
#11875=( BOUNDED_CURVE ( )  B_SPLINE_CURVE ( 2, ( #19223, #6253, #21504, #14926, #23646, #28061, #21649, #1984, #10788 ),
 .UNSPECIFIED., .F., .F. ) 
 B_SPLINE_CURVE_WITH_KNOTS ( ( 3, 2, 2, 2, 3 ),
 ( 0.6428571428571427937, 0.6517857142857141906, 0.6607142857142855874, 0.6696428571428569843, 0.6785714285714284921 ),
 .UNSPECIFIED. ) 
 CURVE ( )  GEOMETRIC_REPRESENTATION_ITEM ( )  RATIONAL_B_SPLINE_CURVE ( ( 1.000000000000000888, 0.9238795325112857393, 1.000000000000000000, 0.9238795325112867385, 1.000000000000000000, 0.9238795325112867385, 1.000000000000000000, 0.9238795325112877377, 0.9999999999999990008 ) ) 
 REPRESENTATION_ITEM ( '' )  );
#11882=CARTESIAN_POINT ( 'NONE',  ( 96.84719886470459471, 3.152801135295383084, 3.312500001365592972 ) ) ;
#11885=CARTESIAN_POINT ( 'NONE',  ( 103.1528011352953342, -3.152801135295355106, 3.812500001365591640 ) ) ;
#11902=CARTESIAN_POINT ( 'NONE',  ( 102.0710678118654329, -4.999999999999989342, 5.437500002731184168 ) ) ;
#11909=EDGE_CURVE ( 'NONE', #3132, #15219, #23159, .T. ) ;
#11952=CARTESIAN_POINT ( 'NONE',  ( 103.5355339059327093, 3.535533905932755072, 9.624999999999998224 ) ) ;
#11956=( BOUNDED_CURVE ( )  B_SPLINE_CURVE ( 2, ( #27282, #7739, #25680, #25966, #2031, #12830, #14829, #12966, #27556 ),
 .UNSPECIFIED., .F., .F. ) 
 B_SPLINE_CURVE_WITH_KNOTS ( ( 3, 2, 2, 2, 3 ),
 ( 0.4285714285714285476, 0.4375000000000000000, 0.4464285714285713969, 0.4553571428571427937, 0.4642857142857142461 ),
 .UNSPECIFIED. ) 
 CURVE ( )  GEOMETRIC_REPRESENTATION_ITEM ( )  RATIONAL_B_SPLINE_CURVE ( ( 1.000000000000000000, 0.9238795325112867385, 1.000000000000000000, 0.9238795325112867385, 1.000000000000000000, 0.9238795325112867385, 1.000000000000000000, 0.9238795325112871826, 0.9999999999999995559 ) ) 
 REPRESENTATION_ITEM ( '' )  );
#11958=CARTESIAN_POINT ( 'NONE',  ( 99.99999999999995737, 5.000000000000018652, 0.8750000027311858330 ) ) ;
#11961=CARTESIAN_POINT ( 'NONE',  ( 99.99999999999995737, 5.000000000000018652, 11.87500000273118594 ) ) ;
#11966=CARTESIAN_POINT ( 'NONE',  ( 95.54126587499995082, -1.846868145590724986, 6.750000001365592972 ) ) ;
#11968=CARTESIAN_POINT ( 'NONE',  ( 101.8468681455907046, 4.458734125000016313, 11.12500000136559208 ) ) ;
#11978=ADVANCED_FACE ( 'NONE', ( #10157 ), #10444, .F. ) ;
#11982=CARTESIAN_POINT ( 'NONE',  ( 101.8468681455906903, -4.458734124999987891, 5.000000001365592972 ) ) ;
#11994=CARTESIAN_POINT ( 'NONE',  ( 96.46446609406721961, 3.535533905932755072, 4.000000002731185056 ) ) ;
#11995=CARTESIAN_POINT ( 'NONE',  ( 104.4587341249999639, 1.442382525525748735E-14, 6.187500001365592084 ) ) ;
#12008=VERTEX_POINT ( 'NONE', #16734 ) ;
#12010=CARTESIAN_POINT ( 'NONE',  ( 102.0710678118654329, -4.999999999999989342, 0.4375000027311854445 ) ) ;
#12014=LINE ( 'NONE', #8173, #6152 ) ;
#12025=CARTESIAN_POINT ( 'NONE',  ( 99.99999999999995737, -4.458734124999988779, 2.687500001365592528 ) ) ;
#12039=CARTESIAN_POINT ( 'NONE',  ( 103.5355339059327093, 3.535533905932755072, 3.750000002731185056 ) ) ;
#12055=CARTESIAN_POINT ( 'NONE',  ( 99.99999999999995737, 4.458734125000016313, 13.18750000136559208 ) ) ;
#12074=ORIENTED_EDGE ( 'NONE', *, *, #10194, .F. ) ;
#12085=CARTESIAN_POINT ( 'NONE',  ( 97.92893218813451028, -4.999999999999989342, 9.187500000000000000 ) ) ;
#12089=CARTESIAN_POINT ( 'NONE',  ( 94.99999999999995737, -2.071067811865466624, 12.18750000273118950 ) ) ;
#12098=CARTESIAN_POINT ( 'NONE',  ( 99.99999999999995737, -4.458734124999988779, 8.937500001365592084 ) ) ;
#12100=CARTESIAN_POINT ( 'NONE',  ( 103.1528011352953342, -3.152801135295355106, 10.81250000136559208 ) ) ;
#12104=CARTESIAN_POINT ( 'NONE',  ( 102.0710678118654329, -4.999999999999989342, 9.312500000000000000 ) ) ;
#12116=CARTESIAN_POINT ( 'NONE',  ( 96.84719886470459471, -3.152801135295355994, 6.812500001365592084 ) ) ;
#12129=CARTESIAN_POINT ( 'NONE',  ( 95.54126587499996504, -1.846868145590724986, 2.750000001365592528 ) ) ;
#12142=CARTESIAN_POINT ( 'NONE',  ( 96.46446609406721961, -3.535533905932727539, 6.250000002731185056 ) ) ;
#12149=ORIENTED_EDGE ( 'NONE', *, *, #5102, .T. ) ;
#12158=( BOUNDED_CURVE ( )  B_SPLINE_CURVE ( 2, ( #17479, #26179, #6645, #24469, #15623, #9075, #13615, #26760, #965 ),
 .UNSPECIFIED., .F., .F. ) 
 B_SPLINE_CURVE_WITH_KNOTS ( ( 3, 2, 2, 2, 3 ),
 ( 0.4642857142857142461, 0.4732142857142856429, 0.4821428571428570953, 0.4910714285714284366, 0.4999999999999998890 ),
 .UNSPECIFIED. ) 
 CURVE ( )  GEOMETRIC_REPRESENTATION_ITEM ( )  RATIONAL_B_SPLINE_CURVE ( ( 1.000000000000000444, 0.9238795325112862944, 1.000000000000000000, 0.9238795325112867385, 1.000000000000000000, 0.9238795325112867385, 1.000000000000000000, 0.9238795325112877377, 0.9999999999999990008 ) ) 
 REPRESENTATION_ITEM ( '' )  );
#12160=CARTESIAN_POINT ( 'NONE',  ( 95.54126587499996504, 1.387778780781445676E-14, 0.4375000013655920839 ) ) ;
#12167=CARTESIAN_POINT ( 'NONE',  ( 97.92893218813451028, -4.999999999999989342, 6.187499999999998224 ) ) ;
#12175=CARTESIAN_POINT ( 'NONE',  ( 103.5355339059327093, -3.535533905932726206, 4.500000002731185944 ) ) ;
#12192=CARTESIAN_POINT ( 'NONE',  ( 103.1528011352953342, 3.152801135295383084, 12.06250000136559208 ) ) ;
#12196=( BOUNDED_CURVE ( )  B_SPLINE_CURVE ( 2, ( #9745, #14154, #16303, #12010, #3061, #20593, #22448, #24435, #1219 ),
 .UNSPECIFIED., .F., .F. ) 
 B_SPLINE_CURVE_WITH_KNOTS ( ( 3, 2, 2, 2, 3 ),
 ( 0.9642857142857141906, 0.9732142857142855874, 0.9821428571428569843, 0.9910714285714286031, 1.000000000000000000 ),
 .UNSPECIFIED. ) 
 CURVE ( )  GEOMETRIC_REPRESENTATION_ITEM ( )  RATIONAL_B_SPLINE_CURVE ( ( 1.000000000000000888, 0.9238795325112857393, 1.000000000000000000, 0.9238795325112867385, 1.000000000000000000, 0.9238795325112867385, 1.000000000000000000, 0.9238795325112867385, 1.000000000000000000 ) ) 
 REPRESENTATION_ITEM ( '' )  );
#12200=CARTESIAN_POINT ( 'NONE',  ( 104.9999999999999716, 2.071067811865491937, 2.687500002731185944 ) ) ;
#12220=CARTESIAN_POINT ( 'NONE',  ( 94.99999999999995737, 1.387778780781445676E-14, 8.000000000000000000 ) ) ;
#12221=ORIENTED_EDGE ( 'NONE', *, *, #6545, .F. ) ;
#12225=CARTESIAN_POINT ( 'NONE',  ( 102.0710678118654329, 5.000000000000018652, 12.81250000273118950 ) ) ;
#12234=CARTESIAN_POINT ( 'NONE',  ( 98.15313185440925281, 4.458734125000016313, 1.500000001365592972 ) ) ;
#12236=CARTESIAN_POINT ( 'NONE',  ( 101.8468681455907046, 4.458734125000016313, 5.125000001365592972 ) ) ;
#12252=CARTESIAN_POINT ( 'NONE',  ( 99.99999999999995737, 4.458734125000016313, 8.437500001365592084 ) ) ;
#12269=CARTESIAN_POINT ( 'NONE',  ( 98.15313185440923860, 4.458734125000016313, 3.500000001365592528 ) ) ;
#12283=DIRECTION ( 'NONE',  ( -0.000000000000000000, -0.000000000000000000, -1.000000000000000000 ) ) ;
#12303=CARTESIAN_POINT ( 'NONE',  ( 95.54126587499996504, -1.846868145590724986, 13.75000000136559386 ) ) ;
#12311=CARTESIAN_POINT ( 'NONE',  ( 102.0710678118654329, -4.999999999999989342, 6.312499999999998224 ) ) ;
#12319=CARTESIAN_POINT ( 'NONE',  ( 96.46446609406721961, 3.535533905932755072, 7.000000002731185056 ) ) ;
#12326=CARTESIAN_POINT ( 'NONE',  ( 99.99999999999995737, -4.999999999999990230, 9.375000002731184168 ) ) ;
#12339=CARTESIAN_POINT ( 'NONE',  ( 104.4587341249999639, 1.442382525525748735E-14, 11.93750000136559208 ) ) ;
#12346=CARTESIAN_POINT ( 'NONE',  ( 102.0710678118654329, 5.000000000000018652, 2.687499999999999112 ) ) ;
#12364=CARTESIAN_POINT ( 'NONE',  ( 96.46446609406721961, 3.535533905932755072, 10.87500000000000000 ) ) ;
#12374=LINE ( 'NONE', #25921, #7979 ) ;
#12378=CARTESIAN_POINT ( 'NONE',  ( 95.54126587499995082, 1.846868145590750077, 4.625000001365592084 ) ) ;
#12381=CARTESIAN_POINT ( 'NONE',  ( 95.54126587499996504, 1.846868145590750077, 7.375000001365592084 ) ) ;
#12391=EDGE_LOOP ( 'NONE', ( #6508, #27570, #1038, #25618 ) ) ;
#12392=CARTESIAN_POINT ( 'NONE',  ( 95.54126587499995082, 1.846868145590750077, 8.625000001365593860 ) ) ;
#12407=CARTESIAN_POINT ( 'NONE',  ( 101.8468681455906903, -4.458734124999987891, 5.750000001365591196 ) ) ;
#12409=CARTESIAN_POINT ( 'NONE',  ( 104.4587341249999639, 1.442382525525748735E-14, 3.187500001365592972 ) ) ;
#12449=ORIENTED_EDGE ( 'NONE', *, *, #23995, .T. ) ;
#12450=CARTESIAN_POINT ( 'NONE',  ( 97.92893218813451028, 5.000000000000018652, 3.937500002731185056 ) ) ;
#12468=CARTESIAN_POINT ( 'NONE',  ( 101.8468681455906903, 4.458734125000016313, 12.12500000136559208 ) ) ;
#12471=DIRECTION ( 'NONE',  ( 1.000000000000000000, 0.000000000000000000, 0.000000000000000000 ) ) ;
#12479=CARTESIAN_POINT ( 'NONE',  ( 99.99999999999995737, 5.000000000000018652, 11.75000000000000000 ) ) ;
#12495=CARTESIAN_POINT ( 'NONE',  ( 99.99999999999995737, -4.999999999999990230, 8.250000000000000000 ) ) ;
#12501=CARTESIAN_POINT ( 'NONE',  ( 96.46446609406721961, 3.535533905932755072, 12.00000000273118594 ) ) ;
#12508=CARTESIAN_POINT ( 'NONE',  ( 103.1528011352953342, -3.152801135295355106, 4.062500001365592084 ) ) ;
#12511=CARTESIAN_POINT ( 'NONE',  ( 98.15313185440923860, 4.458734125000016313, 6.250000001365592084 ) ) ;
#12526=CARTESIAN_POINT ( 'NONE',  ( 103.1528011352953342, 3.152801135295383084, 6.312500001365592084 ) ) ;
#12542=CARTESIAN_POINT ( 'NONE',  ( 95.54126587499995082, -1.846868145590724986, 3.500000001365591196 ) ) ;
#12544=CARTESIAN_POINT ( 'NONE',  ( 95.54126587499996504, -1.846868145590724986, 1.750000001365591862 ) ) ;
#12554=CARTESIAN_POINT ( 'NONE',  ( 103.5355339059327093, -3.535533905932726206, 3.500000002731184612 ) ) ;
#12575=SURFACE_STYLE_USAGE ( .BOTH. , #21582 ) ;
#12578=CARTESIAN_POINT ( 'NONE',  ( 104.9999999999999716, 2.071067811865496822, 13.56250000000000000 ) ) ;
#12590=CLOSED_SHELL ( 'NONE', ( #21509, #4815, #13873, #11621, #27947, #25196, #11759, #18865, #11376, #14861, #4828, #16459, #15246, #18601, #19344, #15768, #15016, #27792, #12957, #21215, #8422, #25684, #28071, #1132, #14362, #27097, #632, #16780, #11978, #15060, #4665, #26009, #23725, #4997, #4912, #17348, #21673, #24684, #1169 ) ) ;
#12591=CARTESIAN_POINT ( 'NONE',  ( 102.0710678118654329, -4.999999999999989342, 2.437500002731185944 ) ) ;
#12600=CARTESIAN_POINT ( 'NONE',  ( 103.5355339059327093, 3.535533905932755072, 9.750000002731184168 ) ) ;
#12610=CARTESIAN_POINT ( 'NONE',  ( 98.15313185440925281, -4.458734124999987891, 12.62500000136559208 ) ) ;
#12629=CARTESIAN_POINT ( 'NONE',  ( 99.99999999999995737, 5.000000000000018652, 7.749999999999999112 ) ) ;
#12636=ORIENTED_EDGE ( 'NONE', *, *, #6900, .T. ) ;
#12638=CARTESIAN_POINT ( 'NONE',  ( 94.99999999999995737, -2.071067811865466624, 6.062499999999999112 ) ) ;
#12641=COLOUR_RGB ( '', 0.09019608, 0.27058824, 0.51372549) ;
#12654=CARTESIAN_POINT ( 'NONE',  ( 103.5355339059327093, -3.535533905932726206, 8.500000002731185944 ) ) ;
#12655=CARTESIAN_POINT ( 'NONE',  ( 98.15313185440925281, -4.458734124999987891, 4.875000001365592084 ) ) ;
#12657=CARTESIAN_POINT ( 'NONE',  ( 104.4587341249999639, 1.442382525525748735E-14, 7.937500001365592084 ) ) ;
#12662=CARTESIAN_POINT ( 'NONE',  ( 94.99999999999995737, 1.387778780781445676E-14, 13.99999999999999822 ) ) ;
#12665=ORIENTED_EDGE ( 'NONE', *, *, #23597, .F. ) ;
#12672=ORIENTED_EDGE ( 'NONE', *, *, #16925, .F. ) ;
#12674=CARTESIAN_POINT ( 'NONE',  ( 98.15313185440925281, -4.458734124999987891, 4.875000001365592084 ) ) ;
#12688=CARTESIAN_POINT ( 'NONE',  ( 99.99999999999995737, 4.458734125000016313, 2.187500001365592084 ) ) ;
#12690=CARTESIAN_POINT ( 'NONE',  ( 104.4587341249999781, -1.846868145590721655, 4.875000001365592084 ) ) ;
#12692=CARTESIAN_POINT ( 'NONE',  ( 99.99999999999995737, -4.458734124999988779, 2.937500001365592528 ) ) ;
#12698=CARTESIAN_POINT ( 'NONE',  ( 104.9999999999999716, 1.449011120738813565E-14, 1.499999999999999556 ) ) ;
#12700=CARTESIAN_POINT ( 'NONE',  ( 94.99999999999995737, 1.387778780781445676E-14, 5.999999999999998224 ) ) ;
#12708=DIRECTION ( 'NONE',  ( -0.000000000000000000, -0.000000000000000000, -1.000000000000000000 ) ) ;
#12720=CARTESIAN_POINT ( 'NONE',  ( 98.15313185440923860, 4.458734125000016313, 14.50000000136559208 ) ) ;
#12726=EDGE_CURVE ( 'NONE', #7831, #11228, #20766, .T. ) ;
#12734=CARTESIAN_POINT ( 'NONE',  ( 96.46446609406721961, -3.535533905932727539, 1.250000002731184390 ) ) ;
#12739=CARTESIAN_POINT ( 'NONE',  ( 95.27063293749995410, 1.387778780781445676E-14, 14.84375000068279604 ) ) ;
#12742=CARTESIAN_POINT ( 'NONE',  ( 97.92893218813451028, 5.000000000000018652, 9.937500002731184168 ) ) ;
#12751=CARTESIAN_POINT ( 'NONE',  ( 96.84719886470459471, 3.152801135295383084, 8.312500001365592084 ) ) ;
#12755=CARTESIAN_POINT ( 'NONE',  ( 96.84719886470459471, 3.152801135295383084, 10.31250000136559208 ) ) ;
#12758=CARTESIAN_POINT ( 'NONE',  ( 92.99999999999995737, 1.387778780781445676E-14, 15.00000000000000000 ) ) ;
#12779=CARTESIAN_POINT ( 'NONE',  ( 104.9999999999999716, 1.449011120738813565E-14, 3.499999999999999556 ) ) ;
#12794=CARTESIAN_POINT ( 'NONE',  ( 101.8468681455906903, 4.458734125000016313, 2.375000001365592084 ) ) ;
#12796=CARTESIAN_POINT ( 'NONE',  ( 95.54126587499996504, -1.846868145590724986, 7.500000001365592084 ) ) ;
#12809=CARTESIAN_POINT ( 'NONE',  ( 98.15313185440925281, 4.458734125000016313, 1.500000001365592972 ) ) ;
#12815=PRODUCT ( 'connector', 'connector', '', ( #19857 ) ) ;
#12822=CARTESIAN_POINT ( 'NONE',  ( 102.0710678118654329, 5.000000000000018652, 9.687499999999998224 ) ) ;
#12823=CARTESIAN_POINT ( 'NONE',  ( 98.15313185440925281, 4.458734125000016313, 14.50000000136559208 ) ) ;
#12825=CARTESIAN_POINT ( 'NONE',  ( 101.8468681455906903, 4.458734125000016313, 4.125000001365592084 ) ) ;
#12830=CARTESIAN_POINT ( 'NONE',  ( 102.0710678118654329, 5.000000000000018652, 7.812500002731185056 ) ) ;
#12833=VERTEX_POINT ( 'NONE', #13239 ) ;
#12854=CARTESIAN_POINT ( 'NONE',  ( 95.54126587499996504, 1.387778780781445676E-14, 11.68750000136559208 ) ) ;
#12866=CARTESIAN_POINT ( 'NONE',  ( 104.9999999999999574, -2.071067811865462627, 2.562500002731185500 ) ) ;
#12882=CARTESIAN_POINT ( 'NONE',  ( 103.1528011352953342, -3.152801135295355106, 8.812500001365592084 ) ) ;
#12886=CARTESIAN_POINT ( 'NONE',  ( 101.8468681455906903, 4.458734125000016313, 10.12500000136559208 ) ) ;
#12908=CARTESIAN_POINT ( 'NONE',  ( 104.9999999999999716, 1.449011120738813565E-14, 4.499999999999999112 ) ) ;
#12926=CARTESIAN_POINT ( 'NONE',  ( 98.15313185440923860, -4.458734124999987891, 0.6250000013655921949 ) ) ;
#12939=ORIENTED_EDGE ( 'NONE', *, *, #21200, .T. ) ;
#12941=CARTESIAN_POINT ( 'NONE',  ( 95.54126587499995082, -1.846868145590724986, 2.750000001365592084 ) ) ;
#12957=ADVANCED_FACE ( 'NONE', ( #7873 ), #5467, .F. ) ;
#12958=CARTESIAN_POINT ( 'NONE',  ( 101.8468681455906903, 4.458734125000016313, 2.125000001365591640 ) ) ;
#12960=CARTESIAN_POINT ( 'NONE',  ( 103.1528011352953342, 3.152801135295383084, 13.06250000136559208 ) ) ;
#12966=CARTESIAN_POINT ( 'NONE',  ( 104.9999999999999574, 2.071067811865501263, 7.687500002731186832 ) ) ;
#12967=EDGE_CURVE ( 'NONE', #5815, #12008, #4954, .T. ) ;
#12977=CARTESIAN_POINT ( 'NONE',  ( 103.1528011352953342, 3.152801135295383084, 14.31250000136559208 ) ) ;
#12990=CARTESIAN_POINT ( 'NONE',  ( 95.54126587499996504, 1.846868145590750077, 10.62500000136559208 ) ) ;
#13003=CARTESIAN_POINT ( 'NONE',  ( 96.46446609406721961, -3.535533905932727539, 2.250000002731185500 ) ) ;
#13007=DIRECTION ( 'NONE',  ( -1.000000000000000000, 0.000000000000000000, 0.000000000000000000 ) ) ;
#13008=FILL_AREA_STYLE_COLOUR ( '', #2873 ) ;
#13021=LINE ( 'NONE', #10619, #15432 ) ;
#13022=CARTESIAN_POINT ( 'NONE',  ( 99.99999999999995737, -4.458734124999988779, 7.687500001365592084 ) ) ;
#13025=CARTESIAN_POINT ( 'NONE',  ( 96.84719886470459471, -3.152801135295355994, 12.56250000136559208 ) ) ;
#13035=DIRECTION ( 'NONE',  ( 1.000000000000000000, 0.000000000000000000, 0.000000000000000000 ) ) ;
#13048=CARTESIAN_POINT ( 'NONE',  ( 97.92893218813451028, -4.999999999999989342, 7.187499999999999112 ) ) ;
#13064=( BOUNDED_CURVE ( )  B_SPLINE_CURVE ( 2, ( #26788, #13781, #2968, #26644, #2699, #22793, #15791, #26933, #7376 ),
 .UNSPECIFIED., .F., .F. ) 
 B_SPLINE_CURVE_WITH_KNOTS ( ( 3, 2, 2, 2, 3 ),
 ( 0.6785714285714284921, 0.6874999999999998890, 0.6964285714285712858, 0.7053571428571427937, 0.7142857142857141906 ),
 .UNSPECIFIED. ) 
 CURVE ( )  GEOMETRIC_REPRESENTATION_ITEM ( )  RATIONAL_B_SPLINE_CURVE ( ( 1.000000000000000888, 0.9238795325112857393, 1.000000000000000000, 0.9238795325112867385, 1.000000000000000000, 0.9238795325112867385, 1.000000000000000000, 0.9238795325112877377, 0.9999999999999990008 ) ) 
 REPRESENTATION_ITEM ( '' )  );
#13065=CARTESIAN_POINT ( 'NONE',  ( 98.15313185440923860, 4.458734125000016313, 3.250000001365592972 ) ) ;
#13082=CARTESIAN_POINT ( 'NONE',  ( 101.8468681455906903, 4.458734125000016313, 1.375000001365592972 ) ) ;
#13083=ORIENTED_EDGE ( 'NONE', *, *, #21558, .T. ) ;
#13095=CARTESIAN_POINT ( 'NONE',  ( 95.54126587499995082, 1.846868145590750077, 12.62500000136559208 ) ) ;
#13097=CARTESIAN_POINT ( 'NONE',  ( 99.99999999999995737, -4.458734124999988779, 12.68750000136559208 ) ) ;
#13106=VERTEX_POINT ( 'NONE', #27800 ) ;
#13117=CARTESIAN_POINT ( 'NONE',  ( 104.4587341249999781, 1.846868145590750299, 13.25000000136559208 ) ) ;
#13134=CARTESIAN_POINT ( 'NONE',  ( 96.84719886470459471, 3.152801135295383084, 12.56250000136559208 ) ) ;
#13148=CARTESIAN_POINT ( 'NONE',  ( 95.54126587499995082, 1.846868145590750077, 14.37500000136559386 ) ) ;
#13154=DIRECTION ( 'NONE',  ( 0.000000000000000000, 0.000000000000000000, 1.000000000000000000 ) ) ;
#13164=CARTESIAN_POINT ( 'NONE',  ( 96.84719886470459471, -3.152801135295355994, 8.562500001365592084 ) ) ;
#13165=ORIENTED_EDGE ( 'NONE', *, *, #21540, .F. ) ;
#13167=CARTESIAN_POINT ( 'NONE',  ( 104.4587341249999639, 1.442382525525748735E-14, 13.93750000136559208 ) ) ;
#13191=CARTESIAN_POINT ( 'NONE',  ( 94.99999999999995737, 2.071067811865491048, 4.937500000000000888 ) ) ;
#13210=CARTESIAN_POINT ( 'NONE',  ( 96.84719886470459471, -3.152801135295355994, 1.562500001365591418 ) ) ;
#13218=AXIS2_PLACEMENT_3D ( 'NONE', #9615, #16167, #514 ) ;
#13226=CARTESIAN_POINT ( 'NONE',  ( 95.54126587499995082, 1.846868145590750077, 4.625000001365592084 ) ) ;
#13239=CARTESIAN_POINT ( 'NONE',  ( 94.99999999999995737, 1.387778780781445676E-14, 8.000000000000000000 ) ) ;
#13240=CARTESIAN_POINT ( 'NONE',  ( 104.4587341249999781, -1.846868145590721655, 12.12500000136559208 ) ) ;
#13242=CARTESIAN_POINT ( 'NONE',  ( 103.1528011352953342, -3.152801135295355106, 1.812500001365591640 ) ) ;
#13245=DIRECTION ( 'NONE',  ( -0.000000000000000000, -0.000000000000000000, -1.000000000000000000 ) ) ;
#13255=CARTESIAN_POINT ( 'NONE',  ( 102.0710678118654329, -4.999999999999989342, 7.437500002731187720 ) ) ;
#13257=CARTESIAN_POINT ( 'NONE',  ( 96.84719886470459471, -3.152801135295355994, 13.81250000136559208 ) ) ;
#13271=EDGE_LOOP ( 'NONE', ( #929, #12939 ) ) ;
#13275=CARTESIAN_POINT ( 'NONE',  ( 95.54126587499996504, -1.846868145590724986, 9.750000001365593860 ) ) ;
#13281=CARTESIAN_POINT ( 'NONE',  ( 94.99999999999995737, 1.387778780781445676E-14, 34.79898987322334136 ) ) ;
#13308=CARTESIAN_POINT ( 'NONE',  ( 103.1528011352953342, 3.152801135295383084, 8.062500001365592084 ) ) ;
#13311=CARTESIAN_POINT ( 'NONE',  ( 98.15313185440925281, -4.458734124999987891, 13.62500000136559208 ) ) ;
#13332=CARTESIAN_POINT ( 'NONE',  ( 102.0710678118654329, 5.000000000000018652, 7.812500002731185056 ) ) ;
#13355=CARTESIAN_POINT ( 'NONE',  ( 99.99999999999995737, -4.458734124999988779, 2.687500001365592528 ) ) ;
#13358=CARTESIAN_POINT ( 'NONE',  ( 104.9999999999999716, 1.449011120738813565E-14, 4.499999999999999112 ) ) ;
#13371=CARTESIAN_POINT ( 'NONE',  ( 104.9999999999999574, -2.071067811865462627, 13.43749999999999822 ) ) ;
#13385=CARTESIAN_POINT ( 'NONE',  ( 101.8468681455906903, 4.458734125000016313, 12.37500000136559208 ) ) ;
#13388=CARTESIAN_POINT ( 'NONE',  ( 98.15313185440923860, 4.458734125000016313, 12.25000000136559208 ) ) ;
#13390=CARTESIAN_POINT ( 'NONE',  ( 95.54126587499996504, 1.387778780781445676E-14, 0.6875000013655923059 ) ) ;
#13397=CARTESIAN_POINT ( 'NONE',  ( 99.99999999999995737, -4.999999999999990230, 12.37500000273118594 ) ) ;
#13402=FACE_OUTER_BOUND ( 'NONE', #6222, .T. ) ;
#13420=CARTESIAN_POINT ( 'NONE',  ( 99.99999999999995737, 4.458734125000016313, 12.43750000136559208 ) ) ;
#13440=( LENGTH_UNIT ( ) NAMED_UNIT ( * ) SI_UNIT ( .MILLI., .METRE. ) );
#13441=CARTESIAN_POINT ( 'NONE',  ( 94.99999999999997158, -2.071067811865486608, 1.187500002731185722 ) ) ;
#13449=CARTESIAN_POINT ( 'NONE',  ( 103.1528011352953342, 3.152801135295383084, 4.062500001365592084 ) ) ;
#13453=CARTESIAN_POINT ( 'NONE',  ( 99.99999999999995737, 4.458734125000016313, 9.187500001365592084 ) ) ;
#13472=CARTESIAN_POINT ( 'NONE',  ( 103.5355339059327093, -3.535533905932726206, 8.500000002731185944 ) ) ;
#13476=EDGE_CURVE ( 'NONE', #20673, #949, #7095, .T. ) ;
#13477=VERTEX_POINT ( 'NONE', #6234 ) ;
#13481=CARTESIAN_POINT ( 'NONE',  ( 104.9999999999999574, 2.071067811865491937, 1.562499999999999556 ) ) ;
#13485=CARTESIAN_POINT ( 'NONE',  ( 99.99999999999995737, 5.000000000000018652, 5.875000002731185056 ) ) ;
#13503=CARTESIAN_POINT ( 'NONE',  ( 103.1528011352953342, 3.152801135295383084, 1.062500001365592528 ) ) ;
#13506=CARTESIAN_POINT ( 'NONE',  ( 99.99999999999995737, 5.000000000000018652, 4.749999999999999112 ) ) ;
#13523=CARTESIAN_POINT ( 'NONE',  ( 104.9999999999999574, 2.071067811865491937, 12.56249999999999822 ) ) ;
#13532=CYLINDRICAL_SURFACE ( 'NONE', #9954, 5.000000000000004441 ) ;
#13536=CARTESIAN_POINT ( 'NONE',  ( 98.15313185440925281, 4.458734125000016313, 9.500000001365593860 ) ) ;
#13538=CARTESIAN_POINT ( 'NONE',  ( 104.4587341249999639, 1.442382525525748735E-14, 0.9375000013655925279 ) ) ;
#13541=DIRECTION ( 'NONE',  ( -1.000000000000000000, 0.000000000000000000, 0.000000000000000000 ) ) ;
#13548=CARTESIAN_POINT ( 'NONE',  ( 104.9999999999999858, -2.071067811865442643, 1.437500000000000444 ) ) ;
#13552=CARTESIAN_POINT ( 'NONE',  ( 95.54126587499995082, -1.846868145590724986, 9.750000001365593860 ) ) ;
#13568=CARTESIAN_POINT ( 'NONE',  ( 99.99999999999995737, -4.458734124999988779, 6.937500001365592972 ) ) ;
#13588=DIRECTION ( 'NONE',  ( -0.000000000000000000, -0.000000000000000000, -1.000000000000000000 ) ) ;
#13598=CARTESIAN_POINT ( 'NONE',  ( 98.15313185440925281, -4.458734124999987891, 5.625000001365591196 ) ) ;
#13601=CARTESIAN_POINT ( 'NONE',  ( 98.15313185440925281, -4.458734124999987891, 6.625000001365592084 ) ) ;
#13605=FACE_OUTER_BOUND ( 'NONE', #8689, .T. ) ;
#13615=CARTESIAN_POINT ( 'NONE',  ( 96.46446609406721961, -3.535533905932727539, 8.125000000000000000 ) ) ;
#13618=( BOUNDED_CURVE ( )  B_SPLINE_CURVE ( 2, ( #22545, #24534, #17975, #20407, #13684, #22401, #18266, #7417, #26972 ),
 .UNSPECIFIED., .F., .F. ) 
 B_SPLINE_CURVE_WITH_KNOTS ( ( 3, 2, 2, 2, 3 ),
 ( 0.7857142857142856984, 0.7946428571428570953, 0.8035714285714286031, 0.8125000000000000000, 0.8214285714285713969 ),
 .UNSPECIFIED. ) 
 CURVE ( )  GEOMETRIC_REPRESENTATION_ITEM ( )  RATIONAL_B_SPLINE_CURVE ( ( 1.000000000000000000, 0.9238795325112867385, 1.000000000000000000, 0.9238795325112867385, 1.000000000000000000, 0.9238795325112867385, 1.000000000000000000, 0.9238795325112867385, 1.000000000000000000 ) ) 
 REPRESENTATION_ITEM ( '' )  );
#13619=CARTESIAN_POINT ( 'NONE',  ( 97.92893218813451028, 5.000000000000018652, 10.93750000273118594 ) ) ;
#13649=LINE ( 'NONE', #3125, #21232 ) ;
#13664=CARTESIAN_POINT ( 'NONE',  ( 104.9999999999999716, 1.449011120738813565E-14, 6.499999999999999112 ) ) ;
#13665=CARTESIAN_POINT ( 'NONE',  ( 99.99999999999995737, 5.000000000000018652, 14.75000000000000000 ) ) ;
#13671=CYLINDRICAL_SURFACE ( 'NONE', #11195, 5.000000000000004441 ) ;
#13679=CARTESIAN_POINT ( 'NONE',  ( 99.99999999999995737, 4.458734125000016313, 9.437500001365593860 ) ) ;
#13681=CARTESIAN_POINT ( 'NONE',  ( 104.4587341249999639, 1.442382525525748735E-14, 11.93750000136559208 ) ) ;
#13684=CARTESIAN_POINT ( 'NONE',  ( 99.99999999999995737, 5.000000000000018652, 3.750000000000000000 ) ) ;
#13696=CARTESIAN_POINT ( 'NONE',  ( 95.54126587499996504, 1.387778780781445676E-14, 11.68750000136559208 ) ) ;
#13711=CARTESIAN_POINT ( 'NONE',  ( 98.15313185440923860, 4.458734125000016313, 8.500000001365592084 ) ) ;
#13715=CARTESIAN_POINT ( 'NONE',  ( 99.99999999999995737, -4.999999999999990230, 14.24999999999999822 ) ) ;
#13718=CARTESIAN_POINT ( 'NONE',  ( 94.99999999999995737, 1.387778780781445676E-14, 12.00000000000000000 ) ) ;
#13730=CARTESIAN_POINT ( 'NONE',  ( 96.46446609406721961, 3.535533905932755072, 9.000000002731184168 ) ) ;
#13734=CARTESIAN_POINT ( 'NONE',  ( 96.46446609406721961, -3.535533905932727539, 2.250000002731185500 ) ) ;
#13738=CARTESIAN_POINT ( 'NONE',  ( 98.15313185440925281, -4.458734124999987891, 4.625000001365592084 ) ) ;
#13741=CARTESIAN_POINT ( 'NONE',  ( 99.99999999999995737, -4.458734124999988779, 6.687500001365592084 ) ) ;
#13744=DIRECTION ( 'NONE',  ( -0.000000000000000000, -0.000000000000000000, -1.000000000000000000 ) ) ;
#13746=CARTESIAN_POINT ( 'NONE',  ( 102.0710678118654329, -4.999999999999989342, 5.312499999999999112 ) ) ;
#13753=ORIENTED_EDGE ( 'NONE', *, *, #27289, .F. ) ;
#13757=CARTESIAN_POINT ( 'NONE',  ( 96.46446609406721961, 3.535533905932755072, 8.000000002731185944 ) ) ;
#13764=CARTESIAN_POINT ( 'NONE',  ( 94.99999999999995737, 1.387778780781445676E-14, 0.9999999999999991118 ) ) ;
#13781=CARTESIAN_POINT ( 'NONE',  ( 104.9999999999999858, -2.071067811865442643, 4.562500002731185944 ) ) ;
#13802=CARTESIAN_POINT ( 'NONE',  ( 94.99999999999995737, 2.071067811865491048, 12.93749999999999822 ) ) ;
#13810=CARTESIAN_POINT ( 'NONE',  ( 104.9999999999999716, -2.071067811865462627, 3.437499999999999556 ) ) ;
#13816=CARTESIAN_POINT ( 'NONE',  ( 99.99999999999995737, 4.458734125000016313, 5.437500001365592972 ) ) ;
#13818=CARTESIAN_POINT ( 'NONE',  ( 96.84719886470459471, 3.152801135295383084, 10.31250000136559208 ) ) ;
#13833=CARTESIAN_POINT ( 'NONE',  ( 99.99999999999995737, -4.458734124999988779, 10.93750000136559208 ) ) ;
#13850=CARTESIAN_POINT ( 'NONE',  ( 96.84719886470459471, -3.152801135295355994, 8.812500001365592084 ) ) ;
#13870=CARTESIAN_POINT ( 'NONE',  ( 103.5355339059327093, -3.535533905932726206, 13.37500000000000000 ) ) ;
#13873=ADVANCED_FACE ( 'NONE', ( #10456 ), #25578, .F. ) ;
#13877=CYLINDRICAL_SURFACE ( 'NONE', #14149, 5.000000000000004441 ) ;
#13882=CARTESIAN_POINT ( 'NONE',  ( 104.4587341249999781, 1.846868145590750299, 6.000000001365591196 ) ) ;
#13885=CARTESIAN_POINT ( 'NONE',  ( 101.8468681455906903, 4.458734125000016313, 6.125000001365591196 ) ) ;
#13901=CARTESIAN_POINT ( 'NONE',  ( 96.46446609406721961, -3.535533905932727539, 11.25000000273118594 ) ) ;
#13907=CARTESIAN_POINT ( 'NONE',  ( 97.92893218813451028, -4.999999999999989342, 3.187499999999999556 ) ) ;
#13917=CARTESIAN_POINT ( 'NONE',  ( 104.9999999999999716, 1.449011120738813565E-14, 2.625000002731185500 ) ) ;
#13937=VECTOR ( 'NONE', #12283, 1000.000000000000000 ) ;
#13945=CARTESIAN_POINT ( 'NONE',  ( 104.9999999999999716, 1.449011120738813565E-14, 12.49999999999999822 ) ) ;
#13954=CARTESIAN_POINT ( 'NONE',  ( 99.99999999999995737, 1.387778780781445676E-14, 34.79898987322334136 ) ) ;
#13959=CARTESIAN_POINT ( 'NONE',  ( 98.15313185440925281, 4.458734125000016313, 6.500000001365592084 ) ) ;
#13962=CARTESIAN_POINT ( 'NONE',  ( 104.4587341249999781, 1.846868145590750521, 12.00000000136559208 ) ) ;
#13973=LINE ( 'NONE', #3168, #5370 ) ;
#13974=CARTESIAN_POINT ( 'NONE',  ( 96.84719886470459471, 3.152801135295383084, 12.56250000136559208 ) ) ;
#13992=CARTESIAN_POINT ( 'NONE',  ( 103.1528011352953342, 3.152801135295383084, 7.312500001365592084 ) ) ;
#13996=CARTESIAN_POINT ( 'NONE',  ( 104.9999999999999716, 2.071067811865491937, 6.687500002731185056 ) ) ;
#14015=CARTESIAN_POINT ( 'NONE',  ( 104.9999999999999574, 2.071067811865501263, 10.68750000273118594 ) ) ;
#14018=CARTESIAN_POINT ( 'NONE',  ( 103.5355339059327093, -3.535533905932726206, 1.500000002731184612 ) ) ;
#14025=CARTESIAN_POINT ( 'NONE',  ( 104.4587341249999781, 1.846868145590750299, 5.000000001365592972 ) ) ;
#14028=CARTESIAN_POINT ( 'NONE',  ( 98.15313185440925281, 4.458734125000016313, 9.250000001365593860 ) ) ;
#14048=CARTESIAN_POINT ( 'NONE',  ( 97.92893218813451028, -4.999999999999989342, 7.312500002731185944 ) ) ;
#14052=CARTESIAN_POINT ( 'NONE',  ( 94.99999999999995737, 1.387778780781445676E-14, 15.00000000000000000 ) ) ;
#14074=CARTESIAN_POINT ( 'NONE',  ( 104.9999999999999716, 1.449011120738813565E-14, 34.79898987322334136 ) ) ;
#14094=CARTESIAN_POINT ( 'NONE',  ( 102.0710678118654329, 5.000000000000018652, 10.68749999999999822 ) ) ;
#14099=DIRECTION ( 'NONE',  ( 0.000000000000000000, -0.000000000000000000, 1.000000000000000000 ) ) ;
#14106=CARTESIAN_POINT ( 'NONE',  ( 104.4587341249999781, -1.846868145590721655, 7.125000001365592084 ) ) ;
#14108=CARTESIAN_POINT ( 'NONE',  ( 101.8468681455907046, -4.458734124999987891, 8.750000001365592084 ) ) ;
#14111=CARTESIAN_POINT ( 'NONE',  ( 99.99999999999995737, -4.999999999999990230, 9.250000000000000000 ) ) ;
#14118=( BOUNDED_CURVE ( )  B_SPLINE_CURVE ( 2, ( #7163, #24853, #15859, #24568, #13715, #22436, #2904, #777, #12662 ),
 .UNSPECIFIED., .F., .T. ) 
 B_SPLINE_CURVE_WITH_KNOTS ( ( 3, 2, 2, 2, 3 ),
 ( 0.03571428571428574700, 0.04464285714285718548, 0.05357142857142861703, 0.06250000000000005551, 0.07142857142857149400 ),
 .UNSPECIFIED. ) 
 CURVE ( )  GEOMETRIC_REPRESENTATION_ITEM ( )  RATIONAL_B_SPLINE_CURVE ( ( 0.9999999999999996669, 0.9238795325112870716, 1.000000000000000000, 0.9238795325112867385, 1.000000000000000000, 0.9238795325112867385, 1.000000000000000000, 0.9238795325112861834, 1.000000000000000666 ) ) 
 REPRESENTATION_ITEM ( '' )  );
#14121=CARTESIAN_POINT ( 'NONE',  ( 96.84719886470459471, 3.152801135295383084, 6.562500001365592084 ) ) ;
#14136=DIRECTION ( 'NONE',  ( -0.000000000000000000, -0.000000000000000000, -1.000000000000000000 ) ) ;
#14137=CARTESIAN_POINT ( 'NONE',  ( 96.84719886470459471, -3.152801135295355994, 7.812500001365592084 ) ) ;
#14141=FACE_OUTER_BOUND ( 'NONE', #7443, .T. ) ;
#14149=AXIS2_PLACEMENT_3D ( 'NONE', #9472, #18173, #26886 ) ;
#14154=CARTESIAN_POINT ( 'NONE',  ( 104.9999999999999858, -2.071067811865442643, 0.5625000027311864992 ) ) ;
#14160=DIRECTION ( 'NONE',  ( -1.000000000000000000, 0.000000000000000000, 0.000000000000000000 ) ) ;
#14170=CARTESIAN_POINT ( 'NONE',  ( 95.54126587499995082, -1.846868145590724986, 0.5000000013655920839 ) ) ;
#14176=CARTESIAN_POINT ( 'NONE',  ( 104.9999999999999858, -2.071067811865442643, 5.437500000000001776 ) ) ;
#14187=CARTESIAN_POINT ( 'NONE',  ( 94.99999999999995737, 2.071067811865491048, 4.062500002731185056 ) ) ;
#14203=CARTESIAN_POINT ( 'NONE',  ( 96.84719886470459471, -3.152801135295355994, 13.56250000136559208 ) ) ;
#14233=CARTESIAN_POINT ( 'NONE',  ( 96.46446609406721961, 3.535533905932755072, 8.875000000000000000 ) ) ;
#14239=CARTESIAN_POINT ( 'NONE',  ( 103.5355339059327093, 3.535533905932755072, 12.75000000273118594 ) ) ;
#14241=FACE_OUTER_BOUND ( 'NONE', #22438, .T. ) ;
#14247=CARTESIAN_POINT ( 'NONE',  ( 98.15313185440925281, 4.458734125000016313, 7.500000001365592084 ) ) ;
#14249=CARTESIAN_POINT ( 'NONE',  ( 98.15313185440923860, -4.458734124999987891, 10.62500000136559208 ) ) ;
#14263=CARTESIAN_POINT ( 'NONE',  ( 96.84719886470459471, 3.152801135295383084, 8.562500001365592084 ) ) ;
#14276=CARTESIAN_POINT ( 'NONE',  ( 99.99999999999995737, 4.458734125000016313, 3.437500001365592972 ) ) ;
#14280=DIRECTION ( 'NONE',  ( -0.000000000000000000, -0.000000000000000000, -1.000000000000000000 ) ) ;
#14284=( BOUNDED_CURVE ( )  B_SPLINE_CURVE ( 2, ( #14052, #3101, #22773, #11340, #9642, #7502, #26626, #1114, #16196 ),
 .UNSPECIFIED., .F., .T. ) 
 B_SPLINE_CURVE_WITH_KNOTS ( ( 3, 2, 2, 2, 3 ),
 ( 0.000000000000000000, 0.008928571428571436749, 0.01785714285714287350, 0.02678571428571431198, 0.03571428571428574700 ),
 .UNSPECIFIED. ) 
 CURVE ( )  GEOMETRIC_REPRESENTATION_ITEM ( )  RATIONAL_B_SPLINE_CURVE ( ( 1.000000000000000000, 0.9238795325112867385, 1.000000000000000000, 0.9238795325112867385, 1.000000000000000000, 0.9238795325112867385, 1.000000000000000000, 0.9238795325112864054, 1.000000000000000222 ) ) 
 REPRESENTATION_ITEM ( '' )  );
#14295=LINE ( 'NONE', #4045, #3029 ) ;
#14299=CARTESIAN_POINT ( 'NONE',  ( 94.99999999999995737, 1.387778780781445676E-14, 2.999999999999999112 ) ) ;
#14304=ORIENTED_EDGE ( 'NONE', *, *, #28137, .F. ) ;
#14305=CARTESIAN_POINT ( 'NONE',  ( 99.99999999999995737, -4.458734124999988779, 1.687500001365591418 ) ) ;
#14314=DIRECTION ( 'NONE',  ( -0.000000000000000000, -0.000000000000000000, -1.000000000000000000 ) ) ;
#14322=CARTESIAN_POINT ( 'NONE',  ( 94.99999999999995737, 1.387778780781445676E-14, 5.125000002731184168 ) ) ;
#14341=CARTESIAN_POINT ( 'NONE',  ( 96.84719886470459471, 3.152801135295383084, 12.31250000136559208 ) ) ;
#14350=CARTESIAN_POINT ( 'NONE',  ( 104.9999999999999716, 1.449011120738813565E-14, 2.499999999999998668 ) ) ;
#14361=CARTESIAN_POINT ( 'NONE',  ( 104.9999999999999716, 1.449011120738813565E-14, 7.500000000000000000 ) ) ;
#14362=ADVANCED_FACE ( 'NONE', ( #13402 ), #11270, .F. ) ;
#14371=CARTESIAN_POINT ( 'NONE',  ( 99.99999999999995737, 5.000000000000018652, 9.749999999999998224 ) ) ;
#14377=CARTESIAN_POINT ( 'NONE',  ( 94.99999999999995737, -2.071067811865466624, 13.18750000273118594 ) ) ;
#14380=CARTESIAN_POINT ( 'NONE',  ( 97.92893218813451028, 5.000000000000018652, 11.93750000273118950 ) ) ;
#14386=CARTESIAN_POINT ( 'NONE',  ( 103.1528011352953342, -3.152801135295355106, 9.062500001365592084 ) ) ;
#14388=CARTESIAN_POINT ( 'NONE',  ( 96.84719886470459471, 3.152801135295383084, 5.312500001365592972 ) ) ;
#14392=CARTESIAN_POINT ( 'NONE',  ( 94.99999999999995737, -2.071067811865466624, 9.062500000000000000 ) ) ;
#14399=EDGE_CURVE ( 'NONE', #24537, #2527, #13973, .T. ) ;
#14403=CARTESIAN_POINT ( 'NONE',  ( 101.8468681455906903, 4.458734125000016313, 8.375000001365592084 ) ) ;
#14418=CARTESIAN_POINT ( 'NONE',  ( 98.15313185440923860, -4.458734124999987891, 2.875000001365592528 ) ) ;
#14441=AXIS2_PLACEMENT_3D ( 'NONE', #19698, #8866, #17558 ) ;
#14446=ORIENTED_EDGE ( 'NONE', *, *, #2887, .T. ) ;
#14447=CARTESIAN_POINT ( 'NONE',  ( 96.84719886470459471, 3.152801135295383084, 14.56250000136559208 ) ) ;
#14448=CARTESIAN_POINT ( 'NONE',  ( 96.84719886470459471, 3.152801135295383084, 13.56250000136559386 ) ) ;
#14464=CARTESIAN_POINT ( 'NONE',  ( 97.92893218813451028, -4.999999999999989342, 4.312500002731185056 ) ) ;
#14483=DIRECTION ( 'NONE',  ( -0.000000000000000000, -0.000000000000000000, -1.000000000000000000 ) ) ;
#14484=CARTESIAN_POINT ( 'NONE',  ( 95.54126587499996504, 1.387778780781445676E-14, 14.43750000136559208 ) ) ;
#14509=CARTESIAN_POINT ( 'NONE',  ( 94.99999999999995737, 2.071067811865491048, 8.937500000000000000 ) ) ;
#14510=CARTESIAN_POINT ( 'NONE',  ( 94.99999999999997158, 2.071067811865471953, 1.937500000000000888 ) ) ;
#14514=CARTESIAN_POINT ( 'NONE',  ( 104.9999999999999716, 1.449011120738813565E-14, 13.62500000273118417 ) ) ;
#14525=CARTESIAN_POINT ( 'NONE',  ( 95.54126587499995082, 1.846868145590750077, 1.625000001365592972 ) ) ;
#14527=CARTESIAN_POINT ( 'NONE',  ( 99.99999999999995737, -4.458734124999988779, 7.687500001365592084 ) ) ;
#14538=ORIENTED_EDGE ( 'NONE', *, *, #80, .T. ) ;
#14542=CARTESIAN_POINT ( 'NONE',  ( 95.54126587499995082, 1.846868145590750077, 6.625000001365592084 ) ) ;
#14556=EDGE_CURVE ( 'NONE', #13477, #22034, #8406, .T. ) ;
#14558=CARTESIAN_POINT ( 'NONE',  ( 103.1528011352953342, -3.152801135295355106, 2.812500001365592528 ) ) ;
#14559=CARTESIAN_POINT ( 'NONE',  ( 94.99999999999997158, 2.071067811865471953, 4.062500002731185944 ) ) ;
#14560=CARTESIAN_POINT ( 'NONE',  ( 101.8468681455907046, 4.458734125000016313, 3.375000001365592972 ) ) ;
#14576=CARTESIAN_POINT ( 'NONE',  ( 99.99999999999995737, 5.000000000000018652, 1.875000002731185056 ) ) ;
#14586=CARTESIAN_POINT ( 'NONE',  ( 104.4587341249999781, -1.846868145590721655, 13.12500000136559208 ) ) ;
#14600=CARTESIAN_POINT ( 'NONE',  ( 104.9999999999999574, -2.071067811865462627, 4.562500002731185944 ) ) ;
#14604=DIRECTION ( 'NONE',  ( -1.000000000000000000, 0.000000000000000000, 0.000000000000000000 ) ) ;
#14616=CARTESIAN_POINT ( 'NONE',  ( 95.54126587499996504, 1.387778780781445676E-14, 11.43750000136559208 ) ) ;
#14634=EDGE_CURVE ( 'NONE', #27806, #7689, #25658, .T. ) ;
#14642=CARTESIAN_POINT ( 'NONE',  ( 104.9999999999999716, 1.449011120738813565E-14, 8.499999999999998224 ) ) ;
#14646=CARTESIAN_POINT ( 'NONE',  ( 102.0710678118654329, 5.000000000000018652, 13.81250000273118950 ) ) ;
#14655=CARTESIAN_POINT ( 'NONE',  ( 99.99999999999995737, -4.458734124999988779, 1.937500001365591640 ) ) ;
#14657=CARTESIAN_POINT ( 'NONE',  ( 96.84719886470459471, -3.152801135295355994, 7.562500001365592084 ) ) ;
#14666=VERTEX_POINT ( 'NONE', #13664 ) ;
#14667=VECTOR ( 'NONE', #20652, 1000.000000000000000 ) ;
#14671=CARTESIAN_POINT ( 'NONE',  ( 104.4587341249999781, 1.846868145590750299, 7.250000001365591196 ) ) ;
#14681=ORIENTED_EDGE ( 'NONE', *, *, #24668, .F. ) ;
#14687=CARTESIAN_POINT ( 'NONE',  ( 95.54126587499995082, 1.846868145590750077, 5.375000001365592972 ) ) ;
#14689=CARTESIAN_POINT ( 'NONE',  ( 104.4587341249999781, -1.846868145590721655, 4.125000001365592084 ) ) ;
#14709=ORIENTED_EDGE ( 'NONE', *, *, #19574, .F. ) ;
#14710=CARTESIAN_POINT ( 'NONE',  ( 103.5355339059327093, 3.535533905932755072, 1.750000002731184834 ) ) ;
#14715=CARTESIAN_POINT ( 'NONE',  ( 94.99999999999995737, 1.387778780781445676E-14, 34.79898987322334136 ) ) ;
#14734=CARTESIAN_POINT ( 'NONE',  ( 97.92893218813451028, -4.999999999999989342, 2.312500002731185500 ) ) ;
#14740=CARTESIAN_POINT ( 'NONE',  ( 99.99999999999995737, 1.387778780781445676E-14, 34.79898987322334136 ) ) ;
#14751=CARTESIAN_POINT ( 'NONE',  ( 104.9999999999999858, 2.071067811865486608, 12.56249999999999645 ) ) ;
#14752=CARTESIAN_POINT ( 'NONE',  ( 96.46446609406721961, -3.535533905932727539, 13.25000000273118417 ) ) ;
#14758=CARTESIAN_POINT ( 'NONE',  ( 97.92893218813451028, 5.000000000000018652, 2.937500002731185944 ) ) ;
#14777=CARTESIAN_POINT ( 'NONE',  ( 102.0710678118654329, -4.999999999999989342, 3.312499999999999556 ) ) ;
#14790=CARTESIAN_POINT ( 'NONE',  ( 99.99999999999995737, -4.458734124999988779, 3.937500001365591640 ) ) ;
#14792=CARTESIAN_POINT ( 'NONE',  ( 104.4587341249999639, 1.442382525525748735E-14, 5.937500001365592084 ) ) ;
#14806=CARTESIAN_POINT ( 'NONE',  ( 104.9999999999999716, 1.449011120738813565E-14, 34.79898987322334136 ) ) ;
#14807=CARTESIAN_POINT ( 'NONE',  ( 104.4587341249999639, 1.442382525525748735E-14, 4.187500001365592084 ) ) ;
#14819=VERTEX_POINT ( 'NONE', #24089 ) ;
#14824=CARTESIAN_POINT ( 'NONE',  ( 104.4587341249999639, 1.442382525525748735E-14, 3.937500001365591640 ) ) ;
#14826=CARTESIAN_POINT ( 'NONE',  ( 95.54126587499996504, 1.846868145590750077, 2.625000001365592084 ) ) ;
#14829=CARTESIAN_POINT ( 'NONE',  ( 103.5355339059327093, 3.535533905932755072, 7.750000002731185056 ) ) ;
#14850=( BOUNDED_CURVE ( )  B_SPLINE_CURVE ( 2, ( #11121, #19835, #6857, #4738, #13397, #8113, #26058, #21651, #17362 ),
 .UNSPECIFIED., .F., .T. ) 
 B_SPLINE_CURVE_WITH_KNOTS ( ( 3, 2, 2, 2, 3 ),
 ( 0.1071428571428571092, 0.1160714285714285476, 0.1249999999999999861, 0.1339285714285714246, 0.1428571428571428492 ),
 .UNSPECIFIED. ) 
 CURVE ( )  GEOMETRIC_REPRESENTATION_ITEM ( )  RATIONAL_B_SPLINE_CURVE ( ( 1.000000000000000222, 0.9238795325112865164, 1.000000000000000000, 0.9238795325112867385, 1.000000000000000000, 0.9238795325112867385, 1.000000000000000000, 0.9238795325112867385, 1.000000000000000000 ) ) 
 REPRESENTATION_ITEM ( '' )  );
#14856=ORIENTED_EDGE ( 'NONE', *, *, #6887, .F. ) ;
#14861=ADVANCED_FACE ( 'NONE', ( #27092 ), #9544, .F. ) ;
#14866=DIRECTION ( 'NONE',  ( -0.000000000000000000, -0.000000000000000000, -1.000000000000000000 ) ) ;
#14868=DIRECTION ( 'NONE',  ( -0.000000000000000000, -0.000000000000000000, -1.000000000000000000 ) ) ;
#14871=EDGE_CURVE ( 'NONE', #26423, #27592, #22269, .T. ) ;
#14875=CARTESIAN_POINT ( 'NONE',  ( 102.0710678118654329, -4.999999999999989342, 0.4375000027311854445 ) ) ;
#14882=CARTESIAN_POINT ( 'NONE',  ( 99.99999999999995737, 5.000000000000018652, 9.875000002731185944 ) ) ;
#14888=CARTESIAN_POINT ( 'NONE',  ( 103.5355339059327093, -3.535533905932726206, 10.37499999999999822 ) ) ;
#14890=CARTESIAN_POINT ( 'NONE',  ( 98.15313185440925281, 4.458734125000016313, 9.250000001365593860 ) ) ;
#14893=CARTESIAN_POINT ( 'NONE',  ( 103.1528011352953342, 3.152801135295383084, 11.06250000136559208 ) ) ;
#14903=CARTESIAN_POINT ( 'NONE',  ( 95.27063293749995410, 1.387778780781445676E-14, 14.28125000204838813 ) ) ;
#14917=CARTESIAN_POINT ( 'NONE',  ( 97.92893218813451028, -4.999999999999989342, 5.187500000000000888 ) ) ;
#14926=CARTESIAN_POINT ( 'NONE',  ( 97.92893218813451028, 5.000000000000018652, 4.937500002731185944 ) ) ;
#14932=CARTESIAN_POINT ( 'NONE',  ( 101.8468681455906903, -4.458734124999987891, 4.000000001365592084 ) ) ;
#14934=CARTESIAN_POINT ( 'NONE',  ( 103.1528011352953342, 3.152801135295383084, 6.062500001365592084 ) ) ;
#14950=ORIENTED_EDGE ( 'NONE', *, *, #8563, .F. ) ;
#14952=CARTESIAN_POINT ( 'NONE',  ( 96.84719886470459471, 3.152801135295383084, 4.562500001365592084 ) ) ;
#14966=VECTOR ( 'NONE', #6715, 1000.000000000000000 ) ;
#14967=CARTESIAN_POINT ( 'NONE',  ( 95.54126587499996504, 1.387778780781445676E-14, 2.437500001365592084 ) ) ;
#14969=CARTESIAN_POINT ( 'NONE',  ( 101.8468681455906903, 4.458734125000016313, 2.125000001365591640 ) ) ;
#14985=CARTESIAN_POINT ( 'NONE',  ( 103.5355339059327093, -3.535533905932726206, 7.500000002731185944 ) ) ;
#15012=CARTESIAN_POINT ( 'NONE',  ( 96.46446609406721961, -3.535533905932727539, 3.250000002731184612 ) ) ;
#15016=ADVANCED_FACE ( 'NONE', ( #8623 ), #8764, .F. ) ;
#15024=CARTESIAN_POINT ( 'NONE',  ( 96.46446609406721961, 3.535533905932755072, 10.87500000000000000 ) ) ;
#15029=CARTESIAN_POINT ( 'NONE',  ( 96.84719886470459471, 3.152801135295383084, 10.31250000136559208 ) ) ;
#15031=ORIENTED_EDGE ( 'NONE', *, *, #20138, .T. ) ;
#15032=CARTESIAN_POINT ( 'NONE',  ( 99.99999999999995737, 1.387778780781445676E-14, 0.000000000000000000 ) ) ;
#15033=CARTESIAN_POINT ( 'NONE',  ( 95.54126587499995082, 1.846868145590750077, 11.37500000136559208 ) ) ;
#15047=CYLINDRICAL_SURFACE ( 'NONE', #21783, 5.000000000000004441 ) ;
#15055=EDGE_CURVE ( 'NONE', #27806, #6963, #20098, .T. ) ;
#15056=CARTESIAN_POINT ( 'NONE',  ( 104.9999999999999574, -2.071067811865462627, 5.437499999999999112 ) ) ;
#15060=ADVANCED_FACE ( 'NONE', ( #22741 ), #16162, .T. ) ;
#15072=CARTESIAN_POINT ( 'NONE',  ( 101.8468681455907046, -4.458734124999987891, 0.7500000013655925279 ) ) ;
#15087=CARTESIAN_POINT ( 'NONE',  ( 95.54126587499995082, -1.846868145590724986, 3.750000001365591640 ) ) ;
#15100=CARTESIAN_POINT ( 'NONE',  ( 95.54126587499995082, -1.846868145590724986, 2.500000001365592084 ) ) ;
#15102=CARTESIAN_POINT ( 'NONE',  ( 103.1528011352953342, 3.152801135295383084, 4.062500001365592084 ) ) ;
#15104=DIRECTION ( 'NONE',  ( 0.000000000000000000, 0.000000000000000000, 1.000000000000000000 ) ) ;
#15105=( BOUNDED_CURVE ( )  B_SPLINE_CURVE ( 2, ( #20602, #7763, #20743, #5636, #9753, #20462, #943, #3491, #18867 ),
 .UNSPECIFIED., .F., .F. ) 
 B_SPLINE_CURVE_WITH_KNOTS ( ( 3, 2, 2, 2, 3 ),
 ( 0.5357142857142856984, 0.5446428571428570953, 0.5535714285714286031, 0.5625000000000000000, 0.5714285714285713969 ),
 .UNSPECIFIED. ) 
 CURVE ( )  GEOMETRIC_REPRESENTATION_ITEM ( )  RATIONAL_B_SPLINE_CURVE ( ( 1.000000000000000000, 0.9238795325112867385, 1.000000000000000000, 0.9238795325112867385, 1.000000000000000000, 0.9238795325112867385, 1.000000000000000000, 0.9238795325112867385, 1.000000000000000000 ) ) 
 REPRESENTATION_ITEM ( '' )  );
#15120=CARTESIAN_POINT ( 'NONE',  ( 101.8468681455906903, 4.458734125000016313, 14.37500000136559386 ) ) ;
#15136=( NAMED_UNIT ( * ) SI_UNIT ( $, .STERADIAN. ) SOLID_ANGLE_UNIT ( ) );
#15138=CARTESIAN_POINT ( 'NONE',  ( 95.54126587499996504, -1.846868145590724986, 12.75000000136559208 ) ) ;
#15151=CARTESIAN_POINT ( 'NONE',  ( 103.5355339059327093, -3.535533905932726206, 3.500000002731184612 ) ) ;
#15158=CARTESIAN_POINT ( 'NONE',  ( 94.99999999999995737, 1.387778780781445676E-14, 10.12500000273118594 ) ) ;
#15168=CARTESIAN_POINT ( 'NONE',  ( 98.15313185440925281, 4.458734125000016313, 8.250000001365592084 ) ) ;
#15171=CARTESIAN_POINT ( 'NONE',  ( 99.99999999999995737, 4.458734125000016313, 11.18750000136559208 ) ) ;
#15178=CARTESIAN_POINT ( 'NONE',  ( 97.92893218813451028, 5.000000000000018652, 11.81250000000000000 ) ) ;
#15193=CARTESIAN_POINT ( 'NONE',  ( 102.0710678118654329, 5.000000000000018652, 5.687500000000000000 ) ) ;
#15207=EDGE_CURVE ( 'NONE', #6975, #15231, #23179, .T. ) ;
#15219=VERTEX_POINT ( 'NONE', #14299 ) ;
#15230=CARTESIAN_POINT ( 'NONE',  ( 104.4587341249999781, -1.846868145590721655, 2.125000001365591640 ) ) ;
#15231=VERTEX_POINT ( 'NONE', #3347 ) ;
#15242=CARTESIAN_POINT ( 'NONE',  ( 104.9999999999999716, 1.449011120738813565E-14, 9.500000000000000000 ) ) ;
#15243=CARTESIAN_POINT ( 'NONE',  ( 98.15313185440925281, -4.458734124999987891, 9.875000001365593860 ) ) ;
#15245=CARTESIAN_POINT ( 'NONE',  ( 103.1528011352953342, -3.152801135295355106, 13.81250000136559208 ) ) ;
#15246=ADVANCED_FACE ( 'NONE', ( #5634 ), #20878, .F. ) ;
#15250=AXIS2_PLACEMENT_3D ( 'NONE', #4585, #13245, #21977 ) ;
#15259=CARTESIAN_POINT ( 'NONE',  ( 94.99999999999995737, 1.387778780781445676E-14, 3.125000002731185944 ) ) ;
#15274=DIRECTION ( 'NONE',  ( -0.000000000000000000, -0.000000000000000000, -1.000000000000000000 ) ) ;
#15279=ORIENTED_EDGE ( 'NONE', *, *, #23532, .F. ) ;
#15282=CARTESIAN_POINT ( 'NONE',  ( 96.84719886470459471, 3.152801135295383084, 9.562500001365593860 ) ) ;
#15297=CARTESIAN_POINT ( 'NONE',  ( 94.99999999999995737, -2.071067811865466624, 3.187500002731184168 ) ) ;
#15302=PLANE ( 'NONE',  #2509 ) ;
#15314=CARTESIAN_POINT ( 'NONE',  ( 104.4587341249999781, -1.846868145590721655, 6.875000001365592972 ) ) ;
#15317=CARTESIAN_POINT ( 'NONE',  ( 96.84719886470459471, -3.152801135295355994, 10.56250000136559208 ) ) ;
#15327=CARTESIAN_POINT ( 'NONE',  ( 94.99999999999995737, 1.387778780781445676E-14, 11.12500000273118594 ) ) ;
#15339=CARTESIAN_POINT ( 'NONE',  ( 97.92893218813451028, 5.000000000000018652, 3.812500000000000000 ) ) ;
#15357=CARTESIAN_POINT ( 'NONE',  ( 95.54126587499996504, 1.387778780781445676E-14, 2.437500001365592084 ) ) ;
#15374=CARTESIAN_POINT ( 'NONE',  ( 99.99999999999995737, -4.458734124999988779, 2.937500001365592528 ) ) ;
#15383=ORIENTED_EDGE ( 'NONE', *, *, #9004, .T. ) ;
#15390=CARTESIAN_POINT ( 'NONE',  ( 98.15313185440925281, -4.458734124999987891, 10.87500000136559386 ) ) ;
#15392=CARTESIAN_POINT ( 'NONE',  ( 98.15313185440923860, -4.458734124999987891, 13.62500000136559208 ) ) ;
#15409=CARTESIAN_POINT ( 'NONE',  ( 103.1528011352953342, -3.152801135295355106, 14.06250000136559208 ) ) ;
#15426=CARTESIAN_POINT ( 'NONE',  ( 95.54126587499996504, -1.846868145590724986, 11.75000000136559208 ) ) ;
#15432=VECTOR ( 'NONE', #8493, 1000.000000000000000 ) ;
#15445=DIRECTION ( 'NONE',  ( -1.000000000000000000, 0.000000000000000000, 0.000000000000000000 ) ) ;
#15456=CARTESIAN_POINT ( 'NONE',  ( 94.99999999999994316, -2.071067811865456409, 10.06249999999999645 ) ) ;
#15458=CARTESIAN_POINT ( 'NONE',  ( 104.4587341249999639, 1.442382525525748735E-14, 9.937500001365592084 ) ) ;
#15460=CARTESIAN_POINT ( 'NONE',  ( 95.54126587499995082, -1.846868145590724986, 11.50000000136559208 ) ) ;
#15476=CARTESIAN_POINT ( 'NONE',  ( 94.99999999999995737, 1.387778780781445676E-14, 8.125000002731185944 ) ) ;
#15505=CARTESIAN_POINT ( 'NONE',  ( 103.1528011352953342, 3.152801135295383084, 4.062500001365592084 ) ) ;
#15511=ORIENTED_EDGE ( 'NONE', *, *, #23138, .T. ) ;
#15522=CARTESIAN_POINT ( 'NONE',  ( 97.92893218813451028, 5.000000000000018652, 12.81249999999999822 ) ) ;
#15535=CARTESIAN_POINT ( 'NONE',  ( 103.1528011352953342, -3.152801135295355106, 10.06250000136559386 ) ) ;
#15537=CARTESIAN_POINT ( 'NONE',  ( 95.54126587499996504, 1.387778780781445676E-14, 12.43750000136559208 ) ) ;
#15553=LINE ( 'NONE', #27985, #2114 ) ;
#15571=CARTESIAN_POINT ( 'NONE',  ( 103.1528011352953342, -3.152801135295355106, 13.06250000136559208 ) ) ;
#15584=ORIENTED_EDGE ( 'NONE', *, *, #5151, .F. ) ;
#15599=EDGE_CURVE ( 'NONE', #18726, #949, #11846, .T. ) ;
#15602=CARTESIAN_POINT ( 'NONE',  ( 95.54126587499995082, -1.846868145590724986, 6.500000001365592084 ) ) ;
#15605=CARTESIAN_POINT ( 'NONE',  ( 101.8468681455906903, 4.458734125000016313, 7.125000001365591196 ) ) ;
#15610=CARTESIAN_POINT ( 'NONE',  ( 96.46446609406721961, 3.535533905932755072, 7.000000002731185056 ) ) ;
#15623=CARTESIAN_POINT ( 'NONE',  ( 99.99999999999995737, -4.999999999999990230, 8.250000000000000000 ) ) ;
#15626=( BOUNDED_CURVE ( )  B_SPLINE_CURVE ( 2, ( #27565, #21008, #23006, #10430, #19139, #27844, #12142, #16989, #7885 ),
 .UNSPECIFIED., .F., .F. ) 
 B_SPLINE_CURVE_WITH_KNOTS ( ( 3, 2, 2, 2, 3 ),
 ( 0.5357142857142856984, 0.5446428571428570953, 0.5535714285714286031, 0.5625000000000000000, 0.5714285714285713969 ),
 .UNSPECIFIED. ) 
 CURVE ( )  GEOMETRIC_REPRESENTATION_ITEM ( )  RATIONAL_B_SPLINE_CURVE ( ( 1.000000000000000000, 0.9238795325112867385, 1.000000000000000000, 0.9238795325112867385, 1.000000000000000000, 0.9238795325112867385, 1.000000000000000000, 0.9238795325112867385, 1.000000000000000000 ) ) 
 REPRESENTATION_ITEM ( '' )  );
#15627=CARTESIAN_POINT ( 'NONE',  ( 103.5355339059327093, 3.535533905932755072, 9.750000002731184168 ) ) ;
#15638=CARTESIAN_POINT ( 'NONE',  ( 94.99999999999995737, 1.387778780781445676E-14, 6.125000002731185056 ) ) ;
#15650=CARTESIAN_POINT ( 'NONE',  ( 101.8468681455906903, -4.458734124999987891, 1.000000001365592528 ) ) ;
#15652=CARTESIAN_POINT ( 'NONE',  ( 99.99999999999995737, 4.458734125000016313, 2.187500001365592084 ) ) ;
#15669=CARTESIAN_POINT ( 'NONE',  ( 94.99999999999995737, -2.071067811865466624, 14.06249999999999645 ) ) ;
#15677=ORIENTED_EDGE ( 'NONE', *, *, #14871, .F. ) ;
#15682=CARTESIAN_POINT ( 'NONE',  ( 95.54126587499995082, 1.846868145590750077, 9.625000001365593860 ) ) ;
#15684=CARTESIAN_POINT ( 'NONE',  ( 98.15313185440925281, 4.458734125000016313, 1.250000001365592750 ) ) ;
#15698=CARTESIAN_POINT ( 'NONE',  ( 96.84719886470459471, -3.152801135295355994, 10.81250000136559208 ) ) ;
#15713=EDGE_LOOP ( 'NONE', ( #12665, #8805, #24437, #21073 ) ) ;
#15715=CARTESIAN_POINT ( 'NONE',  ( 101.8468681455907046, -4.458734124999987891, 11.00000000136559208 ) ) ;
#15718=CARTESIAN_POINT ( 'NONE',  ( 97.92893218813451028, -4.999999999999989342, 2.187499999999999112 ) ) ;
#15744=CARTESIAN_POINT ( 'NONE',  ( 99.99999999999995737, 4.458734125000016313, 4.187500001365592084 ) ) ;
#15748=CARTESIAN_POINT ( 'NONE',  ( 95.54126587499995082, -1.846868145590724986, 9.500000001365593860 ) ) ;
#15752=CARTESIAN_POINT ( 'NONE',  ( 94.99999999999995737, 1.387778780781445676E-14, 7.125000002731185056 ) ) ;
#15765=CARTESIAN_POINT ( 'NONE',  ( 104.9999999999999574, -2.071067811865462627, 11.56250000273118772 ) ) ;
#15768=ADVANCED_FACE ( 'NONE', ( #14241 ), #27514, .F. ) ;
#15772=CARTESIAN_POINT ( 'NONE',  ( 103.5355339059327093, -3.535533905932726206, 1.374999999999999556 ) ) ;
#15776=DIRECTION ( 'NONE',  ( 0.000000000000000000, 0.000000000000000000, 1.000000000000000000 ) ) ;
#15784=( BOUNDED_CURVE ( )  B_SPLINE_CURVE ( 2, ( #22464, #11599, #20322, #20609, #2929, #1093, #9760, #18470, #27178 ),
 .UNSPECIFIED., .F., .T. ) 
 B_SPLINE_CURVE_WITH_KNOTS ( ( 3, 2, 2, 2, 3 ),
 ( 0.07142857142857149400, 0.08035714285714290472, 0.08928571428571430157, 0.09821428571428571230, 0.1071428571428571092 ),
 .UNSPECIFIED. ) 
 CURVE ( )  GEOMETRIC_REPRESENTATION_ITEM ( )  RATIONAL_B_SPLINE_CURVE ( ( 0.9999999999999994449, 0.9238795325112872936, 1.000000000000000000, 0.9238795325112867385, 1.000000000000000000, 0.9238795325112867385, 1.000000000000000000, 0.9238795325112869605, 0.9999999999999997780 ) ) 
 REPRESENTATION_ITEM ( '' )  );
#15791=CARTESIAN_POINT ( 'NONE',  ( 96.46446609406721961, -3.535533905932727539, 4.250000002731185056 ) ) ;
#15811=CARTESIAN_POINT ( 'NONE',  ( 97.92893218813451028, 5.000000000000018652, 11.81249999999999822 ) ) ;
#15823=CARTESIAN_POINT ( 'NONE',  ( 95.54126587499995082, -1.846868145590724986, 12.75000000136559386 ) ) ;
#15825=CARTESIAN_POINT ( 'NONE',  ( 98.15313185440923860, -4.458734124999987891, 9.625000001365593860 ) ) ;
#15833=CARTESIAN_POINT ( 'NONE',  ( 94.99999999999995737, -2.071067811865466624, 1.062499999999999112 ) ) ;
#15838=CARTESIAN_POINT ( 'NONE',  ( 104.4587341249999639, 1.442382525525748735E-14, 12.18750000136559208 ) ) ;
#15839=ORIENTED_EDGE ( 'NONE', *, *, #19768, .T. ) ;
#15845=CARTESIAN_POINT ( 'NONE',  ( 94.99999999999995737, 1.387778780781445676E-14, 11.12500000273118594 ) ) ;
#15856=CARTESIAN_POINT ( 'NONE',  ( 103.1528011352953342, 3.152801135295383084, 8.312500001365592084 ) ) ;
#15859=CARTESIAN_POINT ( 'NONE',  ( 103.5355339059327093, -3.535533905932726206, 14.37499999999999822 ) ) ;
#15882=CARTESIAN_POINT ( 'NONE',  ( 96.84719886470459471, 3.152801135295383084, 4.312500001365592084 ) ) ;
#15885=CARTESIAN_POINT ( 'NONE',  ( 98.15313185440925281, 4.458734125000016313, 8.250000001365592084 ) ) ;
#15900=CARTESIAN_POINT ( 'NONE',  ( 94.99999999999995737, -2.071067811865466624, 9.187500002731184168 ) ) ;
#15905=CARTESIAN_POINT ( 'NONE',  ( 104.9999999999999716, 1.449011120738813565E-14, 2.499999999999998668 ) ) ;
#15909=CARTESIAN_POINT ( 'NONE',  ( 97.92893218813451028, 5.000000000000018652, 5.937500002731185056 ) ) ;
#15946=CARTESIAN_POINT ( 'NONE',  ( 96.46446609406721961, -3.535533905932727539, 12.12500000000000000 ) ) ;
#15954=CARTESIAN_POINT ( 'NONE',  ( 94.99999999999995737, -2.071067811865466624, 3.062499999999999112 ) ) ;
#15961=CARTESIAN_POINT ( 'NONE',  ( 101.8468681455906903, -4.458734124999987891, 8.000000001365592084 ) ) ;
#15964=CARTESIAN_POINT ( 'NONE',  ( 98.15313185440923860, -4.458734124999987891, 8.625000001365592084 ) ) ;
#15967=CARTESIAN_POINT ( 'NONE',  ( 104.9999999999999716, 1.449011120738813565E-14, 34.79898987322334136 ) ) ;
#15976=ORIENTED_EDGE ( 'NONE', *, *, #24123, .T. ) ;
#15978=CARTESIAN_POINT ( 'NONE',  ( 95.54126587499995082, 1.846868145590750077, 11.62500000136559031 ) ) ;
#15993=CARTESIAN_POINT ( 'NONE',  ( 104.4587341249999781, -1.846868145590721655, 6.125000001365592084 ) ) ;
#15997=ORIENTED_EDGE ( 'NONE', *, *, #19057, .T. ) ;
#15999=( BOUNDED_CURVE ( )  B_SPLINE_CURVE ( 2, ( #16909, #27898, #27354, #14758, #19195, #1552, #5549, #12200, #1270 ),
 .UNSPECIFIED., .F., .F. ) 
 B_SPLINE_CURVE_WITH_KNOTS ( ( 3, 2, 2, 2, 3 ),
 ( 0.7857142857142856984, 0.7946428571428570953, 0.8035714285714286031, 0.8125000000000000000, 0.8214285714285713969 ),
 .UNSPECIFIED. ) 
 CURVE ( )  GEOMETRIC_REPRESENTATION_ITEM ( )  RATIONAL_B_SPLINE_CURVE ( ( 1.000000000000000000, 0.9238795325112867385, 1.000000000000000000, 0.9238795325112867385, 1.000000000000000000, 0.9238795325112867385, 1.000000000000000000, 0.9238795325112867385, 1.000000000000000000 ) ) 
 REPRESENTATION_ITEM ( '' )  );
#16005=EDGE_LOOP ( 'NONE', ( #27633, #28133, #7478, #6650 ) ) ;
#16023=CARTESIAN_POINT ( 'NONE',  ( 104.4587341249999639, 1.442382525525748735E-14, 2.937500001365592528 ) ) ;
#16026=CARTESIAN_POINT ( 'NONE',  ( 103.1528011352953342, 3.152801135295383084, 9.062500001365592084 ) ) ;
#16037=FACE_BOUND ( 'NONE', #13271, .T. ) ;
#16044=CARTESIAN_POINT ( 'NONE',  ( 102.0710678118654329, -4.999999999999989342, 8.437500002731185944 ) ) ;
#16059=AXIS2_PLACEMENT_3D ( 'NONE', #5082, #13744, #22468 ) ;
#16062=CARTESIAN_POINT ( 'NONE',  ( 99.99999999999995737, 1.387778780781445676E-14, 34.79898987322334136 ) ) ;
#16091=CARTESIAN_POINT ( 'NONE',  ( 96.46446609406721961, 3.535533905932755072, 13.87499999999999822 ) ) ;
#16097=CARTESIAN_POINT ( 'NONE',  ( 104.9999999999999574, -2.071067811865462627, 13.56250000273118772 ) ) ;
#16107=CARTESIAN_POINT ( 'NONE',  ( 95.54126587499995082, -1.846868145590724986, 8.750000001365592084 ) ) ;
#16109=CARTESIAN_POINT ( 'NONE',  ( 96.84719886470459471, -3.152801135295355994, 11.56250000136559208 ) ) ;
#16123=CARTESIAN_POINT ( 'NONE',  ( 104.4587341249999781, 1.846868145590750299, 10.25000000136559386 ) ) ;
#16125=ORIENTED_EDGE ( 'NONE', *, *, #21370, .F. ) ;
#16142=CARTESIAN_POINT ( 'NONE',  ( 95.54126587499996504, 1.846868145590750077, 7.625000001365592084 ) ) ;
#16145=LINE ( 'NONE', #20154, #5797 ) ;
#16160=VERTEX_POINT ( 'NONE', #18063 ) ;
#16162=CYLINDRICAL_SURFACE ( 'NONE', #10847, 7.000000000000006217 ) ;
#16167=DIRECTION ( 'NONE',  ( -0.000000000000000000, -0.000000000000000000, -1.000000000000000000 ) ) ;
#16172=CARTESIAN_POINT ( 'NONE',  ( 103.1528011352953342, -3.152801135295355106, 3.812500001365591640 ) ) ;
#16173=ORIENTED_EDGE ( 'NONE', *, *, #7755, .T. ) ;
#16175=CARTESIAN_POINT ( 'NONE',  ( 98.15313185440925281, -4.458734124999987891, 9.625000001365593860 ) ) ;
#16192=CARTESIAN_POINT ( 'NONE',  ( 103.5355339059327093, -3.535533905932726206, 6.500000002731185944 ) ) ;
#16196=CARTESIAN_POINT ( 'NONE',  ( 104.9999999999999716, 1.449011120738813565E-14, 14.49999999999999822 ) ) ;
#16209=CARTESIAN_POINT ( 'NONE',  ( 99.99999999999995737, 1.387778780781445676E-14, 34.79898987322334136 ) ) ;
#16242=CARTESIAN_POINT ( 'NONE',  ( 94.99999999999995737, -2.071067811865466624, 8.062500000000000000 ) ) ;
#16243=ORIENTED_EDGE ( 'NONE', *, *, #6900, .F. ) ;
#16247=CARTESIAN_POINT ( 'NONE',  ( 102.0710678118654329, -4.999999999999989342, 12.43750000273118950 ) ) ;
#16253=CARTESIAN_POINT ( 'NONE',  ( 95.54126587499996504, 1.387778780781445676E-14, 8.687500001365592084 ) ) ;
#16255=CARTESIAN_POINT ( 'NONE',  ( 104.4587341249999639, 1.442382525525748735E-14, 9.937500001365592084 ) ) ;
#16271=CARTESIAN_POINT ( 'NONE',  ( 95.54126587499995082, 1.846868145590750077, 10.62500000136559208 ) ) ;
#16286=CARTESIAN_POINT ( 'NONE',  ( 104.4587341249999781, -1.846868145590721655, 8.125000001365592084 ) ) ;
#16303=CARTESIAN_POINT ( 'NONE',  ( 103.5355339059327093, -3.535533905932726206, 0.5000000027311855000 ) ) ;
#16310=DIRECTION ( 'NONE',  ( -0.000000000000000000, -0.000000000000000000, -1.000000000000000000 ) ) ;
#16311=CARTESIAN_POINT ( 'NONE',  ( 99.99999999999995737, 5.000000000000018652, 8.875000002731184168 ) ) ;
#16312=CARTESIAN_POINT ( 'NONE',  ( 103.1528011352953342, -3.152801135295355106, 1.062500001365592528 ) ) ;
#16313=CARTESIAN_POINT ( 'NONE',  ( 99.99999999999995737, 1.387778780781445676E-14, 34.79898987322334136 ) ) ;
#16316=CARTESIAN_POINT ( 'NONE',  ( 106.9999999999999716, 1.473504056721760595E-14, 0.000000000000000000 ) ) ;
#16320=CARTESIAN_POINT ( 'NONE',  ( 104.4587341249999781, 1.846868145590750299, 13.25000000136559208 ) ) ;
#16338=CARTESIAN_POINT ( 'NONE',  ( 102.0710678118654329, 5.000000000000018652, 4.812500002731185056 ) ) ;
#16381=VECTOR ( 'NONE', #23144, 1000.000000000000000 ) ;
#16382=CARTESIAN_POINT ( 'NONE',  ( 97.92893218813451028, 5.000000000000018652, 7.812499999999999112 ) ) ;
#16386=( BOUNDED_CURVE ( )  B_SPLINE_CURVE ( 2, ( #20314, #7040, #24589, #5072, #20033, #11594, #13734, #9056, #26738 ),
 .UNSPECIFIED., .F., .F. ) 
 B_SPLINE_CURVE_WITH_KNOTS ( ( 3, 2, 2, 2, 3 ),
 ( 0.8214285714285713969, 0.8303571428571429047, 0.8392857142857143016, 0.8482142857142856984, 0.8571428571428570953 ),
 .UNSPECIFIED. ) 
 CURVE ( )  GEOMETRIC_REPRESENTATION_ITEM ( )  RATIONAL_B_SPLINE_CURVE ( ( 1.000000000000000000, 0.9238795325112867385, 1.000000000000000000, 0.9238795325112867385, 1.000000000000000000, 0.9238795325112867385, 1.000000000000000000, 0.9238795325112867385, 1.000000000000000000 ) ) 
 REPRESENTATION_ITEM ( '' )  );
#16388=CARTESIAN_POINT ( 'NONE',  ( 99.99999999999995737, 5.000000000000018652, 11.87500000273118594 ) ) ;
#16398=CARTESIAN_POINT ( 'NONE',  ( 104.4587341249999639, 1.442382525525748735E-14, 7.187500001365592972 ) ) ;
#16401=CARTESIAN_POINT ( 'NONE',  ( 101.8468681455907046, -4.458734124999987891, 10.75000000136559208 ) ) ;
#16404=CARTESIAN_POINT ( 'NONE',  ( 94.99999999999995737, 1.387778780781445676E-14, 4.000000000000000000 ) ) ;
#16413=CARTESIAN_POINT ( 'NONE',  ( 96.84719886470459471, -3.152801135295355994, 8.812500001365592084 ) ) ;
#16426=CARTESIAN_POINT ( 'NONE',  ( 101.8468681455907046, 4.458734125000016313, 8.375000001365592084 ) ) ;
#16436=CARTESIAN_POINT ( 'NONE',  ( 99.99999999999995737, 1.387778780781445676E-14, 34.79898987322334136 ) ) ;
#16451=DIRECTION ( 'NONE',  ( -0.000000000000000000, -0.000000000000000000, -1.000000000000000000 ) ) ;
#16456=CARTESIAN_POINT ( 'NONE',  ( 104.4587341249999639, 1.442382525525748735E-14, 0.9375000013655925279 ) ) ;
#16459=ADVANCED_FACE ( 'NONE', ( #27568 ), #9746, .F. ) ;
#16474=CARTESIAN_POINT ( 'NONE',  ( 96.46446609406721961, -3.535533905932727539, 5.250000002731184168 ) ) ;
#16484=ORIENTED_EDGE ( 'NONE', *, *, #5894, .T. ) ;
#16494=CARTESIAN_POINT ( 'NONE',  ( 101.8468681455906903, 4.458734125000016313, 13.12500000136559208 ) ) ;
#16509=VERTEX_POINT ( 'NONE', #1356 ) ;
#16524=CARTESIAN_POINT ( 'NONE',  ( 97.92893218813451028, -4.999999999999989342, 8.187500000000000000 ) ) ;
#16529=CARTESIAN_POINT ( 'NONE',  ( 104.9999999999999574, 2.071067811865491937, 13.68750000273118772 ) ) ;
#16533=CARTESIAN_POINT ( 'NONE',  ( 95.54126587499996504, 1.387778780781445676E-14, 14.43750000136559208 ) ) ;
#16540=CARTESIAN_POINT ( 'NONE',  ( 95.54126587499995082, -1.846868145590724986, 5.750000001365591196 ) ) ;
#16542=CARTESIAN_POINT ( 'NONE',  ( 96.84719886470459471, -3.152801135295355994, 6.562500001365592084 ) ) ;
#16555=CARTESIAN_POINT ( 'NONE',  ( 99.99999999999995737, 4.458734125000016313, 5.437500001365592972 ) ) ;
#16559=DIRECTION ( 'NONE',  ( -0.000000000000000000, -0.000000000000000000, -1.000000000000000000 ) ) ;
#16568=CARTESIAN_POINT ( 'NONE',  ( 103.1528011352953342, -3.152801135295355106, 2.062500001365591640 ) ) ;
#16576=LINE ( 'NONE', #10141, #16381 ) ;
#16580=CARTESIAN_POINT ( 'NONE',  ( 95.54126587499996504, 1.387778780781445676E-14, 0.5625000013655921949 ) ) ;
#16596=ORIENTED_EDGE ( 'NONE', *, *, #9191, .T. ) ;
#16599=CARTESIAN_POINT ( 'NONE',  ( 103.1528011352953342, 3.152801135295383084, 1.062500001365592528 ) ) ;
#16600=CARTESIAN_POINT ( 'NONE',  ( 99.99999999999995737, 4.458734125000016313, 14.43750000136559208 ) ) ;
#16616=CARTESIAN_POINT ( 'NONE',  ( 104.9999999999999574, -2.071067811865462627, 5.562500002731184168 ) ) ;
#16634=CARTESIAN_POINT ( 'NONE',  ( 103.1528011352953342, -3.152801135295355106, 13.81250000136559208 ) ) ;
#16664=CARTESIAN_POINT ( 'NONE',  ( 99.99999999999995737, 5.000000000000018652, 10.75000000000000000 ) ) ;
#16676=CARTESIAN_POINT ( 'NONE',  ( 95.54126587499996504, 1.387778780781445676E-14, 4.687500001365592084 ) ) ;
#16678=CARTESIAN_POINT ( 'NONE',  ( 95.54126587499996504, 1.846868145590750077, 5.375000001365592972 ) ) ;
#16688=ORIENTED_EDGE ( 'NONE', *, *, #23758, .F. ) ;
#16693=CARTESIAN_POINT ( 'NONE',  ( 98.15313185440925281, 4.458734125000016313, 8.500000001365592084 ) ) ;
#16708=CARTESIAN_POINT ( 'NONE',  ( 95.54126587499995082, 1.846868145590750077, 2.375000001365592084 ) ) ;
#16710=CARTESIAN_POINT ( 'NONE',  ( 103.1528011352953342, -3.152801135295355106, 5.062500001365592972 ) ) ;
#16734=CARTESIAN_POINT ( 'NONE',  ( 104.9999999999999716, 1.449011120738813565E-14, 3.625000002731184612 ) ) ;
#16739=CARTESIAN_POINT ( 'NONE',  ( 104.4587341249999781, 1.846868145590750521, 13.25000000136559564 ) ) ;
#16746=DIRECTION ( 'NONE',  ( -0.000000000000000000, -0.000000000000000000, -1.000000000000000000 ) ) ;
#16748=ORIENTED_EDGE ( 'NONE', *, *, #11387, .F. ) ;
#16751=CARTESIAN_POINT ( 'NONE',  ( 104.9999999999999574, -2.071067811865462627, 7.562500002731187720 ) ) ;
#16770=CARTESIAN_POINT ( 'NONE',  ( 104.4587341249999781, 1.846868145590750299, 12.00000000136559208 ) ) ;
#16775=CARTESIAN_POINT ( 'NONE',  ( 102.0710678118654329, 5.000000000000018652, 8.687499999999998224 ) ) ;
#16780=ADVANCED_FACE ( 'NONE', ( #8585 ), #10846, .F. ) ;
#16797=CARTESIAN_POINT ( 'NONE',  ( 99.99999999999995737, -4.999999999999990230, 10.24999999999999822 ) ) ;
#16812=CARTESIAN_POINT ( 'NONE',  ( 99.99999999999995737, 1.387778780781445676E-14, 34.79898987322334136 ) ) ;
#16813=CARTESIAN_POINT ( 'NONE',  ( 104.4587341249999639, 1.442382525525748735E-14, 1.187500001365592750 ) ) ;
#16816=CARTESIAN_POINT ( 'NONE',  ( 99.99999999999995737, -4.458734124999988779, 6.687500001365592084 ) ) ;
#16819=CIRCLE ( 'NONE', #17712, 7.000000000000006217 ) ;
#16831=CARTESIAN_POINT ( 'NONE',  ( 96.84719886470459471, -3.152801135295355994, 5.812500001365591196 ) ) ;
#16845=CARTESIAN_POINT ( 'NONE',  ( 96.84719886470459471, -3.152801135295355994, 2.562500001365592084 ) ) ;
#16847=CARTESIAN_POINT ( 'NONE',  ( 101.8468681455907046, 4.458734125000016313, 4.375000001365592084 ) ) ;
#16875=( LENGTH_UNIT ( ) NAMED_UNIT ( * ) SI_UNIT ( .MILLI., .METRE. ) );
#16886=CARTESIAN_POINT ( 'NONE',  ( 99.99999999999995737, 5.000000000000018652, 2.875000002731185944 ) ) ;
#16902=CARTESIAN_POINT ( 'NONE',  ( 104.4587341249999781, 1.846868145590750299, 11.00000000136559208 ) ) ;
#16903=CARTESIAN_POINT ( 'NONE',  ( 104.9999999999999574, -2.071067811865468844, 13.56250000273118417 ) ) ;
#16909=CARTESIAN_POINT ( 'NONE',  ( 94.99999999999995737, 1.387778780781445676E-14, 3.125000002731185944 ) ) ;
#16925=EDGE_CURVE ( 'NONE', #27294, #22247, #20913, .T. ) ;
#16929=CARTESIAN_POINT ( 'NONE',  ( 104.9999999999999574, 2.071067811865491937, 5.562500000000000000 ) ) ;
#16934=CARTESIAN_POINT ( 'NONE',  ( 96.46446609406721961, -3.535533905932727539, 11.12500000000000000 ) ) ;
#16939=CARTESIAN_POINT ( 'NONE',  ( 102.0710678118654329, -4.999999999999989342, 8.437500002731185944 ) ) ;
#16940=CARTESIAN_POINT ( 'NONE',  ( 96.84719886470459471, -3.152801135295355994, 2.812500001365592528 ) ) ;
#16942=CARTESIAN_POINT ( 'NONE',  ( 98.15313185440923860, -4.458734124999987891, 7.625000001365592084 ) ) ;
#16959=CARTESIAN_POINT ( 'NONE',  ( 103.1528011352953342, -3.152801135295355106, 6.062500001365592084 ) ) ;
#16974=EDGE_CURVE ( 'NONE', #25528, #11744, #21996, .T. ) ;
#16976=CARTESIAN_POINT ( 'NONE',  ( 99.99999999999995737, -4.458734124999988779, 4.687500001365592084 ) ) ;
#16977=CARTESIAN_POINT ( 'NONE',  ( 103.5355339059327093, 3.535533905932755072, 3.750000002731185056 ) ) ;
#16979=CARTESIAN_POINT ( 'NONE',  ( 96.84719886470459471, -3.152801135295355994, 2.812500001365592528 ) ) ;
#16989=CARTESIAN_POINT ( 'NONE',  ( 94.99999999999995737, -2.071067811865466624, 6.187500002731185056 ) ) ;
#17003=ORIENTED_EDGE ( 'NONE', *, *, #23995, .F. ) ;
#17006=CARTESIAN_POINT ( 'NONE',  ( 99.99999999999995737, -4.458734124999988779, 13.93750000136559208 ) ) ;
#17019=CARTESIAN_POINT ( 'NONE',  ( 97.92893218813451028, 5.000000000000018652, 0.9375000027311859441 ) ) ;
#17028=CARTESIAN_POINT ( 'NONE',  ( 94.99999999999995737, 1.387778780781445676E-14, 5.999999999999998224 ) ) ;
#17037=CARTESIAN_POINT ( 'NONE',  ( 103.1528011352953342, -3.152801135295355106, 10.81250000136559208 ) ) ;
#17041=CARTESIAN_POINT ( 'NONE',  ( 96.84719886470459471, 3.152801135295383084, 11.31250000136559208 ) ) ;
#17053=VERTEX_POINT ( 'NONE', #15845 ) ;
#17054=DIRECTION ( 'NONE',  ( -0.000000000000000000, -0.000000000000000000, -1.000000000000000000 ) ) ;
#17062=EDGE_LOOP ( 'NONE', ( #12672, #5839, #4989, #16243 ) ) ;
#17063=CARTESIAN_POINT ( 'NONE',  ( 99.99999999999995737, -4.999999999999990230, 4.249999999999998224 ) ) ;
#17076=CARTESIAN_POINT ( 'NONE',  ( 95.54126587499995082, -1.846868145590724986, 2.750000001365592084 ) ) ;
#17081=CARTESIAN_POINT ( 'NONE',  ( 95.54126587499996504, 1.846868145590750077, 6.375000001365592084 ) ) ;
#17087=ORIENTED_EDGE ( 'NONE', *, *, #22101, .F. ) ;
#17096=CARTESIAN_POINT ( 'NONE',  ( 96.84719886470459471, 3.152801135295383084, 1.562500001365592972 ) ) ;
#17111=CARTESIAN_POINT ( 'NONE',  ( 98.15313185440925281, 4.458734125000016313, 1.250000001365592750 ) ) ;
#17113=CARTESIAN_POINT ( 'NONE',  ( 101.8468681455906903, -4.458734124999987891, 3.750000001365591640 ) ) ;
#17114=CARTESIAN_POINT ( 'NONE',  ( 104.9999999999999716, 2.071067811865491937, 3.687500002731185056 ) ) ;
#17115=CARTESIAN_POINT ( 'NONE',  ( 95.54126587499996504, -1.846868145590724986, 0.7500000013655925279 ) ) ;
#17135=CARTESIAN_POINT ( 'NONE',  ( 99.99999999999995737, 4.458734125000016313, 14.43750000136559208 ) ) ;
#17138=CARTESIAN_POINT ( 'NONE',  ( 104.9999999999999716, 1.449011120738813565E-14, 5.500000000000000000 ) ) ;
#17166=CARTESIAN_POINT ( 'NONE',  ( 94.99999999999995737, 2.071067811865491048, 2.062500002731185500 ) ) ;
#17177=CARTESIAN_POINT ( 'NONE',  ( 94.99999999999995737, 1.387778780781445676E-14, 11.00000000000000000 ) ) ;
#17180=CARTESIAN_POINT ( 'NONE',  ( 95.54126587499995082, 1.846868145590750077, 7.375000001365592084 ) ) ;
#17184=CARTESIAN_POINT ( 'NONE',  ( 95.54126587499995082, -1.846868145590724986, 12.50000000136559208 ) ) ;
#17201=( BOUNDED_CURVE ( )  B_SPLINE_CURVE ( 2, ( #3537, #16903, #21337, #25600, #10621, #6086, #14752, #1405, #10064 ),
 .UNSPECIFIED., .F., .F. ) 
 B_SPLINE_CURVE_WITH_KNOTS ( ( 3, 2, 2, 2, 3 ),
 ( 0.03571428571428574700, 0.04464285714285718548, 0.05357142857142861703, 0.06250000000000005551, 0.07142857142857149400 ),
 .UNSPECIFIED. ) 
 CURVE ( )  GEOMETRIC_REPRESENTATION_ITEM ( )  RATIONAL_B_SPLINE_CURVE ( ( 0.9999999999999996669, 0.9238795325112870716, 1.000000000000000000, 0.9238795325112867385, 1.000000000000000000, 0.9238795325112867385, 1.000000000000000000, 0.9238795325112861834, 1.000000000000000666 ) ) 
 REPRESENTATION_ITEM ( '' )  );
#17207=CARTESIAN_POINT ( 'NONE',  ( 104.9999999999999716, 1.449011120738813565E-14, 5.500000000000000000 ) ) ;
#17208=CARTESIAN_POINT ( 'NONE',  ( 102.0710678118654329, 5.000000000000018652, 1.687499999999999778 ) ) ;
#17221=CARTESIAN_POINT ( 'NONE',  ( 95.54126587499996504, 1.387778780781445676E-14, 1.687500001365591418 ) ) ;
#17223=CARTESIAN_POINT ( 'NONE',  ( 104.4587341249999639, 1.442382525525748735E-14, 0.9375000013655925279 ) ) ;
#17230=AXIS2_PLACEMENT_3D ( 'NONE', #16313, #3769, #14160 ) ;
#17235=ORIENTED_EDGE ( 'NONE', *, *, #13476, .F. ) ;
#17240=CARTESIAN_POINT ( 'NONE',  ( 99.99999999999995737, -4.458734124999988779, 0.9375000013655925279 ) ) ;
#17258=CARTESIAN_POINT ( 'NONE',  ( 101.8468681455906903, -4.458734124999987891, 1.750000001365591862 ) ) ;
#17260=CARTESIAN_POINT ( 'NONE',  ( 95.54126587499996504, 1.387778780781445676E-14, 3.437500001365592972 ) ) ;
#17267=ORIENTED_EDGE ( 'NONE', *, *, #28137, .T. ) ;
#17272=ORIENTED_EDGE ( 'NONE', *, *, #27289, .T. ) ;
#17275=CARTESIAN_POINT ( 'NONE',  ( 99.99999999999995737, 1.387778780781445676E-14, 34.79898987322334136 ) ) ;
#17281=VECTOR ( 'NONE', #1624, 1000.000000000000000 ) ;
#17289=ORIENTED_EDGE ( 'NONE', *, *, #20138, .F. ) ;
#17291=CARTESIAN_POINT ( 'NONE',  ( 103.1528011352953342, -3.152801135295355106, 11.06250000136559208 ) ) ;
#17297=CARTESIAN_POINT ( 'NONE',  ( 94.99999999999995737, 1.387778780781445676E-14, 12.00000000000000000 ) ) ;
#17305=CARTESIAN_POINT ( 'NONE',  ( 103.5355339059327093, -3.535533905932726206, 2.500000002731185500 ) ) ;
#17310=DIRECTION ( 'NONE',  ( 0.000000000000000000, -1.000000000000000000, 0.000000000000000000 ) ) ;
#17327=CARTESIAN_POINT ( 'NONE',  ( 98.15313185440925281, -4.458734124999987891, 9.625000001365593860 ) ) ;
#17329=CARTESIAN_POINT ( 'NONE',  ( 95.54126587499995082, 1.846868145590750077, 12.37500000136559208 ) ) ;
#17348=ADVANCED_FACE ( 'NONE', ( #9964 ), #18253, .T. ) ;
#17351=CARTESIAN_POINT ( 'NONE',  ( 94.99999999999995737, -2.071067811865466624, 4.062499999999998224 ) ) ;
#17356=EDGE_CURVE ( 'NONE', #13106, #5755, #24669, .T. ) ;
#17362=CARTESIAN_POINT ( 'NONE',  ( 94.99999999999995737, 1.387778780781445676E-14, 12.12500000273118594 ) ) ;
#17369=CARTESIAN_POINT ( 'NONE',  ( 101.8468681455907046, 4.458734125000016313, 2.125000001365591640 ) ) ;
#17372=CARTESIAN_POINT ( 'NONE',  ( 103.5355339059327093, 3.535533905932755072, 4.624999999999999112 ) ) ;
#17384=CARTESIAN_POINT ( 'NONE',  ( 104.4587341249999781, -1.846868145590721655, 4.125000001365592084 ) ) ;
#17393=EDGE_CURVE ( 'NONE', #26730, #15219, #11493, .T. ) ;
#17399=CARTESIAN_POINT ( 'NONE',  ( 104.4587341249999781, 1.846868145590750299, 9.250000001365593860 ) ) ;
#17401=CARTESIAN_POINT ( 'NONE',  ( 104.4587341249999781, -1.846868145590721655, 1.875000001365591862 ) ) ;
#17418=DIRECTION ( 'NONE',  ( -0.8660254037844404840, -0.000000000000000000, -0.4999999999999967804 ) ) ;
#17431=EDGE_LOOP ( 'NONE', ( #1066, #27370, #12449, #4069 ) ) ;
#17434=CARTESIAN_POINT ( 'NONE',  ( 103.1528011352953342, -3.152801135295355106, 12.06250000136559208 ) ) ;
#17447=CARTESIAN_POINT ( 'NONE',  ( 102.0710678118654329, 5.000000000000018652, 2.812500002731185944 ) ) ;
#17451=DIRECTION ( 'NONE',  ( -0.000000000000000000, -0.000000000000000000, -1.000000000000000000 ) ) ;
#17453=CARTESIAN_POINT ( 'NONE',  ( 104.9999999999999574, 2.071067811865501263, 9.687500002731182391 ) ) ;
#17461=CARTESIAN_POINT ( 'NONE',  ( 101.8468681455906903, 4.458734125000016313, 7.125000001365591196 ) ) ;
#17464=CARTESIAN_POINT ( 'NONE',  ( 104.4587341249999781, -1.846868145590721655, 12.87500000136559208 ) ) ;
#17479=CARTESIAN_POINT ( 'NONE',  ( 104.9999999999999716, 1.449011120738813565E-14, 8.499999999999998224 ) ) ;
#17488=CARTESIAN_POINT ( 'NONE',  ( 96.46446609406721961, -3.535533905932727539, 4.124999999999998224 ) ) ;
#17507=CARTESIAN_POINT ( 'NONE',  ( 98.15313185440923860, -4.458734124999987891, 2.625000001365592084 ) ) ;
#17524=ORIENTED_EDGE ( 'NONE', *, *, #15055, .F. ) ;
#17526=CARTESIAN_POINT ( 'NONE',  ( 103.1528011352953342, -3.152801135295355106, 4.062500001365592084 ) ) ;
#17530=UNCERTAINTY_MEASURE_WITH_UNIT (LENGTH_MEASURE( 1.000000000000000082E-05 ), #13440, 'distance_accuracy_value', 'NONE');
#17539=CARTESIAN_POINT ( 'NONE',  ( 96.84719886470459471, 3.152801135295383084, 10.56250000136559208 ) ) ;
#17541=CARTESIAN_POINT ( 'NONE',  ( 104.4587341249999781, -1.846868145590721655, 12.87500000136559208 ) ) ;
#17558=DIRECTION ( 'NONE',  ( -1.000000000000000000, 0.000000000000000000, 0.000000000000000000 ) ) ;
#17574=CARTESIAN_POINT ( 'NONE',  ( 95.54126587499996504, 1.846868145590750077, 9.625000001365593860 ) ) ;
#17582=CARTESIAN_POINT ( 'NONE',  ( 96.46446609406721961, -3.535533905932727539, 12.12500000000000000 ) ) ;
#17600=CARTESIAN_POINT ( 'NONE',  ( 99.99999999999995737, 1.387778780781445676E-14, 15.00000000000000000 ) ) ;
#17604=CARTESIAN_POINT ( 'NONE',  ( 103.1528011352953342, 3.152801135295383084, 9.062500001365592084 ) ) ;
#17606=CARTESIAN_POINT ( 'NONE',  ( 98.15313185440925281, -4.458734124999987891, 12.62500000136559208 ) ) ;
#17629=CARTESIAN_POINT ( 'NONE',  ( 102.0710678118654329, -4.999999999999989342, 1.312499999999999556 ) ) ;
#17649=CARTESIAN_POINT ( 'NONE',  ( 95.54126587499996504, -1.846868145590724986, 2.500000001365592084 ) ) ;
#17667=CARTESIAN_POINT ( 'NONE',  ( 96.84719886470459471, -3.152801135295355994, 4.812500001365592084 ) ) ;
#17680=EDGE_CURVE ( 'NONE', #5755, #7831, #3704, .T. ) ;
#17685=CIRCLE ( 'NONE', #20889, 7.000000000000006217 ) ;
#17687=CARTESIAN_POINT ( 'NONE',  ( 96.84719886470459471, -3.152801135295355994, 11.81250000136559208 ) ) ;
#17689=CARTESIAN_POINT ( 'NONE',  ( 103.1528011352953342, 3.152801135295383084, 14.06250000136559208 ) ) ;
#17691=AXIS2_PLACEMENT_3D ( 'NONE', #16062, #2690, #24770 ) ;
#17706=CARTESIAN_POINT ( 'NONE',  ( 101.8468681455906903, -4.458734124999987891, 13.00000000136559386 ) ) ;
#17712=AXIS2_PLACEMENT_3D ( 'NONE', #26103, #15104, #4447 ) ;
#17724=CARTESIAN_POINT ( 'NONE',  ( 103.1528011352953342, 3.152801135295383084, 9.312500001365593860 ) ) ;
#17739=CIRCLE ( 'NONE', #4093, 5.000000000000004441 ) ;
#17742=FACE_OUTER_BOUND ( 'NONE', #22478, .T. ) ;
#17744=CARTESIAN_POINT ( 'NONE',  ( 104.9999999999999716, 1.449011120738813565E-14, 1.625000002731184834 ) ) ;
#17747=FACE_OUTER_BOUND ( 'NONE', #23804, .T. ) ;
#17754=CARTESIAN_POINT ( 'NONE',  ( 103.1528011352953342, 3.152801135295383084, 10.06250000136559208 ) ) ;
#17757=CARTESIAN_POINT ( 'NONE',  ( 99.99999999999995737, 4.458734125000016313, 8.187500001365592084 ) ) ;
#17766=DIRECTION ( 'NONE',  ( 0.000000000000000000, 0.000000000000000000, 1.000000000000000000 ) ) ;
#17773=CARTESIAN_POINT ( 'NONE',  ( 97.92893218813451028, 5.000000000000018652, 8.937500002731184168 ) ) ;
#17798=CARTESIAN_POINT ( 'NONE',  ( 101.8468681455907046, -4.458734124999987891, 1.750000001365591862 ) ) ;
#17814=CARTESIAN_POINT ( 'NONE',  ( 95.54126587499996504, 1.387778780781445676E-14, 0.6875000013655923059 ) ) ;
#17819=DIRECTION ( 'NONE',  ( -0.000000000000000000, -0.000000000000000000, -1.000000000000000000 ) ) ;
#17826=CARTESIAN_POINT ( 'NONE',  ( 96.84719886470459471, -3.152801135295355994, 10.81250000136559208 ) ) ;
#17829=CARTESIAN_POINT ( 'NONE',  ( 95.54126587499995082, 1.846868145590750077, 1.375000001365592972 ) ) ;
#17846=CARTESIAN_POINT ( 'NONE',  ( 104.4587341249999781, 1.846868145590750299, 11.25000000136559208 ) ) ;
#17863=CARTESIAN_POINT ( 'NONE',  ( 98.15313185440923860, 4.458734125000016313, 11.50000000136559208 ) ) ;
#17867=CARTESIAN_POINT ( 'NONE',  ( 94.99999999999997158, -2.071067811865486608, 2.062499999999999556 ) ) ;
#17878=EDGE_CURVE ( 'NONE', #27159, #19876, #24255, .T. ) ;
#17879=STYLED_ITEM ( 'NONE', ( #24298 ), #26591 ) ;
#17882=CARTESIAN_POINT ( 'NONE',  ( 94.99999999999995737, 1.387778780781445676E-14, 11.12500000273118594 ) ) ;
#17883=SHAPE_REPRESENTATION ( 'connector', ( #26844 ), #20877 ) ;
#17892=CARTESIAN_POINT ( 'NONE',  ( 95.54126587499995082, 1.846868145590750077, 3.375000001365592972 ) ) ;
#17895=CARTESIAN_POINT ( 'NONE',  ( 103.1528011352953342, -3.152801135295355106, 9.812500001365593860 ) ) ;
#17912=CARTESIAN_POINT ( 'NONE',  ( 96.46446609406721961, -3.535533905932727539, 8.250000002731185944 ) ) ;
#17917=CARTESIAN_POINT ( 'NONE',  ( 103.5355339059327093, 3.535533905932755072, 2.624999999999998668 ) ) ;
#17952=ORIENTED_EDGE ( 'NONE', *, *, #20584, .T. ) ;
#17954=CARTESIAN_POINT ( 'NONE',  ( 94.99999999999995737, 1.387778780781445676E-14, 15.00000000000000000 ) ) ;
#17969=CARTESIAN_POINT ( 'NONE',  ( 98.15313185440925281, 4.458734125000016313, 12.50000000136559208 ) ) ;
#17972=CARTESIAN_POINT ( 'NONE',  ( 101.8468681455906903, -4.458734124999987891, 0.7500000013655925279 ) ) ;
#17975=CARTESIAN_POINT ( 'NONE',  ( 96.46446609406721961, 3.535533905932755072, 3.875000000000000000 ) ) ;
#17982=ORIENTED_EDGE ( 'NONE', *, *, #7051, .T. ) ;
#17984=CARTESIAN_POINT ( 'NONE',  ( 95.54126587499995082, 1.846868145590750077, 12.62500000136559208 ) ) ;
#18003=CARTESIAN_POINT ( 'NONE',  ( 96.84719886470459471, 3.152801135295383084, 6.562500001365592084 ) ) ;
#18020=CARTESIAN_POINT ( 'NONE',  ( 102.0710678118654329, 5.000000000000018652, 10.81250000273118417 ) ) ;
#18028=CARTESIAN_POINT ( 'NONE',  ( 103.1528011352953342, 3.152801135295383084, 6.062500001365592084 ) ) ;
#18032=CARTESIAN_POINT ( 'NONE',  ( 99.99999999999995737, -4.458734124999988779, 9.687500001365593860 ) ) ;
#18050=CARTESIAN_POINT ( 'NONE',  ( 102.0710678118654329, -4.999999999999989342, 10.43750000273118417 ) ) ;
#18063=CARTESIAN_POINT ( 'NONE',  ( 94.99999999999995737, 1.387778780781445676E-14, 12.12500000273118594 ) ) ;
#18064=CARTESIAN_POINT ( 'NONE',  ( 104.9999999999999716, 1.449011120738813565E-14, 1.625000002731184834 ) ) ;
#18096=CARTESIAN_POINT ( 'NONE',  ( 98.15313185440925281, -4.458734124999987891, 0.8750000013655926390 ) ) ;
#18111=CARTESIAN_POINT ( 'NONE',  ( 96.84719886470459471, -3.152801135295355994, 7.812500001365592084 ) ) ;
#18113=CARTESIAN_POINT ( 'NONE',  ( 98.15313185440923860, 4.458734125000016313, 10.25000000136559031 ) ) ;
#18128=CARTESIAN_POINT ( 'NONE',  ( 98.15313185440925281, 4.458734125000016313, 10.50000000136559208 ) ) ;
#18129=ORIENTED_EDGE ( 'NONE', *, *, #27140, .F. ) ;
#18146=CARTESIAN_POINT ( 'NONE',  ( 103.1528011352953342, 3.152801135295383084, 6.312500001365592084 ) ) ;
#18156=AXIS2_PLACEMENT_3D ( 'NONE', #18245, #1015, #10324 ) ;
#18173=DIRECTION ( 'NONE',  ( -0.000000000000000000, -0.000000000000000000, -1.000000000000000000 ) ) ;
#18177=CARTESIAN_POINT ( 'NONE',  ( 96.84719886470459471, -3.152801135295355994, 3.562500001365591196 ) ) ;
#18180=CARTESIAN_POINT ( 'NONE',  ( 98.15313185440925281, 4.458734125000016313, 6.250000001365592084 ) ) ;
#18192=ORIENTED_EDGE ( 'NONE', *, *, #3035, .T. ) ;
#18196=CARTESIAN_POINT ( 'NONE',  ( 94.99999999999995737, 1.387778780781445676E-14, 10.12500000273118594 ) ) ;
#18245=CARTESIAN_POINT ( 'NONE',  ( 99.99999999999995737, 1.387778780781445676E-14, 34.79898987322334136 ) ) ;
#18247=CARTESIAN_POINT ( 'NONE',  ( 104.9999999999999716, 1.449011120738813565E-14, 14.49999999999999822 ) ) ;
#18252=CARTESIAN_POINT ( 'NONE',  ( 97.92893218813451028, -4.999999999999989342, 13.31250000273118772 ) ) ;
#18253=PLANE ( 'NONE',  #25282 ) ;
#18260=CARTESIAN_POINT ( 'NONE',  ( 104.4587341249999639, 1.442382525525748735E-14, 5.187500001365592972 ) ) ;
#18263=CARTESIAN_POINT ( 'NONE',  ( 95.54126587499996504, 1.846868145590750077, 8.375000001365592084 ) ) ;
#18266=CARTESIAN_POINT ( 'NONE',  ( 103.5355339059327093, 3.535533905932755072, 3.624999999999999556 ) ) ;
#18272=CARTESIAN_POINT ( 'NONE',  ( 102.0710678118654329, -4.999999999999989342, 1.312499999999999334 ) ) ;
#18278=CARTESIAN_POINT ( 'NONE',  ( 96.84719886470459471, -3.152801135295355994, 9.812500001365593860 ) ) ;
#18279=ORIENTED_EDGE ( 'NONE', *, *, #7755, .F. ) ;
#18293=CARTESIAN_POINT ( 'NONE',  ( 99.99999999999995737, 4.458734125000016313, 6.437500001365592084 ) ) ;
#18295=CARTESIAN_POINT ( 'NONE',  ( 94.99999999999995737, 1.387778780781445676E-14, 1.999999999999998224 ) ) ;
#18312=CARTESIAN_POINT ( 'NONE',  ( 97.92893218813451028, -4.999999999999989342, 13.18750000000000000 ) ) ;
#18313=CARTESIAN_POINT ( 'NONE',  ( 104.9999999999999716, 2.071067811865491937, 8.687500002731184168 ) ) ;
#18314=CARTESIAN_POINT ( 'NONE',  ( 99.99999999999995737, 1.387778780781445676E-14, 34.79898987322334136 ) ) ;
#18324=CARTESIAN_POINT ( 'NONE',  ( 99.99999999999995737, 4.458734125000016313, 5.187500001365592972 ) ) ;
#18327=CARTESIAN_POINT ( 'NONE',  ( 96.84719886470459471, -3.152801135295355994, 8.562500001365592084 ) ) ;
#18338=AXIS2_PLACEMENT_3D ( 'NONE', #17600, #24444, #26305 ) ;
#18343=CARTESIAN_POINT ( 'NONE',  ( 96.46446609406721961, 3.535533905932755072, 10.00000000273118594 ) ) ;
#18387=CARTESIAN_POINT ( 'NONE',  ( 94.99999999999995737, 1.387778780781445676E-14, 9.999999999999998224 ) ) ;
#18393=CARTESIAN_POINT ( 'NONE',  ( 96.46446609406721961, -3.535533905932727539, 12.25000000273118594 ) ) ;
#18402=CARTESIAN_POINT ( 'NONE',  ( 95.54126587499995082, 1.846868145590750077, 6.625000001365592084 ) ) ;
#18404=CARTESIAN_POINT ( 'NONE',  ( 95.54126587499996504, 1.846868145590750077, 10.37500000136559208 ) ) ;
#18419=CARTESIAN_POINT ( 'NONE',  ( 98.15313185440925281, -4.458734124999987891, 11.87500000136559031 ) ) ;
#18436=CARTESIAN_POINT ( 'NONE',  ( 104.4587341249999781, 1.846868145590750521, 5.250000001365592972 ) ) ;
#18447=CARTESIAN_POINT ( 'NONE',  ( 94.99999999999995737, 1.387778780781445676E-14, 3.125000002731185944 ) ) ;
#18455=ORIENTED_EDGE ( 'NONE', *, *, #26275, .F. ) ;
#18464=DIRECTION ( 'NONE',  ( -0.000000000000000000, -0.000000000000000000, -1.000000000000000000 ) ) ;
#18469=CARTESIAN_POINT ( 'NONE',  ( 99.99999999999995737, -4.458734124999988779, 13.93750000136559208 ) ) ;
#18470=CARTESIAN_POINT ( 'NONE',  ( 104.9999999999999716, 2.071067811865496822, 12.68750000273118772 ) ) ;
#18471=CARTESIAN_POINT ( 'NONE',  ( 99.99999999999995737, -4.458734124999988779, 2.687500001365592528 ) ) ;
#18486=CARTESIAN_POINT ( 'NONE',  ( 97.92893218813451028, -4.999999999999989342, 5.312500002731184168 ) ) ;
#18491=CARTESIAN_POINT ( 'NONE',  ( 104.9999999999999716, 1.449011120738813565E-14, 13.50000000000000000 ) ) ;
#18520=CARTESIAN_POINT ( 'NONE',  ( 94.99999999999997158, 2.071067811865471953, 7.937500000000001776 ) ) ;
#18530=CARTESIAN_POINT ( 'NONE',  ( 104.9999999999999574, -2.071067811865462627, 7.437500000000000000 ) ) ;
#18536=CARTESIAN_POINT ( 'NONE',  ( 104.9999999999999716, 1.449011120738813565E-14, 13.62500000273118417 ) ) ;
#18537=DIRECTION ( 'NONE',  ( -0.000000000000000000, -0.000000000000000000, -1.000000000000000000 ) ) ;
#18539=CARTESIAN_POINT ( 'NONE',  ( 103.5355339059327093, 3.535533905932755072, 11.75000000273118594 ) ) ;
#18544=CARTESIAN_POINT ( 'NONE',  ( 104.4587341249999781, 1.846868145590750299, 6.250000001365592084 ) ) ;
#18546=CARTESIAN_POINT ( 'NONE',  ( 96.84719886470459471, -3.152801135295355994, 10.56250000136559208 ) ) ;
#18562=CARTESIAN_POINT ( 'NONE',  ( 95.54126587499996504, 1.387778780781445676E-14, 6.687500001365592084 ) ) ;
#18577=CARTESIAN_POINT ( 'NONE',  ( 98.15313185440923860, -4.458734124999987891, 7.875000001365592084 ) ) ;
#18584=DIRECTION ( 'NONE',  ( 1.000000000000000000, 0.000000000000000000, 0.000000000000000000 ) ) ;
#18596=DIRECTION ( 'NONE',  ( -0.000000000000000000, -0.000000000000000000, -1.000000000000000000 ) ) ;
#18601=ADVANCED_FACE ( 'NONE', ( #21697 ), #24108, .F. ) ;
#18607=CARTESIAN_POINT ( 'NONE',  ( 103.1528011352953342, 3.152801135295383084, 2.062500001365591640 ) ) ;
#18620=ORIENTED_EDGE ( 'NONE', *, *, #10798, .F. ) ;
#18625=CARTESIAN_POINT ( 'NONE',  ( 103.5355339059327093, -3.535533905932726206, 5.500000002731185056 ) ) ;
#18641=CARTESIAN_POINT ( 'NONE',  ( 98.15313185440925281, 4.458734125000016313, 13.25000000136559208 ) ) ;
#18659=ORIENTED_EDGE ( 'NONE', *, *, #1180, .F. ) ;
#18670=CARTESIAN_POINT ( 'NONE',  ( 104.9999999999999574, -2.071067811865462627, 9.437500000000000000 ) ) ;
#18675=CARTESIAN_POINT ( 'NONE',  ( 96.46446609406721961, 3.535533905932755072, 1.000000002731185944 ) ) ;
#18683=CARTESIAN_POINT ( 'NONE',  ( 96.84719886470459471, 3.152801135295383084, 8.562500001365592084 ) ) ;
#18685=CARTESIAN_POINT ( 'NONE',  ( 104.4587341249999781, -1.846868145590721655, 9.875000001365593860 ) ) ;
#18697=CARTESIAN_POINT ( 'NONE',  ( 101.8468681455906903, 4.458734125000016313, 6.375000001365592084 ) ) ;
#18709=CARTESIAN_POINT ( 'NONE',  ( 95.54126587499996504, 1.387778780781445676E-14, 1.687500001365591418 ) ) ;
#18726=VERTEX_POINT ( 'NONE', #11259 ) ;
#18742=ORIENTED_EDGE ( 'NONE', *, *, #10555, .F. ) ;
#18743=CARTESIAN_POINT ( 'NONE',  ( 104.4587341249999781, 1.846868145590750299, 1.000000001365592528 ) ) ;
#18752=LINE ( 'NONE', #1650, #6310 ) ;
#18759=CARTESIAN_POINT ( 'NONE',  ( 102.0710678118654329, 5.000000000000018652, 5.812500002731185056 ) ) ;
#18768=CARTESIAN_POINT ( 'NONE',  ( 95.54126587499996504, 1.387778780781445676E-14, 14.56250000136559208 ) ) ;
#18775=CARTESIAN_POINT ( 'NONE',  ( 104.4587341249999781, -1.846868145590721655, 13.87500000136559208 ) ) ;
#18801=CARTESIAN_POINT ( 'NONE',  ( 103.5355339059327093, 3.535533905932755072, 10.62499999999999822 ) ) ;
#18806=CARTESIAN_POINT ( 'NONE',  ( 94.99999999999995737, 1.387778780781445676E-14, 12.12500000273118594 ) ) ;
#18809=CARTESIAN_POINT ( 'NONE',  ( 94.99999999999995737, 2.071067811865491493, 12.06250000273118950 ) ) ;
#18815=CARTESIAN_POINT ( 'NONE',  ( 96.84719886470459471, 3.152801135295383084, 4.562500001365592084 ) ) ;
#18817=CARTESIAN_POINT ( 'NONE',  ( 95.54126587499996504, 1.387778780781445676E-14, 6.437500001365592084 ) ) ;
#18829=CARTESIAN_POINT ( 'NONE',  ( 101.8468681455906903, 4.458734125000016313, 7.375000001365592084 ) ) ;
#18830=EDGE_CURVE ( 'NONE', #26423, #11228, #24389, .T. ) ;
#18844=CARTESIAN_POINT ( 'NONE',  ( 101.8468681455907046, 4.458734125000016313, 1.375000001365592972 ) ) ;
#18861=CARTESIAN_POINT ( 'NONE',  ( 104.9999999999999574, 2.071067811865511032, 1.687500002731185944 ) ) ;
#18865=ADVANCED_FACE ( 'NONE', ( #599 ), #2737, .F. ) ;
#18867=CARTESIAN_POINT ( 'NONE',  ( 94.99999999999995737, 1.387778780781445676E-14, 6.999999999999999112 ) ) ;
#18868=CARTESIAN_POINT ( 'NONE',  ( 99.99999999999995737, 1.387778780781445676E-14, 34.79898987322334136 ) ) ;
#18874=CARTESIAN_POINT ( 'NONE',  ( 96.46446609406721961, 3.535533905932755072, 13.87499999999999822 ) ) ;
#18880=LINE ( 'NONE', #27590, #21394 ) ;
#18886=CARTESIAN_POINT ( 'NONE',  ( 97.92893218813451028, -4.999999999999989342, 6.312500002731185056 ) ) ;
#18893=EDGE_CURVE ( 'NONE', #6644, #26730, #13618, .T. ) ;
#18906=CARTESIAN_POINT ( 'NONE',  ( 95.54126587499995082, 1.846868145590750077, 13.37500000136559386 ) ) ;
#18912=CARTESIAN_POINT ( 'NONE',  ( 97.92893218813451028, 5.000000000000018652, 8.812500000000000000 ) ) ;
#18924=ORIENTED_EDGE ( 'NONE', *, *, #24657, .F. ) ;
#18934=CARTESIAN_POINT ( 'NONE',  ( 99.99999999999995737, -4.999999999999990230, 11.25000000000000000 ) ) ;
#18948=CARTESIAN_POINT ( 'NONE',  ( 98.15313185440925281, -4.458734124999987891, 1.875000001365591862 ) ) ;
#18950=CARTESIAN_POINT ( 'NONE',  ( 101.8468681455907046, 4.458734125000016313, 8.125000001365592084 ) ) ;
#18966=CARTESIAN_POINT ( 'NONE',  ( 104.4587341249999781, -1.846868145590721655, 7.125000001365592084 ) ) ;
#18967=ORIENTED_EDGE ( 'NONE', *, *, #17878, .T. ) ;
#18980=CARTESIAN_POINT ( 'NONE',  ( 104.4587341249999781, 1.846868145590750299, 4.000000001365592084 ) ) ;
#18982=CARTESIAN_POINT ( 'NONE',  ( 101.8468681455907046, -4.458734124999987891, 5.000000001365592972 ) ) ;
#19024=CARTESIAN_POINT ( 'NONE',  ( 97.92893218813451028, 5.000000000000018652, 1.937500002731185500 ) ) ;
#19031=CARTESIAN_POINT ( 'NONE',  ( 102.0710678118654329, -4.999999999999989342, 9.437500002731184168 ) ) ;
#19039=CARTESIAN_POINT ( 'NONE',  ( 104.9999999999999716, 1.449011120738813565E-14, 10.49999999999999822 ) ) ;
#19041=EDGE_CURVE ( 'NONE', #11228, #27159, #27306, .T. ) ;
#19044=CARTESIAN_POINT ( 'NONE',  ( 96.84719886470459471, 3.152801135295383084, 11.31250000136559208 ) ) ;
#19057=EDGE_CURVE ( 'NONE', #7211, #6644, #19460, .T. ) ;
#19074=CARTESIAN_POINT ( 'NONE',  ( 103.5355339059327093, 3.535533905932755072, 3.624999999999999556 ) ) ;
#19076=CARTESIAN_POINT ( 'NONE',  ( 104.9999999999999574, 2.071067811865511032, 1.562500000000000444 ) ) ;
#19078=CARTESIAN_POINT ( 'NONE',  ( 104.9999999999999716, 1.449011120738813565E-14, 0.000000000000000000 ) ) ;
#19081=CARTESIAN_POINT ( 'NONE',  ( 94.99999999999995737, 1.387778780781445676E-14, 9.000000000000000000 ) ) ;
#19088=CARTESIAN_POINT ( 'NONE',  ( 99.99999999999995737, 4.458734125000016313, 2.437500001365592084 ) ) ;
#19090=CARTESIAN_POINT ( 'NONE',  ( 103.1528011352953342, -3.152801135295355106, 6.812500001365592084 ) ) ;
#19108=CARTESIAN_POINT ( 'NONE',  ( 104.4587341249999781, 1.846868145590750299, 5.250000001365592972 ) ) ;
#19124=CARTESIAN_POINT ( 'NONE',  ( 104.4587341249999781, 1.846868145590750299, 5.000000001365592972 ) ) ;
#19126=CARTESIAN_POINT ( 'NONE',  ( 96.84719886470459471, -3.152801135295355994, 1.812500001365591640 ) ) ;
#19139=CARTESIAN_POINT ( 'NONE',  ( 99.99999999999995737, -4.999999999999990230, 6.375000002731185944 ) ) ;
#19157=CARTESIAN_POINT ( 'NONE',  ( 103.1528011352953342, -3.152801135295355106, 14.06250000136559208 ) ) ;
#19171=CARTESIAN_POINT ( 'NONE',  ( 104.9999999999999574, 2.071067811865491937, 2.687500002731185500 ) ) ;
#19188=CARTESIAN_POINT ( 'NONE',  ( 96.84719886470459471, 3.152801135295383084, 13.31250000136559386 ) ) ;
#19192=CARTESIAN_POINT ( 'NONE',  ( 103.1528011352953342, -3.152801135295355106, 11.81250000136559208 ) ) ;
#19195=CARTESIAN_POINT ( 'NONE',  ( 99.99999999999995737, 5.000000000000018652, 2.875000002731185944 ) ) ;
#19214=CARTESIAN_POINT ( 'NONE',  ( 99.99999999999995737, 5.000000000000018652, 4.749999999999999112 ) ) ;
#19223=CARTESIAN_POINT ( 'NONE',  ( 94.99999999999995737, 1.387778780781445676E-14, 5.125000002731184168 ) ) ;
#19230=CARTESIAN_POINT ( 'NONE',  ( 98.15313185440925281, -4.458734124999987891, 2.875000001365592084 ) ) ;
#19232=CARTESIAN_POINT ( 'NONE',  ( 101.8468681455907046, -4.458734124999987891, 6.750000001365592084 ) ) ;
#19241=CARTESIAN_POINT ( 'NONE',  ( 104.9999999999999716, 1.449011120738813565E-14, 6.625000002731185944 ) ) ;
#19248=CARTESIAN_POINT ( 'NONE',  ( 95.54126587499995082, 1.846868145590750077, 3.625000001365592972 ) ) ;
#19266=CARTESIAN_POINT ( 'NONE',  ( 101.8468681455906903, -4.458734124999987891, 14.00000000136559208 ) ) ;
#19268=CARTESIAN_POINT ( 'NONE',  ( 98.15313185440925281, -4.458734124999987891, 2.625000001365592084 ) ) ;
#19270=CARTESIAN_POINT ( 'NONE',  ( 99.99999999999995737, 4.458734125000016313, 2.437500001365592084 ) ) ;
#19299=( NAMED_UNIT ( * ) PLANE_ANGLE_UNIT ( ) SI_UNIT ( $, .RADIAN. ) );
#19306=DIRECTION ( 'NONE',  ( -0.000000000000000000, -0.000000000000000000, -1.000000000000000000 ) ) ;
#19312=CARTESIAN_POINT ( 'NONE',  ( 104.9999999999999574, -2.071067811865462627, 1.562500002731185056 ) ) ;
#19320=CARTESIAN_POINT ( 'NONE',  ( 104.9999999999999716, 1.449011120738813565E-14, 4.625000002731185944 ) ) ;
#19325=CARTESIAN_POINT ( 'NONE',  ( 98.15313185440925281, -4.458734124999987891, 8.625000001365593860 ) ) ;
#19329=CARTESIAN_POINT ( 'NONE',  ( 98.15313185440925281, 4.458734125000016313, 10.25000000136559386 ) ) ;
#19339=CARTESIAN_POINT ( 'NONE',  ( 94.99999999999995737, -2.071067811865475949, 11.18750000273118417 ) ) ;
#19344=ADVANCED_FACE ( 'NONE', ( #27802 ), #4134, .F. ) ;
#19352=CARTESIAN_POINT ( 'NONE',  ( 94.99999999999995737, 1.387778780781445676E-14, 6.999999999999999112 ) ) ;
#19353=CARTESIAN_POINT ( 'NONE',  ( 96.46446609406721961, 3.535533905932755072, 1.875000000000000000 ) ) ;
#19357=ORIENTED_EDGE ( 'NONE', *, *, #8563, .T. ) ;
#19359=CARTESIAN_POINT ( 'NONE',  ( 104.9999999999999716, 1.449011120738813565E-14, 10.62500000273118594 ) ) ;
#19366=CARTESIAN_POINT ( 'NONE',  ( 103.1528011352953342, -3.152801135295355106, 2.062500001365591640 ) ) ;
#19369=CARTESIAN_POINT ( 'NONE',  ( 98.15313185440923860, -4.458734124999987891, 6.625000001365592084 ) ) ;
#19384=CARTESIAN_POINT ( 'NONE',  ( 104.4587341249999781, -1.846868145590721655, 1.125000001365592750 ) ) ;
#19398=CARTESIAN_POINT ( 'NONE',  ( 95.54126587499995082, 1.846868145590750077, 14.62500000136559208 ) ) ;
#19401=CARTESIAN_POINT ( 'NONE',  ( 96.84719886470459471, -3.152801135295355994, 4.562500001365592084 ) ) ;
#19436=PRESENTATION_STYLE_ASSIGNMENT (( #12575 ) ) ;
#19437=CARTESIAN_POINT ( 'NONE',  ( 103.1528011352953342, 3.152801135295383084, 10.31250000136559208 ) ) ;
#19451=CARTESIAN_POINT ( 'NONE',  ( 94.99999999999995737, -2.071067811865466624, 1.187500002731184390 ) ) ;
#19460=( BOUNDED_CURVE ( )  B_SPLINE_CURVE ( 2, ( #20554, #27391, #23245, #27114, #7711, #7850, #1307, #23108, #16404 ),
 .UNSPECIFIED., .F., .F. ) 
 B_SPLINE_CURVE_WITH_KNOTS ( ( 3, 2, 2, 2, 3 ),
 ( 0.7500000000000000000, 0.7589285714285713969, 0.7678571428571429047, 0.7767857142857143016, 0.7857142857142856984 ),
 .UNSPECIFIED. ) 
 CURVE ( )  GEOMETRIC_REPRESENTATION_ITEM ( )  RATIONAL_B_SPLINE_CURVE ( ( 1.000000000000000000, 0.9238795325112867385, 1.000000000000000000, 0.9238795325112867385, 1.000000000000000000, 0.9238795325112867385, 1.000000000000000000, 0.9238795325112867385, 1.000000000000000000 ) ) 
 REPRESENTATION_ITEM ( '' )  );
#19469=CARTESIAN_POINT ( 'NONE',  ( 99.99999999999995737, 4.458734125000016313, 9.187500001365592084 ) ) ;
#19471=CARTESIAN_POINT ( 'NONE',  ( 104.4587341249999781, 1.846868145590750299, 14.00000000136559208 ) ) ;
#19481=CARTESIAN_POINT ( 'NONE',  ( 94.99999999999995737, 1.387778780781445676E-14, 0.9999999999999991118 ) ) ;
#19494=CARTESIAN_POINT ( 'NONE',  ( 99.99999999999995737, -4.999999999999990230, 5.249999999999999112 ) ) ;
#19510=LINE ( 'NONE', #14074, #14667 ) ;
#19512=CARTESIAN_POINT ( 'NONE',  ( 95.54126587499996504, -1.846868145590724986, 3.500000001365591196 ) ) ;
#19528=CARTESIAN_POINT ( 'NONE',  ( 104.4587341249999781, 1.846868145590750299, 2.250000001365591640 ) ) ;
#19544=CARTESIAN_POINT ( 'NONE',  ( 96.84719886470459471, -3.152801135295355994, 9.812500001365593860 ) ) ;
#19546=CARTESIAN_POINT ( 'NONE',  ( 101.8468681455907046, -4.458734124999987891, 12.75000000136559208 ) ) ;
#19553=ORIENTED_EDGE ( 'NONE', *, *, #17680, .F. ) ;
#19559=CARTESIAN_POINT ( 'NONE',  ( 104.9999999999999716, 1.449011120738813565E-14, 7.625000002731185056 ) ) ;
#19561=CARTESIAN_POINT ( 'NONE',  ( 95.54126587499996504, 1.387778780781445676E-14, 14.68750000136559208 ) ) ;
#19574=EDGE_CURVE ( 'NONE', #896, #7211, #10866, .T. ) ;
#19577=CARTESIAN_POINT ( 'NONE',  ( 101.8468681455907046, 4.458734125000016313, 10.37500000136559208 ) ) ;
#19591=CARTESIAN_POINT ( 'NONE',  ( 94.99999999999995737, 1.387778780781445676E-14, 3.125000002731185944 ) ) ;
#19606=CARTESIAN_POINT ( 'NONE',  ( 103.1528011352953342, -3.152801135295355106, 7.812500001365592084 ) ) ;
#19609=CARTESIAN_POINT ( 'NONE',  ( 96.84719886470459471, -3.152801135295355994, 13.56250000136559208 ) ) ;
#19633=CARTESIAN_POINT ( 'NONE',  ( 94.99999999999995737, 1.387778780781445676E-14, 4.999999999999999112 ) ) ;
#19667=CARTESIAN_POINT ( 'NONE',  ( 104.4587341249999781, -1.846868145590721655, 3.125000001365592528 ) ) ;
#19681=CARTESIAN_POINT ( 'NONE',  ( 104.4587341249999781, 1.846868145590750299, 10.25000000136559386 ) ) ;
#19683=CARTESIAN_POINT ( 'NONE',  ( 96.84719886470459471, 3.152801135295383084, 12.31250000136559208 ) ) ;
#19685=CARTESIAN_POINT ( 'NONE',  ( 96.84719886470459471, -3.152801135295355994, 0.8125000013655924169 ) ) ;
#19696=ORIENTED_EDGE ( 'NONE', *, *, #27140, .T. ) ;
#19698=CARTESIAN_POINT ( 'NONE',  ( 99.99999999999995737, 1.387778780781445676E-14, 34.79898987322334136 ) ) ;
#19699=CARTESIAN_POINT ( 'NONE',  ( 95.54126587499995082, 1.846868145590750077, 14.62500000136559208 ) ) ;
#19715=CARTESIAN_POINT ( 'NONE',  ( 95.54126587499996504, -1.846868145590724986, 10.75000000136559208 ) ) ;
#19721=CARTESIAN_POINT ( 'NONE',  ( 104.9999999999999716, -2.071067811865467956, 12.43749999999999645 ) ) ;
#19728=ORIENTED_EDGE ( 'NONE', *, *, #5382, .F. ) ;
#19745=CARTESIAN_POINT ( 'NONE',  ( 96.84719886470459471, -3.152801135295355994, 10.56250000136559208 ) ) ;
#19748=CARTESIAN_POINT ( 'NONE',  ( 104.4587341249999639, 1.442382525525748735E-14, 12.93750000136559208 ) ) ;
#19768=EDGE_CURVE ( 'NONE', #22244, #27294, #3964, .T. ) ;
#19773=CARTESIAN_POINT ( 'NONE',  ( 104.9999999999999574, -2.071067811865462627, 1.437499999999999778 ) ) ;
#19781=CARTESIAN_POINT ( 'NONE',  ( 104.9999999999999716, 1.449011120738813565E-14, 6.499999999999999112 ) ) ;
#19792=CARTESIAN_POINT ( 'NONE',  ( 96.84719886470459471, -3.152801135295355994, 3.562500001365591196 ) ) ;
#19810=CARTESIAN_POINT ( 'NONE',  ( 99.99999999999995737, 4.458734125000016313, 3.437500001365592972 ) ) ;
#19824=CARTESIAN_POINT ( 'NONE',  ( 99.99999999999995737, 4.458734125000016313, 10.43750000136559208 ) ) ;
#19826=CARTESIAN_POINT ( 'NONE',  ( 102.0710678118654329, 5.000000000000018652, 3.812500002731185056 ) ) ;
#19835=CARTESIAN_POINT ( 'NONE',  ( 104.9999999999999858, -2.071067811865457298, 12.56250000273118594 ) ) ;
#19841=CARTESIAN_POINT ( 'NONE',  ( 104.4587341249999639, 1.442382525525748735E-14, 13.18750000136559208 ) ) ;
#19857=PRODUCT_CONTEXT ( 'NONE', #4974, 'mechanical' ) ;
#19858=CARTESIAN_POINT ( 'NONE',  ( 104.4587341249999781, -1.846868145590721655, 9.125000001365592084 ) ) ;
#19864=AXIS2_PLACEMENT_3D ( 'NONE', #22444, #3761, #6172 ) ;
#19876=VERTEX_POINT ( 'NONE', #28042 ) ;
#19877=CARTESIAN_POINT ( 'NONE',  ( 99.99999999999995737, 1.387778780781445676E-14, 34.79898987322334136 ) ) ;
#19880=CARTESIAN_POINT ( 'NONE',  ( 96.46446609406721961, -3.535533905932727539, 1.250000002731184390 ) ) ;
#19885=DIRECTION ( 'NONE',  ( -0.000000000000000000, -0.000000000000000000, -1.000000000000000000 ) ) ;
#19891=CARTESIAN_POINT ( 'NONE',  ( 101.8468681455906903, -4.458734124999987891, 7.750000001365592084 ) ) ;
#19894=CARTESIAN_POINT ( 'NONE',  ( 99.99999999999995737, -4.458734124999988779, 8.687500001365592084 ) ) ;
#19905=CARTESIAN_POINT ( 'NONE',  ( 102.0710678118654329, -4.999999999999989342, 11.43750000273118772 ) ) ;
#19913=CARTESIAN_POINT ( 'NONE',  ( 103.5355339059327093, 3.535533905932755072, 10.75000000273118594 ) ) ;
#19918=CARTESIAN_POINT ( 'NONE',  ( 94.99999999999995737, 2.071067811865491048, 1.937500000000000000 ) ) ;
#19939=CARTESIAN_POINT ( 'NONE',  ( 101.8468681455907046, 4.458734125000016313, 4.125000001365592084 ) ) ;
#19958=CARTESIAN_POINT ( 'NONE',  ( 97.92893218813451028, -4.999999999999989342, 13.18749999999999822 ) ) ;
#19973=CARTESIAN_POINT ( 'NONE',  ( 98.15313185440925281, 4.458734125000016313, 11.50000000136559208 ) ) ;
#19975=CARTESIAN_POINT ( 'NONE',  ( 99.99999999999995737, 4.458734125000016313, 1.187500001365592750 ) ) ;
#19978=CARTESIAN_POINT ( 'NONE',  ( 104.9999999999999716, 1.449011120738813565E-14, 12.62500000273118594 ) ) ;
#19991=CARTESIAN_POINT ( 'NONE',  ( 95.54126587499995082, -1.846868145590724986, 10.75000000136559208 ) ) ;
#19992=ORIENTED_EDGE ( 'NONE', *, *, #12726, .F. ) ;
#20007=EDGE_LOOP ( 'NONE', ( #11119, #12636, #18620, #25305, #9323, #6868, #24517, #9491, #21123, #7238, #14709, #8789, #7611, #22855, #26709, #17003, #9463, #14950, #11598, #10214, #19992, #19553, #15279, #18129, #17235, #4913, #14681, #26687, #10087, #2705, #20091 ) ) ;
#20009=CARTESIAN_POINT ( 'NONE',  ( 99.99999999999995737, -4.458734124999988779, 11.93750000136559208 ) ) ;
#20028=CARTESIAN_POINT ( 'NONE',  ( 97.92893218813451028, 5.000000000000018652, 10.93750000273118417 ) ) ;
#20033=CARTESIAN_POINT ( 'NONE',  ( 99.99999999999995737, -4.999999999999990230, 2.375000002731185500 ) ) ;
#20037=ORIENTED_EDGE ( 'NONE', *, *, #3443, .T. ) ;
#20038=CARTESIAN_POINT ( 'NONE',  ( 98.15313185440925281, 4.458734125000016313, 6.250000001365592084 ) ) ;
#20039=EDGE_LOOP ( 'NONE', ( #16688, #2709 ) ) ;
#20041=CARTESIAN_POINT ( 'NONE',  ( 95.54126587499995082, -1.846868145590724986, 8.500000001365592084 ) ) ;
#20058=CARTESIAN_POINT ( 'NONE',  ( 104.9999999999999574, -2.071067811865462627, 8.562500002731184168 ) ) ;
#20074=CARTESIAN_POINT ( 'NONE',  ( 104.9999999999999716, 1.449011120738813565E-14, 15.00000000000000000 ) ) ;
#20091=ORIENTED_EDGE ( 'NONE', *, *, #4310, .F. ) ;
#20098=( BOUNDED_CURVE ( )  B_SPLINE_CURVE ( 2, ( #17744, #2786, #14018, #26445, #509, #9611, #19880, #13441, #24729 ),
 .UNSPECIFIED., .F., .T. ) 
 B_SPLINE_CURVE_WITH_KNOTS ( ( 3, 2, 2, 2, 3 ),
 ( 0.8928571428571427937, 0.9017857142857141906, 0.9107142857142855874, 0.9196428571428569843, 0.9285714285714284921 ),
 .UNSPECIFIED. ) 
 CURVE ( )  GEOMETRIC_REPRESENTATION_ITEM ( )  RATIONAL_B_SPLINE_CURVE ( ( 1.000000000000000888, 0.9238795325112857393, 1.000000000000000000, 0.9238795325112867385, 1.000000000000000000, 0.9238795325112867385, 1.000000000000000000, 0.9238795325112877377, 0.9999999999999990008 ) ) 
 REPRESENTATION_ITEM ( '' )  );
#20103=CARTESIAN_POINT ( 'NONE',  ( 99.99999999999995737, 5.000000000000018652, 12.75000000000000000 ) ) ;
#20116=CARTESIAN_POINT ( 'NONE',  ( 103.1528011352953342, 3.152801135295383084, 12.31250000136559208 ) ) ;
#20118=CARTESIAN_POINT ( 'NONE',  ( 96.84719886470459471, 3.152801135295383084, 14.31250000136559208 ) ) ;
#20133=CARTESIAN_POINT ( 'NONE',  ( 95.54126587499995082, 1.846868145590750077, 9.625000001365593860 ) ) ;
#20138=EDGE_CURVE ( 'NONE', #9857, #19876, #2803, .T. ) ;
#20151=CARTESIAN_POINT ( 'NONE',  ( 96.84719886470459471, 3.152801135295383084, 8.562500001365592084 ) ) ;
#20154=CARTESIAN_POINT ( 'NONE',  ( 94.99999999999995737, 1.387778780781445676E-14, 34.79898987322334136 ) ) ;
#20169=LINE ( 'NONE', #507, #227 ) ;
#20171=CARTESIAN_POINT ( 'NONE',  ( 104.9999999999999716, -2.071067811865462627, 5.562500002731185056 ) ) ;
#20178=CARTESIAN_POINT ( 'NONE',  ( 103.1528011352953342, -3.152801135295355106, 5.812500001365591196 ) ) ;
#20181=CARTESIAN_POINT ( 'NONE',  ( 103.1528011352953342, -3.152801135295355106, 7.812500001365592084 ) ) ;
#20191=PLANE ( 'NONE',  #8777 ) ;
#20197=CARTESIAN_POINT ( 'NONE',  ( 94.99999999999995737, 2.071067811865491048, 10.06250000273118417 ) ) ;
#20211=LINE ( 'NONE', #844, #119 ) ;
#20240=CARTESIAN_POINT ( 'NONE',  ( 99.99999999999995737, -4.999999999999990230, 12.25000000000000000 ) ) ;
#20245=CARTESIAN_POINT ( 'NONE',  ( 95.27063293749995410, 1.387778780781445676E-14, 0.8437500006827957089 ) ) ;
#20247=DIRECTION ( 'NONE',  ( -1.000000000000000000, 0.000000000000000000, 0.000000000000000000 ) ) ;
#20251=CARTESIAN_POINT ( 'NONE',  ( 99.99999999999995737, 4.458734125000016313, 6.437500001365592084 ) ) ;
#20254=AXIS2_PLACEMENT_3D ( 'NONE', #14740, #7923, #14604 ) ;
#20255=CARTESIAN_POINT ( 'NONE',  ( 104.4587341249999781, -1.846868145590721655, 11.87500000136559208 ) ) ;
#20269=CARTESIAN_POINT ( 'NONE',  ( 95.54126587499995082, -1.846868145590724986, 11.75000000136559208 ) ) ;
#20287=CARTESIAN_POINT ( 'NONE',  ( 95.54126587499996504, 1.387778780781445676E-14, 6.687500001365592084 ) ) ;
#20291=DIRECTION ( 'NONE',  ( -0.000000000000000000, -0.000000000000000000, -1.000000000000000000 ) ) ;
#20311=CARTESIAN_POINT ( 'NONE',  ( 94.99999999999995737, 1.387778780781445676E-14, 5.125000002731184168 ) ) ;
#20314=CARTESIAN_POINT ( 'NONE',  ( 104.9999999999999716, 1.449011120738813565E-14, 2.625000002731185500 ) ) ;
#20319=CARTESIAN_POINT ( 'NONE',  ( 98.15313185440925281, 4.458734125000016313, 4.250000001365592084 ) ) ;
#20322=CARTESIAN_POINT ( 'NONE',  ( 96.46446609406721961, 3.535533905932755072, 13.00000000273118417 ) ) ;
#20323=CARTESIAN_POINT ( 'NONE',  ( 101.8468681455906903, -4.458734124999987891, 9.750000001365593860 ) ) ;
#20328=CARTESIAN_POINT ( 'NONE',  ( 96.46446609406721961, -3.535533905932727539, 5.124999999999999112 ) ) ;
#20331=EDGE_CURVE ( 'NONE', #14666, #22034, #26381, .T. ) ;
#20343=CARTESIAN_POINT ( 'NONE',  ( 96.46446609406721961, -3.535533905932727539, 9.250000002731184168 ) ) ;
#20350=CARTESIAN_POINT ( 'NONE',  ( 99.99999999999995737, 5.000000000000018652, 1.749999999999999778 ) ) ;
#20365=EDGE_CURVE ( 'NONE', #6963, #10159, #3647, .T. ) ;
#20387=CARTESIAN_POINT ( 'NONE',  ( 104.9999999999999574, -2.071067811865462627, 14.43749999999999822 ) ) ;
#20402=CARTESIAN_POINT ( 'NONE',  ( 98.15313185440925281, 4.458734125000016313, 8.500000001365592084 ) ) ;
#20404=CARTESIAN_POINT ( 'NONE',  ( 103.1528011352953342, 3.152801135295383084, 12.06250000136559208 ) ) ;
#20407=CARTESIAN_POINT ( 'NONE',  ( 97.92893218813451028, 5.000000000000018652, 3.812500000000000000 ) ) ;
#20412=LINE ( 'NONE', #7717, #2937 ) ;
#20417=CARTESIAN_POINT ( 'NONE',  ( 104.4587341249999781, 1.846868145590750299, 9.250000001365593860 ) ) ;
#20437=CARTESIAN_POINT ( 'NONE',  ( 96.84719886470459471, -3.152801135295355994, 6.812500001365592084 ) ) ;
#20456=CARTESIAN_POINT ( 'NONE',  ( 103.5355339059327093, 3.535533905932755072, 8.750000002731184168 ) ) ;
#20462=CARTESIAN_POINT ( 'NONE',  ( 97.92893218813451028, -4.999999999999989342, 7.187499999999999112 ) ) ;
#20469=CARTESIAN_POINT ( 'NONE',  ( 103.1528011352953342, -3.152801135295355106, 2.812500001365592528 ) ) ;
#20472=CARTESIAN_POINT ( 'NONE',  ( 101.8468681455906903, -4.458734124999987891, 8.750000001365592084 ) ) ;
#20480=DIRECTION ( 'NONE',  ( -0.000000000000000000, -0.000000000000000000, -1.000000000000000000 ) ) ;
#20488=CARTESIAN_POINT ( 'NONE',  ( 104.9999999999999574, 2.071067811865491937, 8.687500002731184168 ) ) ;
#20504=CARTESIAN_POINT ( 'NONE',  ( 102.0710678118654329, 5.000000000000018652, 12.68750000000000178 ) ) ;
#20532=ORIENTED_EDGE ( 'NONE', *, *, #27487, .T. ) ;
#20534=CARTESIAN_POINT ( 'NONE',  ( 102.0710678118654329, -4.999999999999989342, 11.31249999999999822 ) ) ;
#20540=CARTESIAN_POINT ( 'NONE',  ( 103.5355339059327093, 3.535533905932755072, 13.75000000273118594 ) ) ;
#20548=CARTESIAN_POINT ( 'NONE',  ( 103.1528011352953342, -3.152801135295355106, 7.062500001365592972 ) ) ;
#20551=CARTESIAN_POINT ( 'NONE',  ( 99.99999999999995737, 4.458734125000016313, 10.18750000136559208 ) ) ;
#20554=CARTESIAN_POINT ( 'NONE',  ( 104.9999999999999716, 1.449011120738813565E-14, 4.499999999999999112 ) ) ;
#20560=CARTESIAN_POINT ( 'NONE',  ( 104.9999999999999716, 1.449011120738813565E-14, 1.499999999999999556 ) ) ;
#20562=EDGE_LOOP ( 'NONE', ( #12221, #5326 ) ) ;
#20565=CARTESIAN_POINT ( 'NONE',  ( 99.99999999999995737, 4.458734125000016313, 12.43750000136559208 ) ) ;
#20569=CARTESIAN_POINT ( 'NONE',  ( 95.54126587499996504, 1.387778780781445676E-14, 14.68750000136559208 ) ) ;
#20578=CARTESIAN_POINT ( 'NONE',  ( 99.99999999999995737, 4.458734125000016313, 5.437500001365592972 ) ) ;
#20584=EDGE_CURVE ( 'NONE', #4924, #20673, #1987, .T. ) ;
#20593=CARTESIAN_POINT ( 'NONE',  ( 97.92893218813451028, -4.999999999999989342, 0.3125000027311853334 ) ) ;
#20602=CARTESIAN_POINT ( 'NONE',  ( 104.9999999999999716, 1.449011120738813565E-14, 7.500000000000000000 ) ) ;
#20607=CARTESIAN_POINT ( 'NONE',  ( 101.8468681455906903, 4.458734125000016313, 3.125000001365592528 ) ) ;
#20609=CARTESIAN_POINT ( 'NONE',  ( 97.92893218813451028, 5.000000000000018652, 12.93750000273118772 ) ) ;
#20610=CARTESIAN_POINT ( 'NONE',  ( 103.1528011352953342, 3.152801135295383084, 3.062500001365592528 ) ) ;
#20627=CARTESIAN_POINT ( 'NONE',  ( 99.99999999999995737, -4.999999999999990230, 7.375000002731185944 ) ) ;
#20642=EDGE_CURVE ( 'NONE', #2199, #16509, #4624, .T. ) ;
#20652=DIRECTION ( 'NONE',  ( -0.000000000000000000, -0.000000000000000000, -1.000000000000000000 ) ) ;
#20673=VERTEX_POINT ( 'NONE', #13718 ) ;
#20674=CARTESIAN_POINT ( 'NONE',  ( 94.99999999999995737, 2.071067811865491048, 7.937500000000000888 ) ) ;
#20680=CARTESIAN_POINT ( 'NONE',  ( 104.9999999999999574, 2.071067811865511032, 0.6875000027311864992 ) ) ;
#20689=CARTESIAN_POINT ( 'NONE',  ( 98.15313185440925281, -4.458734124999987891, 7.875000001365591196 ) ) ;
#20691=CARTESIAN_POINT ( 'NONE',  ( 98.15313185440923860, -4.458734124999987891, 11.62500000136559031 ) ) ;
#20694=CARTESIAN_POINT ( 'NONE',  ( 97.92893218813451028, -4.999999999999989342, 9.187500000000000000 ) ) ;
#20706=CARTESIAN_POINT ( 'NONE',  ( 98.15313185440925281, 4.458734125000016313, 7.500000001365592084 ) ) ;
#20719=CARTESIAN_POINT ( 'NONE',  ( 103.1528011352953342, -3.152801135295355106, 8.062500001365592084 ) ) ;
#20722=CARTESIAN_POINT ( 'NONE',  ( 97.92893218813451028, 5.000000000000018652, 6.937500002731185056 ) ) ;
#20728=LINE ( 'NONE', #10013, #17281 ) ;
#20737=ORIENTED_EDGE ( 'NONE', *, *, #15055, .T. ) ;
#20738=CARTESIAN_POINT ( 'NONE',  ( 94.99999999999995737, 2.071067811865491493, 2.062500002731185056 ) ) ;
#20743=CARTESIAN_POINT ( 'NONE',  ( 103.5355339059327093, -3.535533905932726206, 7.375000000000000000 ) ) ;
#20749=CARTESIAN_POINT ( 'NONE',  ( 98.15313185440925281, 4.458734125000016313, 2.250000001365591640 ) ) ;
#20751=CARTESIAN_POINT ( 'NONE',  ( 94.99999999999995737, 1.387778780781445676E-14, 13.99999999999999822 ) ) ;
#20758=ORIENTED_EDGE ( 'NONE', *, *, #26932, .T. ) ;
#20763=CARTESIAN_POINT ( 'NONE',  ( 99.99999999999995737, 5.000000000000018652, 4.875000002731185944 ) ) ;
#20766=( BOUNDED_CURVE ( )  B_SPLINE_CURVE ( 2, ( #25814, #6288, #23685, #4162, #8706, #12822, #26097, #6562, #15242 ),
 .UNSPECIFIED., .F., .F. ) 
 B_SPLINE_CURVE_WITH_KNOTS ( ( 3, 2, 2, 2, 3 ),
 ( 0.3571428571428572063, 0.3660714285714286031, 0.3750000000000000000, 0.3839285714285714524, 0.3928571428571428492 ),
 .UNSPECIFIED. ) 
 CURVE ( )  GEOMETRIC_REPRESENTATION_ITEM ( )  RATIONAL_B_SPLINE_CURVE ( ( 0.9999999999999995559, 0.9238795325112871826, 1.000000000000000000, 0.9238795325112867385, 1.000000000000000000, 0.9238795325112867385, 1.000000000000000000, 0.9238795325112867385, 1.000000000000000000 ) ) 
 REPRESENTATION_ITEM ( '' )  );
#20781=CARTESIAN_POINT ( 'NONE',  ( 98.15313185440925281, 4.458734125000016313, 11.25000000136559031 ) ) ;
#20789=CARTESIAN_POINT ( 'NONE',  ( 94.99999999999995737, 1.387778780781445676E-14, 13.99999999999999822 ) ) ;
#20807=ORIENTED_EDGE ( 'NONE', *, *, #20365, .T. ) ;
#20808=CARTESIAN_POINT ( 'NONE',  ( 99.99999999999995737, 5.000000000000018652, 8.749999999999998224 ) ) ;
#20809=ORIENTED_EDGE ( 'NONE', *, *, #10194, .T. ) ;
#20814=CARTESIAN_POINT ( 'NONE',  ( 99.99999999999995737, 5.000000000000018652, 13.87500000273118594 ) ) ;
#20815=CARTESIAN_POINT ( 'NONE',  ( 97.92893218813451028, -4.999999999999989342, 12.31250000273118772 ) ) ;
#20819=CARTESIAN_POINT ( 'NONE',  ( 103.5355339059327093, -3.535533905932726206, 11.37500000000000000 ) ) ;
#20825=CARTESIAN_POINT ( 'NONE',  ( 96.84719886470459471, -3.152801135295355994, 6.812500001365592084 ) ) ;
#20827=CARTESIAN_POINT ( 'NONE',  ( 96.84719886470459471, 3.152801135295383084, 9.312500001365593860 ) ) ;
#20842=CARTESIAN_POINT ( 'NONE',  ( 98.15313185440925281, 4.458734125000016313, 6.500000001365592084 ) ) ;
#20856=CARTESIAN_POINT ( 'NONE',  ( 95.54126587499996504, 1.846868145590750077, 4.625000001365592084 ) ) ;
#20877=( GEOMETRIC_REPRESENTATION_CONTEXT ( 3 ) GLOBAL_UNCERTAINTY_ASSIGNED_CONTEXT ( ( #8053 ) ) GLOBAL_UNIT_ASSIGNED_CONTEXT ( ( #16875, #19299, #15136 ) ) REPRESENTATION_CONTEXT ( 'NONE', 'WORKASPACE' ) );
#20878=CYLINDRICAL_SURFACE ( 'NONE', #17230, 5.000000000000004441 ) ;
#20886=CARTESIAN_POINT ( 'NONE',  ( 98.15313185440925281, -4.458734124999987891, 13.87500000136559208 ) ) ;
#20887=CARTESIAN_POINT ( 'NONE',  ( 101.8468681455907046, -4.458734124999987891, 14.00000000136559208 ) ) ;
#20889=AXIS2_PLACEMENT_3D ( 'NONE', #22050, #17766, #13035 ) ;
#20905=CARTESIAN_POINT ( 'NONE',  ( 99.99999999999995737, -4.999999999999990230, 4.375000002731185056 ) ) ;
#20913=LINE ( 'NONE', #18768, #4803 ) ;
#20921=CARTESIAN_POINT ( 'NONE',  ( 103.1528011352953342, -3.152801135295355106, 11.81250000136559208 ) ) ;
#20948=CARTESIAN_POINT ( 'NONE',  ( 102.0710678118654329, 5.000000000000018652, 7.687499999999999112 ) ) ;
#20952=CARTESIAN_POINT ( 'NONE',  ( 94.99999999999995737, 1.387778780781445676E-14, 14.12500000273118594 ) ) ;
#20953=CARTESIAN_POINT ( 'NONE',  ( 94.99999999999995737, 1.387778780781445676E-14, 1.125000002731184390 ) ) ;
#20962=CARTESIAN_POINT ( 'NONE',  ( 101.8468681455906903, 4.458734125000016313, 1.375000001365592972 ) ) ;
#20965=CARTESIAN_POINT ( 'NONE',  ( 103.1528011352953342, 3.152801135295383084, 5.062500001365592972 ) ) ;
#20974=( BOUNDED_CURVE ( )  B_SPLINE_CURVE ( 2, ( #9888, #5350, #13730, #9610, #16311, #24584, #20456, #18313, #24728 ),
 .UNSPECIFIED., .F., .F. ) 
 B_SPLINE_CURVE_WITH_KNOTS ( ( 3, 2, 2, 2, 3 ),
 ( 0.3571428571428572063, 0.3660714285714286031, 0.3750000000000000000, 0.3839285714285714524, 0.3928571428571428492 ),
 .UNSPECIFIED. ) 
 CURVE ( )  GEOMETRIC_REPRESENTATION_ITEM ( )  RATIONAL_B_SPLINE_CURVE ( ( 0.9999999999999995559, 0.9238795325112871826, 1.000000000000000000, 0.9238795325112867385, 1.000000000000000000, 0.9238795325112867385, 1.000000000000000000, 0.9238795325112867385, 1.000000000000000000 ) ) 
 REPRESENTATION_ITEM ( '' )  );
#20980=CARTESIAN_POINT ( 'NONE',  ( 101.8468681455906903, -4.458734124999987891, 7.000000001365592972 ) ) ;
#20993=EDGE_CURVE ( 'NONE', #22034, #26723, #27145, .T. ) ;
#20995=CARTESIAN_POINT ( 'NONE',  ( 99.99999999999995737, 4.458734125000016313, 1.437500001365592972 ) ) ;
#21008=CARTESIAN_POINT ( 'NONE',  ( 104.9999999999999716, -2.071067811865462627, 6.562500002731185944 ) ) ;
#21026=CARTESIAN_POINT ( 'NONE',  ( 99.99999999999995737, 4.458734125000016313, 13.43750000136559386 ) ) ;
#21040=CARTESIAN_POINT ( 'NONE',  ( 94.99999999999995737, 1.387778780781445676E-14, 6.125000002731185056 ) ) ;
#21057=FACE_OUTER_BOUND ( 'NONE', #17062, .T. ) ;
#21073=ORIENTED_EDGE ( 'NONE', *, *, #20642, .F. ) ;
#21083=CARTESIAN_POINT ( 'NONE',  ( 97.92893218813451028, 5.000000000000018652, 9.812499999999998224 ) ) ;
#21097=CARTESIAN_POINT ( 'NONE',  ( 96.84719886470459471, -3.152801135295355994, 1.812500001365591640 ) ) ;
#21099=CARTESIAN_POINT ( 'NONE',  ( 95.54126587499996504, -1.846868145590724986, 4.500000001365592084 ) ) ;
#21102=CARTESIAN_POINT ( 'NONE',  ( 103.5355339059327093, -3.535533905932726206, 9.375000000000000000 ) ) ;
#21105=ORIENTED_EDGE ( 'NONE', *, *, #14634, .T. ) ;
#21113=CARTESIAN_POINT ( 'NONE',  ( 103.1528011352953342, 3.152801135295383084, 7.312500001365592084 ) ) ;
#21123=ORIENTED_EDGE ( 'NONE', *, *, #18893, .F. ) ;
#21127=CARTESIAN_POINT ( 'NONE',  ( 95.54126587499995082, -1.846868145590724986, 4.500000001365592084 ) ) ;
#21129=CARTESIAN_POINT ( 'NONE',  ( 103.1528011352953342, -3.152801135295355106, 3.062500001365592528 ) ) ;
#21159=( NAMED_UNIT ( * ) PLANE_ANGLE_UNIT ( ) SI_UNIT ( $, .RADIAN. ) );
#21166=DIRECTION ( 'NONE',  ( -0.000000000000000000, -0.000000000000000000, -1.000000000000000000 ) ) ;
#21176=CARTESIAN_POINT ( 'NONE',  ( 99.99999999999995737, 5.000000000000018652, 3.875000002731185056 ) ) ;
#21193=CARTESIAN_POINT ( 'NONE',  ( 95.54126587499995082, -1.846868145590724986, 11.50000000136559208 ) ) ;
#21200=EDGE_CURVE ( 'NONE', #22694, #14819, #1672, .T. ) ;
#21215=ADVANCED_FACE ( 'NONE', ( #1350 ), #25272, .F. ) ;
#21221=EDGE_LOOP ( 'NONE', ( #18455, #10118, #1181, #1043 ) ) ;
#21222=CARTESIAN_POINT ( 'NONE',  ( 94.99999999999995737, -2.071067811865466624, 10.06249999999999822 ) ) ;
#21231=DIRECTION ( 'NONE',  ( -0.000000000000000000, -0.000000000000000000, 1.000000000000000000 ) ) ;
#21232=VECTOR ( 'NONE', #7526, 1000.000000000000000 ) ;
#21236=CARTESIAN_POINT ( 'NONE',  ( 99.99999999999995737, -4.999999999999990230, 8.375000002731185944 ) ) ;
#21237=CARTESIAN_POINT ( 'NONE',  ( 99.99999999999995737, 4.458734125000016313, 4.437500001365592084 ) ) ;
#21239=CARTESIAN_POINT ( 'NONE',  ( 103.1528011352953342, -3.152801135295355106, 4.812500001365592084 ) ) ;
#21242=AXIS2_PLACEMENT_3D ( 'NONE', #16436, #10143, #8300 ) ;
#21243=DIRECTION ( 'NONE',  ( -0.000000000000000000, -0.000000000000000000, -1.000000000000000000 ) ) ;
#21255=CARTESIAN_POINT ( 'NONE',  ( 104.4587341249999781, 1.846868145590750299, 6.250000001365592084 ) ) ;
#21268=CARTESIAN_POINT ( 'NONE',  ( 104.4587341249999639, 1.442382525525748735E-14, 2.937500001365592528 ) ) ;
#21270=CARTESIAN_POINT ( 'NONE',  ( 96.84719886470459471, 3.152801135295383084, 1.562500001365592972 ) ) ;
#21292=AXIS2_PLACEMENT_3D ( 'NONE', #8700, #21828, #25805 ) ;
#21295=( BOUNDED_CURVE ( )  B_SPLINE_CURVE ( 2, ( #15158, #21751, #23463, #12742, #14882, #8487, #12600, #17453, #23325 ),
 .UNSPECIFIED., .F., .T. ) 
 B_SPLINE_CURVE_WITH_KNOTS ( ( 3, 2, 2, 2, 3 ),
 ( 0.2857142857142856984, 0.2946428571428571508, 0.3035714285714284921, 0.3124999999999999445, 0.3214285714285713969 ),
 .UNSPECIFIED. ) 
 CURVE ( )  GEOMETRIC_REPRESENTATION_ITEM ( )  RATIONAL_B_SPLINE_CURVE ( ( 1.000000000000000000, 0.9238795325112867385, 1.000000000000000000, 0.9238795325112867385, 1.000000000000000000, 0.9238795325112867385, 1.000000000000000000, 0.9238795325112871826, 0.9999999999999995559 ) ) 
 REPRESENTATION_ITEM ( '' )  );
#21308=CARTESIAN_POINT ( 'NONE',  ( 103.5355339059327093, -3.535533905932726206, 6.374999999999999112 ) ) ;
#21315=CARTESIAN_POINT ( 'NONE',  ( 103.1528011352953342, 3.152801135295383084, 14.06250000136559208 ) ) ;
#21321=ORIENTED_EDGE ( 'NONE', *, *, #5151, .T. ) ;
#21336=CARTESIAN_POINT ( 'NONE',  ( 104.9999999999999716, 1.449011120738813565E-14, 12.49999999999999822 ) ) ;
#21337=CARTESIAN_POINT ( 'NONE',  ( 103.5355339059327093, -3.535533905932726206, 13.50000000273118417 ) ) ;
#21338=ORIENTED_EDGE ( 'NONE', *, *, #21370, .T. ) ;
#21349=ORIENTED_EDGE ( 'NONE', *, *, #15599, .T. ) ;
#21359=EDGE_CURVE ( 'NONE', #25944, #8379, #5902, .T. ) ;
#21363=EDGE_LOOP ( 'NONE', ( #19728, #5625, #1489, #11284 ) ) ;
#21366=CARTESIAN_POINT ( 'NONE',  ( 97.92893218813451028, 5.000000000000018652, 4.812500000000000000 ) ) ;
#21370=EDGE_CURVE ( 'NONE', #3896, #13477, #15626, .T. ) ;
#21379=CARTESIAN_POINT ( 'NONE',  ( 97.92893218813451028, -4.999999999999989342, 8.312500002731185944 ) ) ;
#21380=CARTESIAN_POINT ( 'NONE',  ( 95.54126587499995082, -1.846868145590724986, 4.750000001365592084 ) ) ;
#21382=CARTESIAN_POINT ( 'NONE',  ( 103.1528011352953342, -3.152801135295355106, 7.812500001365592084 ) ) ;
#21394=VECTOR ( 'NONE', #16746, 1000.000000000000000 ) ;
#21398=DIRECTION ( 'NONE',  ( -0.000000000000000000, -0.000000000000000000, -1.000000000000000000 ) ) ;
#21400=CARTESIAN_POINT ( 'NONE',  ( 103.1528011352953342, 3.152801135295383084, 2.312500001365592084 ) ) ;
#21413=CARTESIAN_POINT ( 'NONE',  ( 101.8468681455906903, 4.458734125000016313, 1.125000001365592750 ) ) ;
#21415=CARTESIAN_POINT ( 'NONE',  ( 101.8468681455906903, 4.458734125000016313, 5.125000001365592972 ) ) ;
#21417=CARTESIAN_POINT ( 'NONE',  ( 96.84719886470459471, 3.152801135295383084, 2.562500001365592084 ) ) ;
#21425=CARTESIAN_POINT ( 'NONE',  ( 103.5355339059327093, 3.535533905932755072, 5.625000000000000000 ) ) ;
#21446=CARTESIAN_POINT ( 'NONE',  ( 103.1528011352953342, 3.152801135295383084, 14.31250000136559208 ) ) ;
#21458=CARTESIAN_POINT ( 'NONE',  ( 103.5355339059327093, 3.535533905932755072, 1.750000002731184834 ) ) ;
#21474=CARTESIAN_POINT ( 'NONE',  ( 98.15313185440925281, -4.458734124999987891, 7.625000001365592084 ) ) ;
#21476=CARTESIAN_POINT ( 'NONE',  ( 99.99999999999995737, 4.458734125000016313, 13.18750000136559208 ) ) ;
#21495=CARTESIAN_POINT ( 'NONE',  ( 103.5355339059327093, -3.535533905932726206, 3.374999999999999556 ) ) ;
#21504=CARTESIAN_POINT ( 'NONE',  ( 96.46446609406721961, 3.535533905932755072, 5.000000002731185944 ) ) ;
#21509=ADVANCED_FACE ( 'NONE', ( #25425 ), #8029, .F. ) ;
#21512=CARTESIAN_POINT ( 'NONE',  ( 104.4587341249999781, 1.846868145590750299, 2.250000001365591640 ) ) ;
#21515=CARTESIAN_POINT ( 'NONE',  ( 101.8468681455907046, -4.458734124999987891, 5.750000001365591196 ) ) ;
#21532=CARTESIAN_POINT ( 'NONE',  ( 104.4587341249999639, 1.442382525525748735E-14, 1.187500001365592750 ) ) ;
#21540=EDGE_CURVE ( 'NONE', #27745, #7831, #14295, .T. ) ;
#21549=CARTESIAN_POINT ( 'NONE',  ( 99.99999999999995737, 4.458734125000016313, 14.43750000136559208 ) ) ;
#21551=CARTESIAN_POINT ( 'NONE',  ( 98.15313185440925281, 4.458734125000016313, 4.250000001365592084 ) ) ;
#21558=EDGE_CURVE ( 'NONE', #8379, #11095, #15553, .T. ) ;
#21563=CARTESIAN_POINT ( 'NONE',  ( 104.9999999999999716, 1.449011120738813565E-14, 5.500000000000000000 ) ) ;
#21571=ORIENTED_EDGE ( 'NONE', *, *, #24954, .F. ) ;
#21582=SURFACE_SIDE_STYLE ('',( #3916 ) ) ;
#21583=CARTESIAN_POINT ( 'NONE',  ( 99.99999999999995737, -4.458734124999988779, 10.93750000136559208 ) ) ;
#21596=CARTESIAN_POINT ( 'NONE',  ( 95.54126587499996504, 1.387778780781445676E-14, 14.43750000136559208 ) ) ;
#21600=CARTESIAN_POINT ( 'NONE',  ( 104.9999999999999716, 1.449011120738813565E-14, 13.62500000273118417 ) ) ;
#21607=CARTESIAN_POINT ( 'NONE',  ( 97.92893218813451028, 5.000000000000018652, 10.81250000000000000 ) ) ;
#21612=CARTESIAN_POINT ( 'NONE',  ( 95.54126587499995082, -1.846868145590724986, 8.500000001365592084 ) ) ;
#21616=CARTESIAN_POINT ( 'NONE',  ( 103.1528011352953342, 3.152801135295383084, 10.06250000136559208 ) ) ;
#21623=CARTESIAN_POINT ( 'NONE',  ( 94.99999999999994316, 2.071067811865481278, 11.93750000000000000 ) ) ;
#21624=( BOUNDED_CURVE ( )  B_SPLINE_CURVE ( 2, ( #24887, #14176, #24744, #13746, #7484, #26895, #20328, #5366, #9765 ),
 .UNSPECIFIED., .F., .T. ) 
 B_SPLINE_CURVE_WITH_KNOTS ( ( 3, 2, 2, 2, 3 ),
 ( 0.6785714285714284921, 0.6874999999999998890, 0.6964285714285712858, 0.7053571428571427937, 0.7142857142857141906 ),
 .UNSPECIFIED. ) 
 CURVE ( )  GEOMETRIC_REPRESENTATION_ITEM ( )  RATIONAL_B_SPLINE_CURVE ( ( 1.000000000000000888, 0.9238795325112857393, 1.000000000000000000, 0.9238795325112867385, 1.000000000000000000, 0.9238795325112867385, 1.000000000000000000, 0.9238795325112877377, 0.9999999999999990008 ) ) 
 REPRESENTATION_ITEM ( '' )  );
#21625=ORIENTED_EDGE ( 'NONE', *, *, #27599, .T. ) ;
#21641=CARTESIAN_POINT ( 'NONE',  ( 103.5355339059327093, -3.535533905932726206, 4.374999999999999112 ) ) ;
#21649=CARTESIAN_POINT ( 'NONE',  ( 103.5355339059327093, 3.535533905932755072, 4.750000002731185944 ) ) ;
#21651=CARTESIAN_POINT ( 'NONE',  ( 94.99999999999995737, -2.071067811865466624, 12.18750000273118950 ) ) ;
#21658=CARTESIAN_POINT ( 'NONE',  ( 96.84719886470459471, -3.152801135295355994, 0.5625000013655921949 ) ) ;
#21673=ADVANCED_FACE ( 'NONE', ( #4597 ), #11793, .F. ) ;
#21675=CARTESIAN_POINT ( 'NONE',  ( 95.54126587499995082, -1.846868145590724986, 4.750000001365592084 ) ) ;
#21692=CARTESIAN_POINT ( 'NONE',  ( 95.54126587499995082, 1.846868145590750077, 13.62500000136559386 ) ) ;
#21694=CARTESIAN_POINT ( 'NONE',  ( 104.4587341249999781, 1.846868145590750521, 13.00000000136559386 ) ) ;
#21697=FACE_OUTER_BOUND ( 'NONE', #6959, .T. ) ;
#21710=CARTESIAN_POINT ( 'NONE',  ( 94.99999999999995737, 1.387778780781445676E-14, 7.125000002731185056 ) ) ;
#21713=CARTESIAN_POINT ( 'NONE',  ( 95.54126587499995082, -1.846868145590724986, 13.75000000136559208 ) ) ;
#21730=CARTESIAN_POINT ( 'NONE',  ( 98.15313185440923860, -4.458734124999987891, 9.875000001365593860 ) ) ;
#21743=CARTESIAN_POINT ( 'NONE',  ( 96.84719886470459471, 3.152801135295383084, 14.31250000136559208 ) ) ;
#21751=CARTESIAN_POINT ( 'NONE',  ( 94.99999999999995737, 2.071067811865491493, 10.06250000273118417 ) ) ;
#21759=CARTESIAN_POINT ( 'NONE',  ( 99.99999999999995737, -4.458734124999988779, 10.68750000136559208 ) ) ;
#21762=CARTESIAN_POINT ( 'NONE',  ( 96.84719886470459471, -3.152801135295355994, 11.56250000136559208 ) ) ;
#21774=ORIENTED_EDGE ( 'NONE', *, *, #9831, .T. ) ;
#21775=FACE_OUTER_BOUND ( 'NONE', #8868, .T. ) ;
#21783=AXIS2_PLACEMENT_3D ( 'NONE', #26039, #17054, #107 ) ;
#21784=CARTESIAN_POINT ( 'NONE',  ( 94.99999999999995737, -2.071067811865466624, 7.062499999999999112 ) ) ;
#21790=CARTESIAN_POINT ( 'NONE',  ( 94.99999999999995737, 1.387778780781445676E-14, 9.125000002731184168 ) ) ;
#21793=( BOUNDED_CURVE ( )  B_SPLINE_CURVE ( 2, ( #7451, #7601, #24421, #22861, #9174, #15718, #9592, #17867, #18295 ),
 .UNSPECIFIED., .F., .T. ) 
 B_SPLINE_CURVE_WITH_KNOTS ( ( 3, 2, 2, 2, 3 ),
 ( 0.8928571428571427937, 0.9017857142857141906, 0.9107142857142855874, 0.9196428571428569843, 0.9285714285714284921 ),
 .UNSPECIFIED. ) 
 CURVE ( )  GEOMETRIC_REPRESENTATION_ITEM ( )  RATIONAL_B_SPLINE_CURVE ( ( 1.000000000000000888, 0.9238795325112857393, 1.000000000000000000, 0.9238795325112867385, 1.000000000000000000, 0.9238795325112867385, 1.000000000000000000, 0.9238795325112877377, 0.9999999999999990008 ) ) 
 REPRESENTATION_ITEM ( '' )  );
#21802=CARTESIAN_POINT ( 'NONE',  ( 98.15313185440923860, 4.458734125000016313, 2.250000001365592084 ) ) ;
#21809=ORIENTED_EDGE ( 'NONE', *, *, #9004, .F. ) ;
#21821=CARTESIAN_POINT ( 'NONE',  ( 103.1528011352953342, -3.152801135295355106, 3.062500001365592528 ) ) ;
#21828=DIRECTION ( 'NONE',  ( -0.000000000000000000, -0.000000000000000000, -1.000000000000000000 ) ) ;
#21836=CARTESIAN_POINT ( 'NONE',  ( 99.99999999999995737, -4.458734124999988779, 11.93750000136559208 ) ) ;
#21838=CARTESIAN_POINT ( 'NONE',  ( 104.4587341249999781, 1.846868145590750521, 14.00000000136559208 ) ) ;
#21869=CARTESIAN_POINT ( 'NONE',  ( 101.8468681455907046, 4.458734125000016313, 11.37500000136559386 ) ) ;
#21886=CARTESIAN_POINT ( 'NONE',  ( 102.0710678118654329, 5.000000000000018652, 0.8125000027311859441 ) ) ;
#21892=DIRECTION ( 'NONE',  ( 0.000000000000000000, -1.000000000000000000, 0.000000000000000000 ) ) ;
#21901=CARTESIAN_POINT ( 'NONE',  ( 102.0710678118654329, -4.999999999999989342, 10.31249999999999822 ) ) ;
#21903=CARTESIAN_POINT ( 'NONE',  ( 104.4587341249999781, -1.846868145590721655, 8.875000001365593860 ) ) ;
#21906=CARTESIAN_POINT ( 'NONE',  ( 104.4587341249999781, -1.846868145590721655, 13.87500000136559208 ) ) ;
#21927=CARTESIAN_POINT ( 'NONE',  ( 102.0710678118654329, -4.999999999999989342, 5.312499999999999112 ) ) ;
#21934=CARTESIAN_POINT ( 'NONE',  ( 97.92893218813451028, 5.000000000000018652, 6.812499999999999112 ) ) ;
#21942=CARTESIAN_POINT ( 'NONE',  ( 96.84719886470459471, -3.152801135295355994, 0.8125000013655924169 ) ) ;
#21944=CARTESIAN_POINT ( 'NONE',  ( 104.4587341249999639, 1.442382525525748735E-14, 2.937500001365592528 ) ) ;
#21958=CARTESIAN_POINT ( 'NONE',  ( 95.54126587499995082, -1.846868145590724986, 1.750000001365591862 ) ) ;
#21963=( BOUNDED_CURVE ( )  B_SPLINE_CURVE ( 2, ( #20560, #13548, #11548, #18272, #2746, #11408, #7138, #15833, #7283 ),
 .UNSPECIFIED., .F., .T. ) 
 B_SPLINE_CURVE_WITH_KNOTS ( ( 3, 2, 2, 2, 3 ),
 ( 0.9642857142857141906, 0.9732142857142855874, 0.9821428571428569843, 0.9910714285714286031, 1.000000000000000000 ),
 .UNSPECIFIED. ) 
 CURVE ( )  GEOMETRIC_REPRESENTATION_ITEM ( )  RATIONAL_B_SPLINE_CURVE ( ( 1.000000000000000888, 0.9238795325112857393, 1.000000000000000000, 0.9238795325112867385, 1.000000000000000000, 0.9238795325112867385, 1.000000000000000000, 0.9238795325112867385, 1.000000000000000000 ) ) 
 REPRESENTATION_ITEM ( '' )  );
#21972=CARTESIAN_POINT ( 'NONE',  ( 104.4587341249999781, 1.846868145590750299, 11.25000000136559208 ) ) ;
#21974=CARTESIAN_POINT ( 'NONE',  ( 104.4587341249999781, -1.846868145590721655, 13.87500000136559208 ) ) ;
#21977=DIRECTION ( 'NONE',  ( -1.000000000000000000, 0.000000000000000000, 0.000000000000000000 ) ) ;
#21986=CARTESIAN_POINT ( 'NONE',  ( 96.46446609406721961, -3.535533905932727539, 7.250000002731185056 ) ) ;
#21988=CARTESIAN_POINT ( 'NONE',  ( 98.15313185440925281, -4.458734124999987891, 13.87500000136559208 ) ) ;
#21996=LINE ( 'NONE', #24408, #8898 ) ;
#22002=ORIENTED_EDGE ( 'NONE', *, *, #4310, .T. ) ;
#22005=CARTESIAN_POINT ( 'NONE',  ( 104.4587341249999781, 1.846868145590750521, 9.250000001365592084 ) ) ;
#22029=EDGE_CURVE ( 'NONE', #27745, #26423, #21295, .T. ) ;
#22033=CARTESIAN_POINT ( 'NONE',  ( 97.92893218813451028, -4.999999999999989342, 10.18749999999999822 ) ) ;
#22034=VERTEX_POINT ( 'NONE', #17028 ) ;
#22035=CARTESIAN_POINT ( 'NONE',  ( 104.4587341249999781, 1.846868145590750299, 8.000000001365592084 ) ) ;
#22038=CARTESIAN_POINT ( 'NONE',  ( 103.1528011352953342, 3.152801135295383084, 12.06250000136559208 ) ) ;
#22048=( BOUNDED_CURVE ( )  B_SPLINE_CURVE ( 2, ( #20751, #25440, #18874, #1644, #5922, #23029, #3920, #12578, #8186 ),
 .UNSPECIFIED., .F., .F. ) 
 B_SPLINE_CURVE_WITH_KNOTS ( ( 3, 2, 2, 2, 3 ),
 ( 0.07142857142857149400, 0.08035714285714290472, 0.08928571428571430157, 0.09821428571428571230, 0.1071428571428571092 ),
 .UNSPECIFIED. ) 
 CURVE ( )  GEOMETRIC_REPRESENTATION_ITEM ( )  RATIONAL_B_SPLINE_CURVE ( ( 0.9999999999999994449, 0.9238795325112872936, 1.000000000000000000, 0.9238795325112867385, 1.000000000000000000, 0.9238795325112867385, 1.000000000000000000, 0.9238795325112869605, 0.9999999999999997780 ) ) 
 REPRESENTATION_ITEM ( '' )  );
#22050=CARTESIAN_POINT ( 'NONE',  ( 99.99999999999995737, 1.387778780781445676E-14, 15.00000000000000000 ) ) ;
#22058=CARTESIAN_POINT ( 'NONE',  ( 103.5355339059327093, 3.535533905932755072, 7.750000002731185056 ) ) ;
#22065=CARTESIAN_POINT ( 'NONE',  ( 94.99999999999995737, -2.071067811865466624, 3.062499999999999112 ) ) ;
#22083=CARTESIAN_POINT ( 'NONE',  ( 104.4587341249999639, 1.442382525525748735E-14, 3.937500001365591640 ) ) ;
#22100=CARTESIAN_POINT ( 'NONE',  ( 99.99999999999995737, -4.999999999999990230, 14.24999999999999822 ) ) ;
#22101=EDGE_CURVE ( 'NONE', #6975, #26723, #10470, .T. ) ;
#22103=LINE ( 'NONE', #27200, #26161 ) ;
#22113=CARTESIAN_POINT ( 'NONE',  ( 95.54126587499995082, 1.846868145590750077, 10.62500000136559208 ) ) ;
#22115=CARTESIAN_POINT ( 'NONE',  ( 95.54126587499996504, 1.846868145590750077, 14.37500000136559386 ) ) ;
#22124=CARTESIAN_POINT ( 'NONE',  ( 94.99999999999995737, 1.387778780781445676E-14, 9.999999999999998224 ) ) ;
#22130=CARTESIAN_POINT ( 'NONE',  ( 98.15313185440925281, 4.458734125000016313, 11.50000000136559208 ) ) ;
#22146=CARTESIAN_POINT ( 'NONE',  ( 101.8468681455907046, -4.458734124999987891, 13.00000000136559386 ) ) ;
#22165=ORIENTED_EDGE ( 'NONE', *, *, #2181, .T. ) ;
#22172=DIRECTION ( 'NONE',  ( -1.000000000000000000, 0.000000000000000000, 0.000000000000000000 ) ) ;
#22176=CARTESIAN_POINT ( 'NONE',  ( 101.8468681455906903, -4.458734124999987891, 6.750000001365592972 ) ) ;
#22179=CARTESIAN_POINT ( 'NONE',  ( 99.99999999999995737, -4.458734124999988779, 7.687500001365592084 ) ) ;
#22180=CARTESIAN_POINT ( 'NONE',  ( 104.9999999999999716, 1.449011120738813565E-14, 8.499999999999998224 ) ) ;
#22197=CARTESIAN_POINT ( 'NONE',  ( 94.99999999999995737, 2.071067811865491048, 9.062500002731184168 ) ) ;
#22203=CARTESIAN_POINT ( 'NONE',  ( 96.46446609406721961, 3.535533905932755072, 2.874999999999999112 ) ) ;
#22211=CYLINDRICAL_SURFACE ( 'NONE', #17691, 5.000000000000004441 ) ;
#22223=CARTESIAN_POINT ( 'NONE',  ( 98.15313185440923860, -4.458734124999987891, 3.625000001365591196 ) ) ;
#22240=ORIENTED_EDGE ( 'NONE', *, *, #1482, .F. ) ;
#22242=CARTESIAN_POINT ( 'NONE',  ( 104.9999999999999574, -2.071067811865462627, 12.43750000000000000 ) ) ;
#22244=VERTEX_POINT ( 'NONE', #11847 ) ;
#22247=VERTEX_POINT ( 'NONE', #20569 ) ;
#22257=CARTESIAN_POINT ( 'NONE',  ( 98.15313185440925281, -4.458734124999987891, 11.87500000136559031 ) ) ;
#22258=LINE ( 'NONE', #8995, #23991 ) ;
#22259=CARTESIAN_POINT ( 'NONE',  ( 104.4587341249999781, -1.846868145590721655, 0.8750000013655926390 ) ) ;
#22269=( BOUNDED_CURVE ( )  B_SPLINE_CURVE ( 2, ( #23188, #23461, #27742, #19031, #12326, #10469, #5135, #25591, #11664 ),
 .UNSPECIFIED., .F., .T. ) 
 B_SPLINE_CURVE_WITH_KNOTS ( ( 3, 2, 2, 2, 3 ),
 ( 0.3214285714285713969, 0.3303571428571427937, 0.3392857142857143016, 0.3482142857142856984, 0.3571428571428572063 ),
 .UNSPECIFIED. ) 
 CURVE ( )  GEOMETRIC_REPRESENTATION_ITEM ( )  RATIONAL_B_SPLINE_CURVE ( ( 1.000000000000000444, 0.9238795325112862944, 1.000000000000000000, 0.9238795325112867385, 1.000000000000000000, 0.9238795325112867385, 1.000000000000000000, 0.9238795325112862944, 1.000000000000000444 ) ) 
 REPRESENTATION_ITEM ( '' )  );
#22276=CARTESIAN_POINT ( 'NONE',  ( 104.4587341249999781, -1.846868145590721655, 9.125000001365592084 ) ) ;
#22291=CARTESIAN_POINT ( 'NONE',  ( 95.54126587499996504, 1.846868145590750077, 6.625000001365592084 ) ) ;
#22304=ORIENTED_EDGE ( 'NONE', *, *, #11675, .F. ) ;
#22310=CARTESIAN_POINT ( 'NONE',  ( 94.99999999999995737, -2.071067811865466624, 13.06250000000000000 ) ) ;
#22313=DIRECTION ( 'NONE',  ( -0.000000000000000000, -0.000000000000000000, -1.000000000000000000 ) ) ;
#22321=CARTESIAN_POINT ( 'NONE',  ( 95.54126587499995082, -1.846868145590724986, 5.500000001365591196 ) ) ;
#22324=CARTESIAN_POINT ( 'NONE',  ( 95.54126587499995082, -1.846868145590724986, 6.500000001365592084 ) ) ;
#22341=CARTESIAN_POINT ( 'NONE',  ( 102.0710678118654329, 5.000000000000018652, 10.81250000273118417 ) ) ;
#22380=CARTESIAN_POINT ( 'NONE',  ( 102.0710678118654329, -4.999999999999989342, 13.31250000000000000 ) ) ;
#22387=DIRECTION ( 'NONE',  ( -1.000000000000000000, 0.000000000000000000, 0.000000000000000000 ) ) ;
#22396=CARTESIAN_POINT ( 'NONE',  ( 101.8468681455906903, 4.458734125000016313, 9.375000001365592084 ) ) ;
#22398=CARTESIAN_POINT ( 'NONE',  ( 104.4587341249999781, 1.846868145590750521, 10.00000000136559208 ) ) ;
#22401=CARTESIAN_POINT ( 'NONE',  ( 102.0710678118654329, 5.000000000000018652, 3.687500000000000444 ) ) ;
#22412=CARTESIAN_POINT ( 'NONE',  ( 96.84719886470459471, 3.152801135295383084, 10.56250000136559208 ) ) ;
#22429=( BOUNDED_CURVE ( )  B_SPLINE_CURVE ( 2, ( #3991, #3847, #12654, #16939, #21236, #21379, #1858, #1718, #10380 ),
 .UNSPECIFIED., .F., .F. ) 
 B_SPLINE_CURVE_WITH_KNOTS ( ( 3, 2, 2, 2, 3 ),
 ( 0.3928571428571428492, 0.4017857142857143016, 0.4107142857142856984, 0.4196428571428571508, 0.4285714285714285476 ),
 .UNSPECIFIED. ) 
 CURVE ( )  GEOMETRIC_REPRESENTATION_ITEM ( )  RATIONAL_B_SPLINE_CURVE ( ( 1.000000000000000000, 0.9238795325112867385, 1.000000000000000000, 0.9238795325112867385, 1.000000000000000000, 0.9238795325112867385, 1.000000000000000000, 0.9238795325112867385, 1.000000000000000000 ) ) 
 REPRESENTATION_ITEM ( '' )  );
#22432=CARTESIAN_POINT ( 'NONE',  ( 96.84719886470459471, 3.152801135295383084, 7.562500001365592084 ) ) ;
#22436=CARTESIAN_POINT ( 'NONE',  ( 97.92893218813451028, -4.999999999999989342, 14.18749999999999645 ) ) ;
#22438=EDGE_LOOP ( 'NONE', ( #4193, #10861, #15976, #24429 ) ) ;
#22444=CARTESIAN_POINT ( 'NONE',  ( 99.99999999999995737, 1.387778780781445676E-14, 0.000000000000000000 ) ) ;
#22448=CARTESIAN_POINT ( 'NONE',  ( 96.46446609406721961, -3.535533905932727539, 0.2500000027311852779 ) ) ;
#22458=CARTESIAN_POINT ( 'NONE',  ( 99.99999999999995737, 1.387778780781445676E-14, 34.79898987322334136 ) ) ;
#22462=CARTESIAN_POINT ( 'NONE',  ( 99.99999999999995737, 4.458734125000016313, 3.187500001365592972 ) ) ;
#22464=CARTESIAN_POINT ( 'NONE',  ( 94.99999999999995737, 1.387778780781445676E-14, 13.12500000273118417 ) ) ;
#22465=CARTESIAN_POINT ( 'NONE',  ( 103.1528011352953342, -3.152801135295355106, 8.812500001365592084 ) ) ;
#22468=DIRECTION ( 'NONE',  ( -1.000000000000000000, 0.000000000000000000, 0.000000000000000000 ) ) ;
#22478=EDGE_LOOP ( 'NONE', ( #21809, #22165, #15997, #3661 ) ) ;
#22482=CARTESIAN_POINT ( 'NONE',  ( 96.46446609406721961, 3.535533905932755072, 11.00000000273118594 ) ) ;
#22487=CARTESIAN_POINT ( 'NONE',  ( 103.5355339059327093, -3.535533905932726206, 2.374999999999998668 ) ) ;
#22526=CARTESIAN_POINT ( 'NONE',  ( 103.5355339059327093, 3.535533905932755072, 12.62499999999999822 ) ) ;
#22539=CARTESIAN_POINT ( 'NONE',  ( 101.8468681455906903, 4.458734125000016313, 5.375000001365592972 ) ) ;
#22542=CARTESIAN_POINT ( 'NONE',  ( 101.8468681455907046, 4.458734125000016313, 9.125000001365592084 ) ) ;
#22545=CARTESIAN_POINT ( 'NONE',  ( 94.99999999999995737, 1.387778780781445676E-14, 4.000000000000000000 ) ) ;
#22558=CARTESIAN_POINT ( 'NONE',  ( 104.4587341249999781, -1.846868145590721655, 11.12500000136559386 ) ) ;
#22564=EDGE_CURVE ( 'NONE', #22244, #4790, #24039, .T. ) ;
#22575=CARTESIAN_POINT ( 'NONE',  ( 96.84719886470459471, 3.152801135295383084, 5.562500001365592972 ) ) ;
#22597=CARTESIAN_POINT ( 'NONE',  ( 96.46446609406721961, -3.535533905932727539, 13.12500000000000000 ) ) ;
#22598=( NAMED_UNIT ( * ) SI_UNIT ( $, .STERADIAN. ) SOLID_ANGLE_UNIT ( ) );
#22602=( BOUNDED_CURVE ( )  B_SPLINE_CURVE ( 2, ( #4805, #8510, #10770, #19905, #1965, #4237, #6784, #19339, #15327 ),
 .UNSPECIFIED., .F., .F. ) 
 B_SPLINE_CURVE_WITH_KNOTS ( ( 3, 2, 2, 2, 3 ),
 ( 0.1785714285714286031, 0.1875000000000000000, 0.1964285714285713969, 0.2053571428571428215, 0.2142857142857142183 ),
 .UNSPECIFIED. ) 
 CURVE ( )  GEOMETRIC_REPRESENTATION_ITEM ( )  RATIONAL_B_SPLINE_CURVE ( ( 0.9999999999999997780, 0.9238795325112869605, 1.000000000000000000, 0.9238795325112867385, 1.000000000000000000, 0.9238795325112867385, 1.000000000000000000, 0.9238795325112871826, 0.9999999999999995559 ) ) 
 REPRESENTATION_ITEM ( '' )  );
#22608=CARTESIAN_POINT ( 'NONE',  ( 98.15313185440925281, 4.458734125000016313, 3.250000001365592528 ) ) ;
#22611=CARTESIAN_POINT ( 'NONE',  ( 103.1528011352953342, 3.152801135295383084, 6.062500001365592084 ) ) ;
#22628=CARTESIAN_POINT ( 'NONE',  ( 104.9999999999999574, 2.071067811865491937, 10.68750000273118417 ) ) ;
#22672=CARTESIAN_POINT ( 'NONE',  ( 97.92893218813451028, -4.999999999999989342, 12.18750000000000000 ) ) ;
#22685=CARTESIAN_POINT ( 'NONE',  ( 104.4587341249999781, 1.846868145590750299, 8.250000001365592084 ) ) ;
#22687=CARTESIAN_POINT ( 'NONE',  ( 99.99999999999995737, -4.458734124999988779, 11.68750000136559208 ) ) ;
#22694=VERTEX_POINT ( 'NONE', #19078 ) ;
#22702=CARTESIAN_POINT ( 'NONE',  ( 99.99999999999995737, -4.458734124999988779, 11.93750000136559208 ) ) ;
#22718=CARTESIAN_POINT ( 'NONE',  ( 101.8468681455907046, -4.458734124999987891, 7.000000001365592972 ) ) ;
#22741=FACE_OUTER_BOUND ( 'NONE', #4735, .T. ) ;
#22750=CARTESIAN_POINT ( 'NONE',  ( 95.54126587499995082, -1.846868145590724986, 4.500000001365592084 ) ) ;
#22753=CARTESIAN_POINT ( 'NONE',  ( 104.4587341249999639, 1.442382525525748735E-14, 8.937500001365592084 ) ) ;
#22769=CARTESIAN_POINT ( 'NONE',  ( 94.99999999999995737, 2.071067811865491048, 6.062500002731184168 ) ) ;
#22772=( BOUNDED_CURVE ( )  B_SPLINE_CURVE ( 2, ( #4058, #10032, #8321, #12720, #16600, #6324, #21446, #7905, #10451, #1924, #19157, #20887, #17006, #23439, #25292, #12303, #5780, #10303, #14448, #3778, #21026, #27583, #8042, #16739, #5920, #14586, #15571, #22146, #6463, #345, #6884, #15138, #4760, #9032, #13134, #24279, #13420, #11288, #8742, #2627, #26567, #10865, #17434, #24417, #20009, #489, #26133, #15426, #12854, #9171, #26426, #17863, #23856, #21869, #7020, #4334, #2347, #201, #17291, #15715, #21583, #11003, #2203, #19715, #24139, #12990, #2059, #10729, #8884, #19577, #19437, #4616, #28136, #8603, #61, #6599, #25993, #21730, #26280, #13275, #4478, #17574, #15282, #24001, #11142, #6741, #17724, #22005, #2481, #19858, #2900, #9305, #3042, #24565, #13850, #11431, #24707, #7736, #20151, #13711, #22857, #16426, #15856, #5046, #7306, #16286, #20719, #5187, #630, #18577, #14137, #9870, #9446, #16142, #22432, #9589, #24850, #11570, #13992, #4906, #5328, #11712, #2767, #22718, #13568, #7160, #20437, #24987, #20287, #22291, #18003, #918, #18293, #773, #18146, #5468, #11995, #15993, #3324, #26999, #3186, #26860, #1202, #27280, #7446, #26711, #22575, #11856, #20578, #1061, #9731, #18436, #27144, #7596, #16710, #18982, #5750, #27969, #5610, #1895, #4027, #20856, #23549, #1754, #3464, #16847, #10420, #8154, #8426, #14689, #25545, #1475, #23275, #22994, #23408, #25122, #27411, #3748, #8287, #12269, #14276, #14560, #3610, #6025, #12409, #10561, #21129, #10132, #12692, #14418, #16979, #12129, #7874, #14826, #21417, #1615, #19270, #23133, #1338, #10002, #10273, #25677, #16568, #6159, #27692, #3883, #19126, #12544, #18709, #25259, #21270, #27833, #20995, #18844, #27553, #8010, #25408, #5890, #172, #456, #6706, #2170, #19685, #17115, #13390 ),
 .UNSPECIFIED., .F., .T. ) 
 B_SPLINE_CURVE_WITH_KNOTS ( ( 3, 2, 2, 2, 2, 2, 2, 2, 2, 2, 2, 2, 2, 2, 2, 2, 2, 2, 2, 2, 2, 2, 2, 2, 2, 2, 2, 2, 2, 2, 2, 2, 2, 2, 2, 2, 2, 2, 2, 2, 2, 2, 2, 2, 2, 2, 2, 2, 2, 2, 2, 2, 2, 2, 2, 2, 2, 2, 2, 2, 2, 2, 2, 2, 2, 2, 2, 2, 2, 2, 2, 2, 2, 2, 2, 2, 2, 2, 2, 2, 2, 2, 2, 2, 2, 2, 2, 2, 2, 2, 2, 2, 2, 2, 2, 2, 2, 2, 2, 2, 2, 2, 2, 2, 2, 2, 2, 2, 2, 2, 2, 2, 3 ),
 ( 0.000000000000000000, 0.008928571428571428076, 0.01785714285714285615, 0.02678571428571428423, 0.03571428571428571230, 0.04464285714285714385, 0.05357142857142856845, 0.06250000000000000000, 0.07142857142857142461, 0.08035714285714286309, 0.08928571428571428770, 0.09821428571428571230, 0.1071428571428571369, 0.1160714285714285754, 0.1250000000000000000, 0.1339285714285714246, 0.1428571428571428492, 0.1517857142857142738, 0.1607142857142857262, 0.1696428571428571508, 0.1785714285714285754, 0.1875000000000000000, 0.1964285714285714246, 0.2053571428571428492, 0.2142857142857142738, 0.2232142857142857262, 0.2321428571428571508, 0.2410714285714285754, 0.2500000000000000000, 0.2589285714285714524, 0.2678571428571428492, 0.2767857142857143016, 0.2857142857142856984, 0.2946428571428571508, 0.3035714285714285476, 0.3125000000000000000, 0.3214285714285714524, 0.3303571428571428492, 0.3392857142857143016, 0.3482142857142856984, 0.3571428571428571508, 0.3660714285714285476, 0.3750000000000000000, 0.3839285714285714524, 0.3928571428571428492, 0.4017857142857143016, 0.4107142857142856984, 0.4196428571428571508, 0.4285714285714285476, 0.4375000000000000000, 0.4464285714285714524, 0.4553571428571428492, 0.4642857142857143016, 0.4732142857142856984, 0.4821428571428571508, 0.4910714285714285476, 0.5000000000000000000, 0.5089285714285713969, 0.5178571428571429047, 0.5267857142857143016, 0.5357142857142856984, 0.5446428571428570953, 0.5535714285714286031, 0.5625000000000000000, 0.5714285714285713969, 0.5803571428571429047, 0.5892857142857143016, 0.5982142857142856984, 0.6071428571428570953, 0.6160714285714286031, 0.6250000000000000000, 0.6339285714285713969, 0.6428571428571429047, 0.6517857142857143016, 0.6607142857142856984, 0.6696428571428570953, 0.6785714285714286031, 0.6875000000000000000, 0.6964285714285713969, 0.7053571428571429047, 0.7142857142857143016, 0.7232142857142856984, 0.7321428571428570953, 0.7410714285714286031, 0.7500000000000000000, 0.7589285714285713969, 0.7678571428571429047, 0.7767857142857143016, 0.7857142857142856984, 0.7946428571428570953, 0.8035714285714286031, 0.8125000000000000000, 0.8214285714285713969, 0.8303571428571429047, 0.8392857142857143016, 0.8482142857142856984, 0.8571428571428570953, 0.8660714285714286031, 0.8750000000000000000, 0.8839285714285713969, 0.8928571428571429047, 0.9017857142857143016, 0.9107142857142856984, 0.9196428571428570953, 0.9285714285714286031, 0.9375000000000000000, 0.9464285714285713969, 0.9553571428571429047, 0.9642857142857143016, 0.9732142857142856984, 0.9821428571428570953, 0.9910714285714286031, 1.000000000000000000 ),
 .UNSPECIFIED. ) 
 CURVE ( )  GEOMETRIC_REPRESENTATION_ITEM ( )  RATIONAL_B_SPLINE_CURVE ( ( 1.000000000000000000, 0.9238795325112867385, 1.000000000000000000, 0.9238795325112867385, 1.000000000000000000, 0.9238795325112867385, 1.000000000000000000, 0.9238795325112867385, 1.000000000000000000, 0.9238795325112867385, 1.000000000000000000, 0.9238795325112867385, 1.000000000000000000, 0.9238795325112867385, 1.000000000000000000, 0.9238795325112867385, 1.000000000000000000, 0.9238795325112867385, 1.000000000000000000, 0.9238795325112867385, 1.000000000000000000, 0.9238795325112867385, 1.000000000000000000, 0.9238795325112867385, 1.000000000000000000, 0.9238795325112867385, 1.000000000000000000, 0.9238795325112867385, 1.000000000000000000, 0.9238795325112867385, 1.000000000000000000, 0.9238795325112867385, 1.000000000000000000, 0.9238795325112867385, 1.000000000000000000, 0.9238795325112867385, 1.000000000000000000, 0.9238795325112867385, 1.000000000000000000, 0.9238795325112867385, 1.000000000000000000, 0.9238795325112867385, 1.000000000000000000, 0.9238795325112867385, 1.000000000000000000, 0.9238795325112867385, 1.000000000000000000, 0.9238795325112867385, 1.000000000000000000, 0.9238795325112867385, 1.000000000000000000, 0.9238795325112867385, 1.000000000000000000, 0.9238795325112867385, 1.000000000000000000, 0.9238795325112867385, 1.000000000000000000, 0.9238795325112867385, 1.000000000000000000, 0.9238795325112867385, 1.000000000000000000, 0.9238795325112867385, 1.000000000000000000, 0.9238795325112867385, 1.000000000000000000, 0.9238795325112867385, 1.000000000000000000, 0.9238795325112867385, 1.000000000000000000, 0.9238795325112867385, 1.000000000000000000, 0.9238795325112867385, 1.000000000000000000, 0.9238795325112867385, 1.000000000000000000, 0.9238795325112867385, 1.000000000000000000, 0.9238795325112867385, 1.000000000000000000, 0.9238795325112867385, 1.000000000000000000, 0.9238795325112867385, 1.000000000000000000, 0.9238795325112867385, 1.000000000000000000, 0.9238795325112867385, 1.000000000000000000, 0.9238795325112867385, 1.000000000000000000, 0.9238795325112867385, 1.000000000000000000, 0.9238795325112867385, 1.000000000000000000, 0.9238795325112867385, 1.000000000000000000, 0.9238795325112867385, 1.000000000000000000, 0.9238795325112867385, 1.000000000000000000, 0.9238795325112867385, 1.000000000000000000, 0.9238795325112867385, 1.000000000000000000, 0.9238795325112867385, 1.000000000000000000, 0.9238795325112867385, 1.000000000000000000, 0.9238795325112867385, 1.000000000000000000, 0.9238795325112867385, 1.000000000000000000, 0.9238795325112867385, 1.000000000000000000, 0.9238795325112867385, 1.000000000000000000, 0.9238795325112867385, 1.000000000000000000, 0.9238795325112867385, 1.000000000000000000, 0.9238795325112867385, 1.000000000000000000, 0.9238795325112867385, 1.000000000000000000, 0.9238795325112867385, 1.000000000000000000, 0.9238795325112867385, 1.000000000000000000, 0.9238795325112867385, 1.000000000000000000, 0.9238795325112867385, 1.000000000000000000, 0.9238795325112867385, 1.000000000000000000, 0.9238795325112867385, 1.000000000000000000, 0.9238795325112867385, 1.000000000000000000, 0.9238795325112867385, 1.000000000000000000, 0.9238795325112867385, 1.000000000000000000, 0.9238795325112867385, 1.000000000000000000, 0.9238795325112867385, 1.000000000000000000, 0.9238795325112867385, 1.000000000000000000, 0.9238795325112867385, 1.000000000000000000, 0.9238795325112867385, 1.000000000000000000, 0.9238795325112867385, 1.000000000000000000, 0.9238795325112867385, 1.000000000000000000, 0.9238795325112867385, 1.000000000000000000, 0.9238795325112867385, 1.000000000000000000, 0.9238795325112867385, 1.000000000000000000, 0.9238795325112867385, 1.000000000000000000, 0.9238795325112867385, 1.000000000000000000, 0.9238795325112867385, 1.000000000000000000, 0.9238795325112867385, 1.000000000000000000, 0.9238795325112867385, 1.000000000000000000, 0.9238795325112867385, 1.000000000000000000, 0.9238795325112867385, 1.000000000000000000, 0.9238795325112867385, 1.000000000000000000, 0.9238795325112867385, 1.000000000000000000, 0.9238795325112867385, 1.000000000000000000, 0.9238795325112867385, 1.000000000000000000, 0.9238795325112867385, 1.000000000000000000, 0.9238795325112867385, 1.000000000000000000, 0.9238795325112867385, 1.000000000000000000, 0.9238795325112867385, 1.000000000000000000, 0.9238795325112867385, 1.000000000000000000, 0.9238795325112867385, 1.000000000000000000, 0.9238795325112867385, 1.000000000000000000, 0.9238795325112867385, 1.000000000000000000, 0.9238795325112867385, 1.000000000000000000, 0.9238795325112867385, 1.000000000000000000, 0.9238795325112867385, 1.000000000000000000, 0.9238795325112867385, 1.000000000000000000, 0.9238795325112867385, 1.000000000000000000, 0.9238795325112867385, 1.000000000000000000, 0.9238795325112867385, 1.000000000000000000, 0.9238795325112867385, 1.000000000000000000, 0.9238795325112867385, 1.000000000000000000, 0.9238795325112867385, 1.000000000000000000, 0.9238795325112867385, 1.000000000000000000, 0.9238795325112867385, 1.000000000000000000, 0.9238795325112867385, 1.000000000000000000 ) ) 
 REPRESENTATION_ITEM ( '' )  );
#22773=CARTESIAN_POINT ( 'NONE',  ( 96.46446609406721961, 3.535533905932755072, 14.87500000000000000 ) ) ;
#22793=CARTESIAN_POINT ( 'NONE',  ( 97.92893218813451028, -4.999999999999989342, 4.312500002731185056 ) ) ;
#22813=CARTESIAN_POINT ( 'NONE',  ( 97.92893218813451028, -4.999999999999989342, 10.18749999999999822 ) ) ;
#22818=CARTESIAN_POINT ( 'NONE',  ( 103.5355339059327093, -3.535533905932726206, 12.50000000273118594 ) ) ;
#22829=CARTESIAN_POINT ( 'NONE',  ( 99.99999999999995737, -4.458734124999988779, 6.937500001365592972 ) ) ;
#22832=CARTESIAN_POINT ( 'NONE',  ( 99.99999999999995737, -4.458734124999988779, 8.687500001365592084 ) ) ;
#22844=CARTESIAN_POINT ( 'NONE',  ( 95.54126587499996504, 1.387778780781445676E-14, 7.687500001365592084 ) ) ;
#22855=ORIENTED_EDGE ( 'NONE', *, *, #20331, .F. ) ;
#22857=CARTESIAN_POINT ( 'NONE',  ( 99.99999999999995737, 4.458734125000016313, 8.437500001365592084 ) ) ;
#22861=CARTESIAN_POINT ( 'NONE',  ( 102.0710678118654329, -4.999999999999989342, 2.312499999999998668 ) ) ;
#22872=EDGE_LOOP ( 'NONE', ( #25020, #7879, #23282, #13165 ) ) ;
#22888=CARTESIAN_POINT ( 'NONE',  ( 103.1528011352953342, -3.152801135295355106, 14.06250000136559208 ) ) ;
#22905=CARTESIAN_POINT ( 'NONE',  ( 96.46446609406721961, -3.535533905932727539, 4.250000002731185056 ) ) ;
#22955=CARTESIAN_POINT ( 'NONE',  ( 103.5355339059327093, -3.535533905932726206, 10.37499999999999822 ) ) ;
#22960=CARTESIAN_POINT ( 'NONE',  ( 99.99999999999995737, 5.000000000000018652, 12.87500000273118594 ) ) ;
#22969=CARTESIAN_POINT ( 'NONE',  ( 101.8468681455906903, -4.458734124999987891, 7.000000001365592972 ) ) ;
#22970=CARTESIAN_POINT ( 'NONE',  ( 95.54126587499996504, 1.387778780781445676E-14, 10.43750000136559208 ) ) ;
#22983=CARTESIAN_POINT ( 'NONE',  ( 95.54126587499995082, -1.846868145590724986, 8.750000001365592084 ) ) ;
#22994=CARTESIAN_POINT ( 'NONE',  ( 98.15313185440923860, -4.458734124999987891, 3.875000001365591640 ) ) ;
#23003=CARTESIAN_POINT ( 'NONE',  ( 99.99999999999995737, 1.387778780781445676E-14, 0.000000000000000000 ) ) ;
#23006=CARTESIAN_POINT ( 'NONE',  ( 103.5355339059327093, -3.535533905932726206, 6.500000002731185944 ) ) ;
#23026=CARTESIAN_POINT ( 'NONE',  ( 103.1528011352953342, -3.152801135295355106, 1.812500001365591640 ) ) ;
#23029=CARTESIAN_POINT ( 'NONE',  ( 102.0710678118654329, 5.000000000000018652, 13.68750000000000000 ) ) ;
#23043=CARTESIAN_POINT ( 'NONE',  ( 104.9999999999999574, 2.071067811865491937, 4.687500002731185944 ) ) ;
#23058=CARTESIAN_POINT ( 'NONE',  ( 98.15313185440925281, 4.458734125000016313, 12.25000000136559208 ) ) ;
#23068=EDGE_CURVE ( 'NONE', #24537, #2357, #5178, .T. ) ;
#23087=CARTESIAN_POINT ( 'NONE',  ( 94.99999999999995737, 2.071067811865491048, 9.937499999999996447 ) ) ;
#23093=CARTESIAN_POINT ( 'NONE',  ( 96.46446609406721961, 3.535533905932755072, 13.00000000273118417 ) ) ;
#23103=CARTESIAN_POINT ( 'NONE',  ( 96.84719886470459471, 3.152801135295383084, 2.562500001365592084 ) ) ;
#23105=CARTESIAN_POINT ( 'NONE',  ( 99.99999999999995737, 4.458734125000016313, 5.187500001365592972 ) ) ;
#23108=CARTESIAN_POINT ( 'NONE',  ( 94.99999999999995737, -2.071067811865466624, 4.062499999999998224 ) ) ;
#23118=VERTEX_POINT ( 'NONE', #11489 ) ;
#23120=CARTESIAN_POINT ( 'NONE',  ( 96.84719886470459471, 3.152801135295383084, 7.562500001365592084 ) ) ;
#23133=CARTESIAN_POINT ( 'NONE',  ( 101.8468681455907046, 4.458734125000016313, 2.375000001365592084 ) ) ;
#23138=EDGE_CURVE ( 'NONE', #13477, #6975, #23299, .T. ) ;
#23144=DIRECTION ( 'NONE',  ( 0.8660254037844404840, -0.000000000000000000, -0.4999999999999967804 ) ) ;
#23153=ORIENTED_EDGE ( 'NONE', *, *, #27781, .F. ) ;
#23155=PRODUCT_DEFINITION_FORMATION_WITH_SPECIFIED_SOURCE ( 'ANY', '', #12815, .NOT_KNOWN. ) ;
#23159=LINE ( 'NONE', #5773, #27758 ) ;
#23173=CARTESIAN_POINT ( 'NONE',  ( 99.99999999999995737, -4.999999999999990230, 6.249999999999998224 ) ) ;
#23179=( BOUNDED_CURVE ( )  B_SPLINE_CURVE ( 2, ( #11308, #20171, #26590, #7038, #653, #7326, #26732, #11591, #20311 ),
 .UNSPECIFIED., .F., .T. ) 
 B_SPLINE_CURVE_WITH_KNOTS ( ( 3, 2, 2, 2, 3 ),
 ( 0.6071428571428570953, 0.6160714285714286031, 0.6250000000000000000, 0.6339285714285712858, 0.6428571428571427937 ),
 .UNSPECIFIED. ) 
 CURVE ( )  GEOMETRIC_REPRESENTATION_ITEM ( )  RATIONAL_B_SPLINE_CURVE ( ( 1.000000000000000000, 0.9238795325112867385, 1.000000000000000000, 0.9238795325112867385, 1.000000000000000000, 0.9238795325112867385, 1.000000000000000000, 0.9238795325112877377, 0.9999999999999990008 ) ) 
 REPRESENTATION_ITEM ( '' )  );
#23182=CARTESIAN_POINT ( 'NONE',  ( 96.46446609406721961, 3.535533905932755072, 4.000000002731185056 ) ) ;
#23188=CARTESIAN_POINT ( 'NONE',  ( 104.9999999999999716, 1.449011120738813565E-14, 9.625000002731184168 ) ) ;
#23201=CARTESIAN_POINT ( 'NONE',  ( 104.4587341249999781, -1.846868145590721655, 12.87500000136559208 ) ) ;
#23226=CARTESIAN_POINT ( 'NONE',  ( 96.46446609406721961, -3.535533905932727539, 11.12500000000000000 ) ) ;
#23233=CARTESIAN_POINT ( 'NONE',  ( 99.99999999999995737, -4.999999999999990230, 11.25000000000000000 ) ) ;
#23240=CARTESIAN_POINT ( 'NONE',  ( 103.1528011352953342, 3.152801135295383084, 1.312500001365592750 ) ) ;
#23242=CARTESIAN_POINT ( 'NONE',  ( 101.8468681455907046, -4.458734124999987891, 4.750000001365592084 ) ) ;
#23245=CARTESIAN_POINT ( 'NONE',  ( 103.5355339059327093, -3.535533905932726206, 4.374999999999999112 ) ) ;
#23257=CARTESIAN_POINT ( 'NONE',  ( 101.8468681455906903, -4.458734124999987891, 8.000000001365592084 ) ) ;
#23273=CARTESIAN_POINT ( 'NONE',  ( 96.84719886470459471, 3.152801135295383084, 2.312500001365592084 ) ) ;
#23274=CARTESIAN_POINT ( 'NONE',  ( 97.92893218813451028, 5.000000000000018652, 3.937500002731185056 ) ) ;
#23275=CARTESIAN_POINT ( 'NONE',  ( 99.99999999999995737, -4.458734124999988779, 3.937500001365591640 ) ) ;
#23281=CARTESIAN_POINT ( 'NONE',  ( 99.99999999999995737, 1.387778780781445676E-14, 34.79898987322334136 ) ) ;
#23282=ORIENTED_EDGE ( 'NONE', *, *, #17680, .T. ) ;
#23291=DIRECTION ( 'NONE',  ( -1.000000000000000000, 0.000000000000000000, 0.000000000000000000 ) ) ;
#23299=( BOUNDED_CURVE ( )  B_SPLINE_CURVE ( 2, ( #15638, #24766, #5247, #15909, #13485, #11207, #7220, #24339, #982 ),
 .UNSPECIFIED., .F., .F. ) 
 B_SPLINE_CURVE_WITH_KNOTS ( ( 3, 2, 2, 2, 3 ),
 ( 0.5714285714285713969, 0.5803571428571429047, 0.5892857142857143016, 0.5982142857142856984, 0.6071428571428570953 ),
 .UNSPECIFIED. ) 
 CURVE ( )  GEOMETRIC_REPRESENTATION_ITEM ( )  RATIONAL_B_SPLINE_CURVE ( ( 1.000000000000000000, 0.9238795325112867385, 1.000000000000000000, 0.9238795325112867385, 1.000000000000000000, 0.9238795325112867385, 1.000000000000000000, 0.9238795325112867385, 1.000000000000000000 ) ) 
 REPRESENTATION_ITEM ( '' )  );
#23301=DIRECTION ( 'NONE',  ( -1.000000000000000000, 0.000000000000000000, 0.000000000000000000 ) ) ;
#23318=CARTESIAN_POINT ( 'NONE',  ( 94.99999999999995737, -2.071067811865466624, 4.187500002731185056 ) ) ;
#23325=CARTESIAN_POINT ( 'NONE',  ( 104.9999999999999716, 1.449011120738813565E-14, 9.625000002731184168 ) ) ;
#23332=CYLINDRICAL_SURFACE ( 'NONE', #11800, 5.000000000000004441 ) ;
#23333=CARTESIAN_POINT ( 'NONE',  ( 101.8468681455906903, -4.458734124999987891, 12.75000000136559386 ) ) ;
#23352=CARTESIAN_POINT ( 'NONE',  ( 97.92893218813451028, 5.000000000000018652, 7.812499999999999112 ) ) ;
#23359=EDGE_LOOP ( 'NONE', ( #16125, #4751, #24060, #11124 ) ) ;
#23361=CARTESIAN_POINT ( 'NONE',  ( 104.9999999999999574, -2.071067811865462627, 8.437500000000000000 ) ) ;
#23374=DIRECTION ( 'NONE',  ( -1.000000000000000000, 0.000000000000000000, 0.000000000000000000 ) ) ;
#23375=CARTESIAN_POINT ( 'NONE',  ( 104.4587341249999639, 1.442382525525748735E-14, 3.187500001365592972 ) ) ;
#23378=CARTESIAN_POINT ( 'NONE',  ( 96.84719886470459471, 3.152801135295383084, 6.312500001365592084 ) ) ;
#23381=DIRECTION ( 'NONE',  ( -1.000000000000000000, 0.000000000000000000, 0.000000000000000000 ) ) ;
#23388=ORIENTED_EDGE ( 'NONE', *, *, #23138, .F. ) ;
#23392=CARTESIAN_POINT ( 'NONE',  ( 99.99999999999995737, -4.458734124999988779, 6.937500001365592972 ) ) ;
#23406=CARTESIAN_POINT ( 'NONE',  ( 103.1528011352953342, -3.152801135295355106, 5.812500001365591196 ) ) ;
#23408=CARTESIAN_POINT ( 'NONE',  ( 96.84719886470459471, -3.152801135295355994, 3.812500001365591640 ) ) ;
#23427=ORIENTED_EDGE ( 'NONE', *, *, #24668, .T. ) ;
#23439=CARTESIAN_POINT ( 'NONE',  ( 98.15313185440923860, -4.458734124999987891, 13.87500000136559208 ) ) ;
#23444=LINE ( 'NONE', #3922, #8610 ) ;
#23454=CARTESIAN_POINT ( 'NONE',  ( 101.8468681455906903, 4.458734125000016313, 14.12500000136559208 ) ) ;
#23461=CARTESIAN_POINT ( 'NONE',  ( 104.9999999999999716, -2.071067811865452857, 9.562500002731184168 ) ) ;
#23463=CARTESIAN_POINT ( 'NONE',  ( 96.46446609406721961, 3.535533905932755072, 10.00000000273118594 ) ) ;
#23465=AXIS2_PLACEMENT_3D ( 'NONE', #15032, #1817, #12471 ) ;
#23469=CARTESIAN_POINT ( 'NONE',  ( 104.9999999999999716, -2.071067811865452857, 10.43749999999999822 ) ) ;
#23472=CARTESIAN_POINT ( 'NONE',  ( 95.54126587499995082, -1.846868145590724986, 12.50000000136559208 ) ) ;
#23478=CARTESIAN_POINT ( 'NONE',  ( 94.99999999999995737, 2.071067811865491493, 2.937499999999999112 ) ) ;
#23498=CARTESIAN_POINT ( 'NONE',  ( 96.46446609406721961, 3.535533905932755072, 6.874999999999999112 ) ) ;
#23512=CYLINDRICAL_SURFACE ( 'NONE', #25981, 5.000000000000004441 ) ;
#23513=CARTESIAN_POINT ( 'NONE',  ( 98.15313185440925281, -4.458734124999987891, 3.875000001365592084 ) ) ;
#23515=CARTESIAN_POINT ( 'NONE',  ( 95.54126587499996504, 1.387778780781445676E-14, 5.437500001365591196 ) ) ;
#23518=VECTOR ( 'NONE', #10890, 1000.000000000000000 ) ;
#23530=DIRECTION ( 'NONE',  ( -0.000000000000000000, -0.000000000000000000, -1.000000000000000000 ) ) ;
#23531=CARTESIAN_POINT ( 'NONE',  ( 95.54126587499996504, 1.387778780781445676E-14, 1.687500001365591418 ) ) ;
#23532=EDGE_CURVE ( 'NONE', #5414, #5755, #5657, .T. ) ;
#23545=CARTESIAN_POINT ( 'NONE',  ( 98.15313185440925281, 4.458734125000016313, 13.50000000136559208 ) ) ;
#23547=CARTESIAN_POINT ( 'NONE',  ( 95.54126587499995082, 1.846868145590750077, 3.375000001365592972 ) ) ;
#23549=CARTESIAN_POINT ( 'NONE',  ( 96.84719886470459471, 3.152801135295383084, 4.562500001365592084 ) ) ;
#23558=CARTESIAN_POINT ( 'NONE',  ( 97.92893218813451028, 5.000000000000018652, 5.812500000000000000 ) ) ;
#23574=VERTEX_POINT ( 'NONE', #6908 ) ;
#23590=CARTESIAN_POINT ( 'NONE',  ( 104.9999999999999716, 1.449011120738813565E-14, 2.625000002731185500 ) ) ;
#23594=DIRECTION ( 'NONE',  ( -0.000000000000000000, -0.000000000000000000, -1.000000000000000000 ) ) ;
#23597=EDGE_CURVE ( 'NONE', #24544, #2199, #16386, .T. ) ;
#23608=DIRECTION ( 'NONE',  ( 1.000000000000000000, 0.000000000000000000, 0.000000000000000000 ) ) ;
#23610=CARTESIAN_POINT ( 'NONE',  ( 95.54126587499995082, 1.846868145590750077, 9.375000001365592084 ) ) ;
#23614=CARTESIAN_POINT ( 'NONE',  ( 95.54126587499996504, 1.387778780781445676E-14, 12.43750000136559208 ) ) ;
#23624=DIRECTION ( 'NONE',  ( 0.8660254037844404840, 0.000000000000000000, 0.4999999999999967804 ) ) ;
#23638=CARTESIAN_POINT ( 'NONE',  ( 94.99999999999995737, 1.387778780781445676E-14, 4.000000000000000000 ) ) ;
#23646=CARTESIAN_POINT ( 'NONE',  ( 99.99999999999995737, 5.000000000000018652, 4.875000002731185944 ) ) ;
#23653=CARTESIAN_POINT ( 'NONE',  ( 99.99999999999995737, -4.458734124999988779, 4.937500001365592972 ) ) ;
#23655=CARTESIAN_POINT ( 'NONE',  ( 96.84719886470459471, 3.152801135295383084, 7.312500001365592084 ) ) ;
#23661=LINE ( 'NONE', #2140, #7136 ) ;
#23671=CARTESIAN_POINT ( 'NONE',  ( 103.1528011352953342, 3.152801135295383084, 4.312500001365592084 ) ) ;
#23685=CARTESIAN_POINT ( 'NONE',  ( 96.46446609406721961, 3.535533905932755072, 9.874999999999998224 ) ) ;
#23686=CARTESIAN_POINT ( 'NONE',  ( 96.84719886470459471, 3.152801135295383084, 2.312500001365592084 ) ) ;
#23688=CARTESIAN_POINT ( 'NONE',  ( 95.54126587499996504, 1.387778780781445676E-14, 4.437500001365592084 ) ) ;
#23689=CARTESIAN_POINT ( 'NONE',  ( 99.99999999999995737, 5.000000000000018652, 3.875000002731185056 ) ) ;
#23701=ORIENTED_EDGE ( 'NONE', *, *, #26598, .T. ) ;
#23705=ORIENTED_EDGE ( 'NONE', *, *, #8241, .T. ) ;
#23725=ADVANCED_FACE ( 'NONE', ( #17747 ), #6768, .F. ) ;
#23734=CARTESIAN_POINT ( 'NONE',  ( 94.99999999999995737, 2.071067811865491048, 1.062500002731185944 ) ) ;
#23746=CARTESIAN_POINT ( 'NONE',  ( 94.99999999999995737, 1.387778780781445676E-14, 9.999999999999998224 ) ) ;
#23747=CARTESIAN_POINT ( 'NONE',  ( 104.4587341249999781, 1.846868145590750299, 10.00000000136559208 ) ) ;
#23750=CARTESIAN_POINT ( 'NONE',  ( 99.99999999999995737, -4.458734124999988779, 13.68750000136559208 ) ) ;
#23758=EDGE_CURVE ( 'NONE', #2357, #24537, #7909, .T. ) ;
#23772=CARTESIAN_POINT ( 'NONE',  ( 103.5355339059327093, -3.535533905932726206, 5.375000000000000000 ) ) ;
#23778=CARTESIAN_POINT ( 'NONE',  ( 104.9999999999999716, 2.071067811865491937, 6.562499999999998224 ) ) ;
#23790=CARTESIAN_POINT ( 'NONE',  ( 99.99999999999995737, -4.458734124999988779, 0.6875000013655923059 ) ) ;
#23795=DIRECTION ( 'NONE',  ( 0.000000000000000000, 0.000000000000000000, -1.000000000000000000 ) ) ;
#23804=EDGE_LOOP ( 'NONE', ( #9813, #6412, #22002 ) ) ;
#23806=CARTESIAN_POINT ( 'NONE',  ( 104.4587341249999639, 1.442382525525748735E-14, 3.187500001365592972 ) ) ;
#23822=CARTESIAN_POINT ( 'NONE',  ( 95.54126587499996504, 1.387778780781445676E-14, 13.68750000136559386 ) ) ;
#23824=CARTESIAN_POINT ( 'NONE',  ( 96.84719886470459471, 3.152801135295383084, 13.31250000136559386 ) ) ;
#23856=CARTESIAN_POINT ( 'NONE',  ( 99.99999999999995737, 4.458734125000016313, 11.43750000136559208 ) ) ;
#23865=ORIENTED_EDGE ( 'NONE', *, *, #22029, .F. ) ;
#23870=CARTESIAN_POINT ( 'NONE',  ( 102.0710678118654329, -4.999999999999989342, 3.437500002731184612 ) ) ;
#23887=CARTESIAN_POINT ( 'NONE',  ( 99.99999999999995737, 4.458734125000016313, 8.187500001365592084 ) ) ;
#23888=VERTEX_POINT ( 'NONE', #16316 ) ;
#23890=CARTESIAN_POINT ( 'NONE',  ( 95.54126587499995082, 1.846868145590750077, 13.37500000136559386 ) ) ;
#23911=CARTESIAN_POINT ( 'NONE',  ( 103.5355339059327093, -3.535533905932726206, 6.374999999999999112 ) ) ;
#23948=CARTESIAN_POINT ( 'NONE',  ( 101.8468681455906903, -4.458734124999987891, 2.000000001365591640 ) ) ;
#23964=CARTESIAN_POINT ( 'NONE',  ( 103.1528011352953342, -3.152801135295355106, 12.06250000136559208 ) ) ;
#23966=CARTESIAN_POINT ( 'NONE',  ( 98.15313185440923860, 4.458734125000016313, 13.25000000136559564 ) ) ;
#23983=CARTESIAN_POINT ( 'NONE',  ( 99.99999999999995737, 4.458734125000016313, 13.43750000136559386 ) ) ;
#23991=VECTOR ( 'NONE', #2733, 1000.000000000000000 ) ;
#23995=EDGE_CURVE ( 'NONE', #25848, #11744, #15105, .T. ) ;
#24001=CARTESIAN_POINT ( 'NONE',  ( 98.15313185440923860, 4.458734125000016313, 9.500000001365593860 ) ) ;
#24013=CARTESIAN_POINT ( 'NONE',  ( 94.99999999999995737, -2.071067811865466624, 0.1875000027311852502 ) ) ;
#24018=FACE_OUTER_BOUND ( 'NONE', #27566, .T. ) ;
#24019=SURFACE_STYLE_FILL_AREA ( #219 ) ;
#24028=DIRECTION ( 'NONE',  ( 0.000000000000000000, 0.000000000000000000, 1.000000000000000000 ) ) ;
#24029=CARTESIAN_POINT ( 'NONE',  ( 103.1528011352953342, -3.152801135295355106, 6.812500001365592084 ) ) ;
#24031=CARTESIAN_POINT ( 'NONE',  ( 101.8468681455906903, -4.458734124999987891, 12.75000000136559386 ) ) ;
#24039=( BOUNDED_CURVE ( )  B_SPLINE_CURVE ( 2, ( #20952, #5844, #27783, #5979, #20814, #14646, #1292, #1162, #14514 ),
 .UNSPECIFIED., .F., .F. ) 
 B_SPLINE_CURVE_WITH_KNOTS ( ( 3, 2, 2, 2, 3 ),
 ( 0.000000000000000000, 0.008928571428571436749, 0.01785714285714287350, 0.02678571428571431198, 0.03571428571428574700 ),
 .UNSPECIFIED. ) 
 CURVE ( )  GEOMETRIC_REPRESENTATION_ITEM ( )  RATIONAL_B_SPLINE_CURVE ( ( 1.000000000000000000, 0.9238795325112867385, 1.000000000000000000, 0.9238795325112867385, 1.000000000000000000, 0.9238795325112867385, 1.000000000000000000, 0.9238795325112864054, 1.000000000000000222 ) ) 
 REPRESENTATION_ITEM ( '' )  );
#24045=ORIENTED_EDGE ( 'NONE', *, *, #14556, .T. ) ;
#24054=CARTESIAN_POINT ( 'NONE',  ( 102.0710678118654329, 5.000000000000018652, 6.687499999999999112 ) ) ;
#24056=MECHANICAL_DESIGN_GEOMETRIC_PRESENTATION_REPRESENTATION('',(#24512),#9022);
#24060=ORIENTED_EDGE ( 'NONE', *, *, #20331, .T. ) ;
#24072=CARTESIAN_POINT ( 'NONE',  ( 96.84719886470459471, 3.152801135295383084, 2.312500001365592084 ) ) ;
#24089=CARTESIAN_POINT ( 'NONE',  ( 94.99999999999995737, 1.387778780781445676E-14, 0.000000000000000000 ) ) ;
#24090=CARTESIAN_POINT ( 'NONE',  ( 98.15313185440925281, -4.458734124999987891, 2.875000001365592084 ) ) ;
#24102=CARTESIAN_POINT ( 'NONE',  ( 98.15313185440925281, 4.458734125000016313, 10.50000000136559208 ) ) ;
#24105=CARTESIAN_POINT ( 'NONE',  ( 101.8468681455906903, 4.458734125000016313, 1.125000001365592750 ) ) ;
#24108=CYLINDRICAL_SURFACE ( 'NONE', #15250, 5.000000000000004441 ) ;
#24123=EDGE_CURVE ( 'NONE', #22244, #9281, #8454, .T. ) ;
#24125=CARTESIAN_POINT ( 'NONE',  ( 99.99999999999995737, -4.458734124999988779, 13.93750000136559208 ) ) ;
#24139=CARTESIAN_POINT ( 'NONE',  ( 95.54126587499996504, 1.387778780781445676E-14, 10.68750000136559208 ) ) ;
#24172=CARTESIAN_POINT ( 'NONE',  ( 103.1528011352953342, -3.152801135295355106, 9.812500001365593860 ) ) ;
#24175=CARTESIAN_POINT ( 'NONE',  ( 104.4587341249999781, 1.846868145590750299, 11.00000000136559208 ) ) ;
#24191=CARTESIAN_POINT ( 'NONE',  ( 94.99999999999995737, 2.071067811865491048, 8.062500002731185944 ) ) ;
#24197=CARTESIAN_POINT ( 'NONE',  ( 94.99999999999995737, -2.071067811865466624, 1.062499999999999334 ) ) ;
#24215=CARTESIAN_POINT ( 'NONE',  ( 104.4587341249999781, 1.846868145590750521, 1.000000001365592528 ) ) ;
#24230=CARTESIAN_POINT ( 'NONE',  ( 99.99999999999995737, 5.000000000000018652, 11.75000000000000000 ) ) ;
#24243=CARTESIAN_POINT ( 'NONE',  ( 101.8468681455906903, -4.458734124999987891, 10.00000000136559386 ) ) ;
#24245=CARTESIAN_POINT ( 'NONE',  ( 99.99999999999995737, -4.458734124999988779, 0.6875000013655923059 ) ) ;
#24255=( BOUNDED_CURVE ( )  B_SPLINE_CURVE ( 2, ( #27622, #5818, #3680, #18912, #8080, #16775, #10485, #4653, #22180 ),
 .UNSPECIFIED., .F., .T. ) 
 B_SPLINE_CURVE_WITH_KNOTS ( ( 3, 2, 2, 2, 3 ),
 ( 0.4285714285714285476, 0.4375000000000000000, 0.4464285714285713969, 0.4553571428571427937, 0.4642857142857142461 ),
 .UNSPECIFIED. ) 
 CURVE ( )  GEOMETRIC_REPRESENTATION_ITEM ( )  RATIONAL_B_SPLINE_CURVE ( ( 1.000000000000000000, 0.9238795325112867385, 1.000000000000000000, 0.9238795325112867385, 1.000000000000000000, 0.9238795325112867385, 1.000000000000000000, 0.9238795325112871826, 0.9999999999999995559 ) ) 
 REPRESENTATION_ITEM ( '' )  );
#24279=CARTESIAN_POINT ( 'NONE',  ( 98.15313185440923860, 4.458734125000016313, 12.50000000136559208 ) ) ;
#24297=CARTESIAN_POINT ( 'NONE',  ( 94.99999999999994316, 2.071067811865481278, 11.06250000273118594 ) ) ;
#24298=PRESENTATION_STYLE_ASSIGNMENT (( #10888 ) ) ;
#24305=CARTESIAN_POINT ( 'NONE',  ( 104.4587341249999781, -1.846868145590721655, 5.875000001365591196 ) ) ;
#24308=CARTESIAN_POINT ( 'NONE',  ( 104.4587341249999781, 1.846868145590750299, 7.000000001365591196 ) ) ;
#24312=CARTESIAN_POINT ( 'NONE',  ( 99.99999999999995737, 5.000000000000018652, 6.875000002731185056 ) ) ;
#24322=ORIENTED_EDGE ( 'NONE', *, *, #15599, .F. ) ;
#24328=CARTESIAN_POINT ( 'NONE',  ( 103.5355339059327093, -3.535533905932726206, 11.50000000273118417 ) ) ;
#24334=CARTESIAN_POINT ( 'NONE',  ( 99.99999999999995737, -4.999999999999990230, 3.249999999999999556 ) ) ;
#24339=CARTESIAN_POINT ( 'NONE',  ( 104.9999999999999716, 2.071067811865491937, 5.687500002731185056 ) ) ;
#24351=CARTESIAN_POINT ( 'NONE',  ( 98.15313185440923860, 4.458734125000016313, 1.250000001365592750 ) ) ;
#24354=CARTESIAN_POINT ( 'NONE',  ( 96.46446609406721961, 3.535533905932755072, 4.874999999999999112 ) ) ;
#24369=CARTESIAN_POINT ( 'NONE',  ( 94.99999999999995737, 2.071067811865491048, 11.93750000000000000 ) ) ;
#24383=CARTESIAN_POINT ( 'NONE',  ( 96.84719886470459471, 3.152801135295383084, 9.562500001365593860 ) ) ;
#24385=CARTESIAN_POINT ( 'NONE',  ( 104.4587341249999781, 1.846868145590750299, 1.000000001365592528 ) ) ;
#24389=LINE ( 'NONE', #15967, #25283 ) ;
#24393=ORIENTED_EDGE ( 'NONE', *, *, #22564, .T. ) ;
#24401=CARTESIAN_POINT ( 'NONE',  ( 103.1528011352953342, -3.152801135295355106, 10.06250000136559386 ) ) ;
#24405=VECTOR ( 'NONE', #19306, 1000.000000000000000 ) ;
#24408=CARTESIAN_POINT ( 'NONE',  ( 94.99999999999995737, 1.387778780781445676E-14, 34.79898987322334136 ) ) ;
#24417=CARTESIAN_POINT ( 'NONE',  ( 101.8468681455907046, -4.458734124999987891, 12.00000000136559208 ) ) ;
#24421=CARTESIAN_POINT ( 'NONE',  ( 103.5355339059327093, -3.535533905932726206, 2.374999999999998668 ) ) ;
#24429=ORIENTED_EDGE ( 'NONE', *, *, #25360, .T. ) ;
#24435=CARTESIAN_POINT ( 'NONE',  ( 94.99999999999995737, -2.071067811865466624, 0.1875000027311852224 ) ) ;
#24437=ORIENTED_EDGE ( 'NONE', *, *, #2814, .T. ) ;
#24444=DIRECTION ( 'NONE',  ( 0.000000000000000000, 0.000000000000000000, 1.000000000000000000 ) ) ;
#24449=CARTESIAN_POINT ( 'NONE',  ( 104.4587341249999781, -1.846868145590721655, 2.875000001365592084 ) ) ;
#24452=CARTESIAN_POINT ( 'NONE',  ( 101.8468681455906903, -4.458734124999987891, 6.750000001365592972 ) ) ;
#24455=CARTESIAN_POINT ( 'NONE',  ( 102.0710678118654329, 5.000000000000018652, 6.812500002731185056 ) ) ;
#24469=CARTESIAN_POINT ( 'NONE',  ( 102.0710678118654329, -4.999999999999989342, 8.312500000000000000 ) ) ;
#24472=CARTESIAN_POINT ( 'NONE',  ( 94.99999999999995737, 2.071067811865491048, 11.06250000273118417 ) ) ;
#24482=DIRECTION ( 'NONE',  ( 1.000000000000000000, 0.000000000000000000, 0.000000000000000000 ) ) ;
#24486=CARTESIAN_POINT ( 'NONE',  ( 99.99999999999995737, 1.387778780781445676E-14, 15.00000000000000000 ) ) ;
#24512=STYLED_ITEM ( 'NONE', ( #19436 ), #26371 ) ;
#24516=CARTESIAN_POINT ( 'NONE',  ( 103.5355339059327093, 3.535533905932755072, 11.62500000000000000 ) ) ;
#24517=ORIENTED_EDGE ( 'NONE', *, *, #9191, .F. ) ;
#24523=CARTESIAN_POINT ( 'NONE',  ( 102.0710678118654329, -4.999999999999989342, 3.312499999999999556 ) ) ;
#24525=DIRECTION ( 'NONE',  ( -0.000000000000000000, -0.000000000000000000, -1.000000000000000000 ) ) ;
#24529=CARTESIAN_POINT ( 'NONE',  ( 96.84719886470459471, 3.152801135295383084, 12.56250000136559208 ) ) ;
#24530=CARTESIAN_POINT ( 'NONE',  ( 95.54126587499996504, -1.846868145590724986, 8.500000001365592084 ) ) ;
#24534=CARTESIAN_POINT ( 'NONE',  ( 94.99999999999995737, 2.071067811865491493, 3.937500000000000000 ) ) ;
#24537=VERTEX_POINT ( 'NONE', #20074 ) ;
#24544=VERTEX_POINT ( 'NONE', #13917 ) ;
#24547=CARTESIAN_POINT ( 'NONE',  ( 104.4587341249999639, 1.442382525525748735E-14, 9.187500001365592084 ) ) ;
#24565=CARTESIAN_POINT ( 'NONE',  ( 98.15313185440923860, -4.458734124999987891, 8.875000001365592084 ) ) ;
#24567=CARTESIAN_POINT ( 'NONE',  ( 94.99999999999995737, 1.387778780781445676E-14, 7.125000002731185056 ) ) ;
#24568=CARTESIAN_POINT ( 'NONE',  ( 102.0710678118654329, -4.999999999999989342, 14.31249999999999645 ) ) ;
#24583=CARTESIAN_POINT ( 'NONE',  ( 104.9999999999999716, 1.449011120738813565E-14, 10.62500000273118594 ) ) ;
#24584=CARTESIAN_POINT ( 'NONE',  ( 102.0710678118654329, 5.000000000000018652, 8.812500002731184168 ) ) ;
#24589=CARTESIAN_POINT ( 'NONE',  ( 103.5355339059327093, -3.535533905932726206, 2.500000002731185500 ) ) ;
#24598=CARTESIAN_POINT ( 'NONE',  ( 95.54126587499995082, 1.846868145590750077, 4.375000001365592084 ) ) ;
#24600=CARTESIAN_POINT ( 'NONE',  ( 94.99999999999995737, 1.387778780781445676E-14, 4.000000000000000000 ) ) ;
#24601=CARTESIAN_POINT ( 'NONE',  ( 101.8468681455906903, 4.458734125000016313, 8.125000001365592084 ) ) ;
#24611=CARTESIAN_POINT ( 'NONE',  ( 99.99999999999995737, 1.387778780781445676E-14, 0.000000000000000000 ) ) ;
#24617=CARTESIAN_POINT ( 'NONE',  ( 94.99999999999995737, 1.387778780781445676E-14, 9.125000002731184168 ) ) ;
#24623=CARTESIAN_POINT ( 'NONE',  ( 102.0710678118654329, -4.999999999999989342, 2.312499999999998668 ) ) ;
#24625=AXIS2_PLACEMENT_3D ( 'NONE', #18868, #27578, #23301 ) ;
#24632=CARTESIAN_POINT ( 'NONE',  ( 97.92893218813451028, -4.999999999999989342, 10.31250000273118417 ) ) ;
#24657=EDGE_CURVE ( 'NONE', #17053, #5414, #20211, .T. ) ;
#24662=CARTESIAN_POINT ( 'NONE',  ( 96.46446609406721961, 3.535533905932755072, 14.87500000000000000 ) ) ;
#24668=EDGE_CURVE ( 'NONE', #23118, #4924, #24796, .T. ) ;
#24669=LINE ( 'NONE', #5287, #5277 ) ;
#24676=CARTESIAN_POINT ( 'NONE',  ( 95.54126587499996504, 1.387778780781445676E-14, 7.687500001365592084 ) ) ;
#24678=CARTESIAN_POINT ( 'NONE',  ( 101.8468681455907046, -4.458734124999987891, 9.750000001365593860 ) ) ;
#24684=ADVANCED_FACE ( 'NONE', ( #21057 ), #579, .F. ) ;
#24692=CARTESIAN_POINT ( 'NONE',  ( 98.15313185440925281, 4.458734125000016313, 9.500000001365593860 ) ) ;
#24707=CARTESIAN_POINT ( 'NONE',  ( 95.54126587499996504, 1.387778780781445676E-14, 8.687500001365592084 ) ) ;
#24727=CARTESIAN_POINT ( 'NONE',  ( 104.9999999999999716, 1.449011120738813565E-14, 13.50000000000000000 ) ) ;
#24728=CARTESIAN_POINT ( 'NONE',  ( 104.9999999999999716, 1.449011120738813565E-14, 8.625000002731185944 ) ) ;
#24729=CARTESIAN_POINT ( 'NONE',  ( 94.99999999999995737, 1.387778780781445676E-14, 1.125000002731184390 ) ) ;
#24736=CARTESIAN_POINT ( 'NONE',  ( 99.99999999999995737, -4.458734124999988779, 5.687500001365591196 ) ) ;
#24739=CARTESIAN_POINT ( 'NONE',  ( 98.15313185440925281, -4.458734124999987891, 8.625000001365593860 ) ) ;
#24744=CARTESIAN_POINT ( 'NONE',  ( 103.5355339059327093, -3.535533905932726206, 5.375000000000000000 ) ) ;
#24754=CARTESIAN_POINT ( 'NONE',  ( 94.99999999999995737, -2.071067811865466624, 11.18750000273118594 ) ) ;
#24766=CARTESIAN_POINT ( 'NONE',  ( 94.99999999999995737, 2.071067811865491493, 6.062500002731184168 ) ) ;
#24770=DIRECTION ( 'NONE',  ( -1.000000000000000000, 0.000000000000000000, 0.000000000000000000 ) ) ;
#24796=( BOUNDED_CURVE ( )  B_SPLINE_CURVE ( 2, ( #5540, #3113, #2691, #2961, #26637, #20504, #1544, #14751, #21336 ),
 .UNSPECIFIED., .F., .F. ) 
 B_SPLINE_CURVE_WITH_KNOTS ( ( 3, 2, 2, 2, 3 ),
 ( 0.1428571428571428492, 0.1517857142857142738, 0.1607142857142857539, 0.1696428571428571785, 0.1785714285714286031 ),
 .UNSPECIFIED. ) 
 CURVE ( )  GEOMETRIC_REPRESENTATION_ITEM ( )  RATIONAL_B_SPLINE_CURVE ( ( 1.000000000000000000, 0.9238795325112867385, 1.000000000000000000, 0.9238795325112867385, 1.000000000000000000, 0.9238795325112867385, 1.000000000000000000, 0.9238795325112865164, 1.000000000000000222 ) ) 
 REPRESENTATION_ITEM ( '' )  );
#24798=CARTESIAN_POINT ( 'NONE',  ( 97.92893218813451028, 5.000000000000018652, 13.81250000000000000 ) ) ;
#24804=CARTESIAN_POINT ( 'NONE',  ( 102.0710678118654329, -4.999999999999989342, 13.43750000273118772 ) ) ;
#24805=CARTESIAN_POINT ( 'NONE',  ( 99.99999999999995737, -4.999999999999990230, 3.249999999999999556 ) ) ;
#24811=CARTESIAN_POINT ( 'NONE',  ( 103.1528011352953342, -3.152801135295355106, 6.062500001365592084 ) ) ;
#24813=AXIS2_PLACEMENT_3D ( 'NONE', #12739, #17310, #8483 ) ;
#24814=CARTESIAN_POINT ( 'NONE',  ( 99.99999999999995737, 4.458734125000016313, 11.18750000136559208 ) ) ;
#24829=CARTESIAN_POINT ( 'NONE',  ( 104.4587341249999781, 1.846868145590750299, 12.25000000136559208 ) ) ;
#24850=CARTESIAN_POINT ( 'NONE',  ( 99.99999999999995737, 4.458734125000016313, 7.437500001365592084 ) ) ;
#24852=CARTESIAN_POINT ( 'NONE',  ( 106.9999999999999716, 1.473504056721760595E-14, 15.00000000000000000 ) ) ;
#24853=CARTESIAN_POINT ( 'NONE',  ( 104.9999999999999574, -2.071067811865468844, 14.43749999999999645 ) ) ;
#24861=VECTOR ( 'NONE', #23624, 1000.000000000000000 ) ;
#24862=ORIENTED_EDGE ( 'NONE', *, *, #1482, .T. ) ;
#24865=DIRECTION ( 'NONE',  ( -0.000000000000000000, -0.000000000000000000, -1.000000000000000000 ) ) ;
#24876=CARTESIAN_POINT ( 'NONE',  ( 104.9999999999999716, 1.449011120738813565E-14, 34.79898987322334136 ) ) ;
#24880=CARTESIAN_POINT ( 'NONE',  ( 103.1528011352953342, 3.152801135295383084, 5.062500001365592972 ) ) ;
#24883=CARTESIAN_POINT ( 'NONE',  ( 96.84719886470459471, 3.152801135295383084, 8.312500001365592084 ) ) ;
#24887=CARTESIAN_POINT ( 'NONE',  ( 104.9999999999999716, 1.449011120738813565E-14, 5.500000000000000000 ) ) ;
#24899=CARTESIAN_POINT ( 'NONE',  ( 99.99999999999995737, -4.999999999999990230, 6.375000002731185944 ) ) ;
#24904=CARTESIAN_POINT ( 'NONE',  ( 94.99999999999995737, 1.387778780781445676E-14, 11.00000000000000000 ) ) ;
#24912=DIRECTION ( 'NONE',  ( -1.000000000000000000, 0.000000000000000000, 0.000000000000000000 ) ) ;
#24939=CARTESIAN_POINT ( 'NONE',  ( 96.46446609406721961, -3.535533905932727539, 8.125000000000000000 ) ) ;
#24944=CARTESIAN_POINT ( 'NONE',  ( 99.99999999999995737, -4.999999999999990230, 12.37500000273118594 ) ) ;
#24952=CARTESIAN_POINT ( 'NONE',  ( 103.1528011352953342, -3.152801135295355106, 8.062500001365592084 ) ) ;
#24954=EDGE_CURVE ( 'NONE', #26438, #25848, #19510, .T. ) ;
#24955=CARTESIAN_POINT ( 'NONE',  ( 98.15313185440923860, 4.458734125000016313, 9.250000001365592084 ) ) ;
#24965=CARTESIAN_POINT ( 'NONE',  ( 104.9999999999999716, 1.449011120738813565E-14, 2.499999999999998668 ) ) ;
#24969=CARTESIAN_POINT ( 'NONE',  ( 96.84719886470459471, -3.152801135295355994, 12.81250000136559208 ) ) ;
#24987=CARTESIAN_POINT ( 'NONE',  ( 95.54126587499996504, -1.846868145590724986, 6.750000001365592084 ) ) ;
#24991=DIRECTION ( 'NONE',  ( -1.000000000000000000, 0.000000000000000000, 0.000000000000000000 ) ) ;
#25012=CARTESIAN_POINT ( 'NONE',  ( 96.46446609406721961, 3.535533905932755072, 2.000000002731185056 ) ) ;
#25020=ORIENTED_EDGE ( 'NONE', *, *, #27599, .F. ) ;
#25021=CARTESIAN_POINT ( 'NONE',  ( 104.4587341249999639, 1.442382525525748735E-14, 13.18750000136559208 ) ) ;
#25034=EDGE_LOOP ( 'NONE', ( #11000, #24393, #24862, #9143, #16484, #17272, #20809, #1146, #21625, #374, #8147, #23701, #7986, #3538, #26084, #21774, #21338, #15511, #27538, #10312, #15383, #10065, #9688, #4628, #433, #21321, #20737, #3304, #26454, #11305, #18659 ) ) ;
#25038=CARTESIAN_POINT ( 'NONE',  ( 103.5355339059327093, 3.535533905932755072, 4.750000002731185944 ) ) ;
#25056=ORIENTED_EDGE ( 'NONE', *, *, #20365, .F. ) ;
#25081=CARTESIAN_POINT ( 'NONE',  ( 102.0710678118654329, -4.999999999999989342, 9.312499999999998224 ) ) ;
#25086=CARTESIAN_POINT ( 'NONE',  ( 94.99999999999995737, 1.387778780781445676E-14, 14.12500000273118594 ) ) ;
#25096=CARTESIAN_POINT ( 'NONE',  ( 101.8468681455906903, 4.458734125000016313, 8.375000001365592084 ) ) ;
#25099=CARTESIAN_POINT ( 'NONE',  ( 95.54126587499996504, 1.846868145590750077, 9.375000001365593860 ) ) ;
#25109=CARTESIAN_POINT ( 'NONE',  ( 103.1528011352953342, -3.152801135295355106, 8.062500001365592084 ) ) ;
#25122=CARTESIAN_POINT ( 'NONE',  ( 95.54126587499996504, -1.846868145590724986, 3.750000001365591640 ) ) ;
#25151=CARTESIAN_POINT ( 'NONE',  ( 99.99999999999995737, -4.458734124999988779, 0.6875000013655923059 ) ) ;
#25169=CARTESIAN_POINT ( 'NONE',  ( 103.5355339059327093, -3.535533905932726206, 7.500000002731185944 ) ) ;
#25173=ORIENTED_EDGE ( 'NONE', *, *, #22101, .T. ) ;
#25188=CARTESIAN_POINT ( 'NONE',  ( 98.15313185440925281, -4.458734124999987891, 13.62500000136559208 ) ) ;
#25196=ADVANCED_FACE ( 'NONE', ( #13605 ), #668, .F. ) ;
#25216=CARTESIAN_POINT ( 'NONE',  ( 99.99999999999995737, 5.000000000000018652, 7.749999999999999112 ) ) ;
#25222=CARTESIAN_POINT ( 'NONE',  ( 102.0710678118654329, 5.000000000000018652, 13.81250000273118594 ) ) ;
#25224=CARTESIAN_POINT ( 'NONE',  ( 99.99999999999995737, 1.387778780781445676E-14, 34.79898987322334136 ) ) ;
#25230=CARTESIAN_POINT ( 'NONE',  ( 98.15313185440925281, 4.458734125000016313, 5.500000001365592972 ) ) ;
#25232=CARTESIAN_POINT ( 'NONE',  ( 104.4587341249999781, 1.846868145590750521, 6.000000001365592084 ) ) ;
#25246=CARTESIAN_POINT ( 'NONE',  ( 104.4587341249999781, -1.846868145590721655, 6.125000001365591196 ) ) ;
#25259=CARTESIAN_POINT ( 'NONE',  ( 95.54126587499996504, 1.846868145590750077, 1.625000001365593416 ) ) ;
#25263=CYLINDRICAL_SURFACE ( 'NONE', #1078, 5.000000000000004441 ) ;
#25264=ORIENTED_EDGE ( 'NONE', *, *, #9306, .F. ) ;
#25272=CYLINDRICAL_SURFACE ( 'NONE', #21242, 5.000000000000004441 ) ;
#25274=EDGE_LOOP ( 'NONE', ( #14856, #282, #20807, #5595, #9041, #8685 ) ) ;
#25280=CARTESIAN_POINT ( 'NONE',  ( 94.99999999999995737, 1.387778780781445676E-14, 2.125000002731185056 ) ) ;
#25282=AXIS2_PLACEMENT_3D ( 'NONE', #20245, #11818, #14099 ) ;
#25283=VECTOR ( 'NONE', #7131, 1000.000000000000000 ) ;
#25291=CARTESIAN_POINT ( 'NONE',  ( 101.8468681455906903, 4.458734125000016313, 14.37500000136559386 ) ) ;
#25292=CARTESIAN_POINT ( 'NONE',  ( 96.84719886470459471, -3.152801135295355994, 13.81250000136559208 ) ) ;
#25305=ORIENTED_EDGE ( 'NONE', *, *, #3443, .F. ) ;
#25309=CARTESIAN_POINT ( 'NONE',  ( 94.99999999999995737, 2.071067811865491048, 5.062500002731185944 ) ) ;
#25327=CARTESIAN_POINT ( 'NONE',  ( 101.8468681455906903, -4.458734124999987891, 13.75000000136559208 ) ) ;
#25329=ORIENTED_EDGE ( 'NONE', *, *, #3035, .F. ) ;
#25347=CARTESIAN_POINT ( 'NONE',  ( 104.9999999999999716, 2.071067811865491937, 7.562499999999999112 ) ) ;
#25359=CARTESIAN_POINT ( 'NONE',  ( 94.99999999999995737, -2.071067811865466624, 9.062499999999998224 ) ) ;
#25360=EDGE_CURVE ( 'NONE', #9281, #4419, #22048, .T. ) ;
#25375=CARTESIAN_POINT ( 'NONE',  ( 103.1528011352953342, 3.152801135295383084, 2.312500001365592084 ) ) ;
#25377=CARTESIAN_POINT ( 'NONE',  ( 98.15313185440923860, 4.458734125000016313, 7.250000001365592084 ) ) ;
#25392=CARTESIAN_POINT ( 'NONE',  ( 103.1528011352953342, -3.152801135295355106, 5.062500001365592972 ) ) ;
#25406=CARTESIAN_POINT ( 'NONE',  ( 103.1528011352953342, 3.152801135295383084, 5.062500001365592972 ) ) ;
#25408=CARTESIAN_POINT ( 'NONE',  ( 104.4587341249999639, 1.442382525525748735E-14, 1.187500001365592750 ) ) ;
#25425=FACE_OUTER_BOUND ( 'NONE', #3562, .T. ) ;
#25427=CARTESIAN_POINT ( 'NONE',  ( 92.99999999999995737, 1.387778780781445676E-14, 34.79898987322334136 ) ) ;
#25436=VERTEX_POINT ( 'NONE', #24852 ) ;
#25439=VECTOR ( 'NONE', #23530, 1000.000000000000000 ) ;
#25440=CARTESIAN_POINT ( 'NONE',  ( 94.99999999999997158, 2.071067811865503483, 13.93749999999999467 ) ) ;
#25449=UNCERTAINTY_MEASURE_WITH_UNIT (LENGTH_MEASURE( 1.000000000000000082E-05 ), #27860, 'distance_accuracy_value', 'NONE');
#25452=CARTESIAN_POINT ( 'NONE',  ( 96.46446609406721961, 3.535533905932755072, 6.000000002731185056 ) ) ;
#25469=FACE_OUTER_BOUND ( 'NONE', #875, .T. ) ;
#25470=CARTESIAN_POINT ( 'NONE',  ( 96.84719886470459471, -3.152801135295355994, 11.56250000136559208 ) ) ;
#25481=CARTESIAN_POINT ( 'NONE',  ( 104.9999999999999574, 2.071067811865501263, 11.56249999999999822 ) ) ;
#25495=CARTESIAN_POINT ( 'NONE',  ( 102.0710678118654329, 5.000000000000018652, 9.687499999999998224 ) ) ;
#25510=CARTESIAN_POINT ( 'NONE',  ( 95.54126587499995082, 1.846868145590750077, 2.625000001365592084 ) ) ;
#25513=CARTESIAN_POINT ( 'NONE',  ( 101.8468681455907046, -4.458734124999987891, 7.750000001365592084 ) ) ;
#25527=CARTESIAN_POINT ( 'NONE',  ( 96.84719886470459471, 3.152801135295383084, 5.562500001365592972 ) ) ;
#25528=VERTEX_POINT ( 'NONE', #24567 ) ;
#25543=CARTESIAN_POINT ( 'NONE',  ( 104.4587341249999781, 1.846868145590750299, 3.000000001365592528 ) ) ;
#25545=CARTESIAN_POINT ( 'NONE',  ( 103.1528011352953342, -3.152801135295355106, 4.062500001365592084 ) ) ;
#25561=ORIENTED_EDGE ( 'NONE', *, *, #12726, .T. ) ;
#25562=CARTESIAN_POINT ( 'NONE',  ( 97.92893218813451028, 5.000000000000018652, 1.937500002731185500 ) ) ;
#25572=FILL_AREA_STYLE ('',( #6462 ) ) ;
#25578=CYLINDRICAL_SURFACE ( 'NONE', #10921, 5.000000000000004441 ) ;
#25585=CARTESIAN_POINT ( 'NONE',  ( 104.9999999999999574, -2.071067811865462627, 0.5625000027311858330 ) ) ;
#25589=CYLINDRICAL_SURFACE ( 'NONE', #20254, 7.000000000000006217 ) ;
#25591=CARTESIAN_POINT ( 'NONE',  ( 94.99999999999994316, -2.071067811865456409, 9.187500002731182391 ) ) ;
#25599=CARTESIAN_POINT ( 'NONE',  ( 96.84719886470459471, 3.152801135295383084, 14.31250000136559208 ) ) ;
#25600=CARTESIAN_POINT ( 'NONE',  ( 102.0710678118654329, -4.999999999999989342, 13.43750000273118594 ) ) ;
#25607=CARTESIAN_POINT ( 'NONE',  ( 103.5355339059327093, 3.535533905932755072, 2.624999999999998668 ) ) ;
#25618=ORIENTED_EDGE ( 'NONE', *, *, #11909, .F. ) ;
#25619=CARTESIAN_POINT ( 'NONE',  ( 94.99999999999995737, 1.387778780781445676E-14, 8.000000000000000000 ) ) ;
#25629=CARTESIAN_POINT ( 'NONE',  ( 104.9999999999999574, -2.071067811865462627, 3.437499999999999556 ) ) ;
#25634=CARTESIAN_POINT ( 'NONE',  ( 94.99999999999995737, 1.387778780781445676E-14, 11.00000000000000000 ) ) ;
#25641=CARTESIAN_POINT ( 'NONE',  ( 104.4587341249999639, 1.442382525525748735E-14, 2.187500001365592084 ) ) ;
#25643=CARTESIAN_POINT ( 'NONE',  ( 96.84719886470459471, -3.152801135295355994, 4.562500001365592084 ) ) ;
#25658=LINE ( 'NONE', #14806, #25439 ) ;
#25659=CARTESIAN_POINT ( 'NONE',  ( 95.54126587499995082, -1.846868145590724986, 7.750000001365592084 ) ) ;
#25676=CARTESIAN_POINT ( 'NONE',  ( 96.84719886470459471, 3.152801135295383084, 5.312500001365592972 ) ) ;
#25677=CARTESIAN_POINT ( 'NONE',  ( 104.4587341249999781, -1.846868145590721655, 2.125000001365591640 ) ) ;
#25680=CARTESIAN_POINT ( 'NONE',  ( 96.46446609406721961, 3.535533905932755072, 8.000000002731185944 ) ) ;
#25684=ADVANCED_FACE ( 'NONE', ( #14141 ), #25263, .F. ) ;
#25722=CARTESIAN_POINT ( 'NONE',  ( 102.0710678118654329, -4.999999999999989342, 1.437500002731185056 ) ) ;
#25740=CARTESIAN_POINT ( 'NONE',  ( 103.1528011352953342, -3.152801135295355106, 12.81250000136559208 ) ) ;
#25745=CARTESIAN_POINT ( 'NONE',  ( 99.99999999999995737, 4.458734125000016313, 12.18750000136559208 ) ) ;
#25767=CARTESIAN_POINT ( 'NONE',  ( 97.92893218813451028, -4.999999999999989342, 4.187499999999998224 ) ) ;
#25768=ORIENTED_EDGE ( 'NONE', *, *, #26932, .F. ) ;
#25781=CARTESIAN_POINT ( 'NONE',  ( 98.15313185440925281, 4.458734125000016313, 2.500000001365592084 ) ) ;
#25783=CARTESIAN_POINT ( 'NONE',  ( 104.4587341249999781, 1.846868145590750521, 7.000000001365592972 ) ) ;
#25793=ORIENTED_EDGE ( 'NONE', *, *, #10798, .T. ) ;
#25799=CARTESIAN_POINT ( 'NONE',  ( 98.15313185440925281, 4.458734125000016313, 2.500000001365592084 ) ) ;
#25805=DIRECTION ( 'NONE',  ( -1.000000000000000000, 0.000000000000000000, 0.000000000000000000 ) ) ;
#25814=CARTESIAN_POINT ( 'NONE',  ( 94.99999999999995737, 1.387778780781445676E-14, 9.999999999999998224 ) ) ;
#25815=CARTESIAN_POINT ( 'NONE',  ( 95.54126587499996504, 1.387778780781445676E-14, 14.68750000136559208 ) ) ;
#25817=CARTESIAN_POINT ( 'NONE',  ( 96.84719886470459471, -3.152801135295355994, 5.562500001365591196 ) ) ;
#25828=CARTESIAN_POINT ( 'NONE',  ( 99.99999999999995737, 5.000000000000018652, 5.750000000000000000 ) ) ;
#25848=VERTEX_POINT ( 'NONE', #2669 ) ;
#25859=CARTESIAN_POINT ( 'NONE',  ( 94.99999999999995737, 1.387778780781445676E-14, 34.79898987322334136 ) ) ;
#25869=CARTESIAN_POINT ( 'NONE',  ( 104.9999999999999716, 1.449011120738813565E-14, 0.6250000027311856110 ) ) ;
#25873=PLANE ( 'NONE',  #24813 ) ;
#25874=( BOUNDED_CURVE ( )  B_SPLINE_CURVE ( 2, ( #3291, #18809, #12501, #14380, #11961, #9832, #18539, #27243, #5847 ),
 .UNSPECIFIED., .F., .F. ) 
 B_SPLINE_CURVE_WITH_KNOTS ( ( 3, 2, 2, 2, 3 ),
 ( 0.1428571428571428492, 0.1517857142857142738, 0.1607142857142857539, 0.1696428571428571785, 0.1785714285714286031 ),
 .UNSPECIFIED. ) 
 CURVE ( )  GEOMETRIC_REPRESENTATION_ITEM ( )  RATIONAL_B_SPLINE_CURVE ( ( 1.000000000000000000, 0.9238795325112867385, 1.000000000000000000, 0.9238795325112867385, 1.000000000000000000, 0.9238795325112867385, 1.000000000000000000, 0.9238795325112865164, 1.000000000000000222 ) ) 
 REPRESENTATION_ITEM ( '' )  );
#25886=CARTESIAN_POINT ( 'NONE',  ( 104.4587341249999781, 1.846868145590750299, 7.000000001365591196 ) ) ;
#25890=CARTESIAN_POINT ( 'NONE',  ( 95.54126587499995082, 1.846868145590750077, 10.37500000136559208 ) ) ;
#25912=CARTESIAN_POINT ( 'NONE',  ( 104.9999999999999716, 1.449011120738813565E-14, 6.499999999999999112 ) ) ;
#25913=CARTESIAN_POINT ( 'NONE',  ( 104.9999999999999716, 1.449011120738813565E-14, 1.499999999999999556 ) ) ;
#25921=CARTESIAN_POINT ( 'NONE',  ( 94.99999999999995737, 1.387778780781445676E-14, 0.5625000013655921949 ) ) ;
#25926=CARTESIAN_POINT ( 'NONE',  ( 96.84719886470459471, 3.152801135295383084, 3.562500001365592972 ) ) ;
#25928=CARTESIAN_POINT ( 'NONE',  ( 104.4587341249999781, -1.846868145590721655, 0.8750000013655925279 ) ) ;
#25942=CARTESIAN_POINT ( 'NONE',  ( 94.99999999999995737, 1.387778780781445676E-14, 34.79898987322334136 ) ) ;
#25943=CARTESIAN_POINT ( 'NONE',  ( 99.99999999999995737, 4.458734125000016313, 4.437500001365592084 ) ) ;
#25944=VERTEX_POINT ( 'NONE', #104 ) ;
#25958=CARTESIAN_POINT ( 'NONE',  ( 104.4587341249999781, -1.846868145590721655, 14.12500000136559208 ) ) ;
#25961=CARTESIAN_POINT ( 'NONE',  ( 99.99999999999995737, 4.458734125000016313, 3.187500001365592972 ) ) ;
#25963=CARTESIAN_POINT ( 'NONE',  ( 94.99999999999995737, 1.387778780781445676E-14, 1.125000002731184390 ) ) ;
#25966=CARTESIAN_POINT ( 'NONE',  ( 97.92893218813451028, 5.000000000000018652, 7.937500002731185056 ) ) ;
#25978=CARTESIAN_POINT ( 'NONE',  ( 98.15313185440925281, 4.458734125000016313, 14.50000000136559208 ) ) ;
#25981=AXIS2_PLACEMENT_3D ( 'NONE', #16812, #5989, #23374 ) ;
#25990=ORIENTED_EDGE ( 'NONE', *, *, #27781, .T. ) ;
#25993=CARTESIAN_POINT ( 'NONE',  ( 99.99999999999995737, -4.458734124999988779, 9.937500001365593860 ) ) ;
#26005=CARTESIAN_POINT ( 'NONE',  ( 103.5355339059327093, 3.535533905932755072, 0.7500000027311857220 ) ) ;
#26009=ADVANCED_FACE ( 'NONE', ( #7346, #16037 ), #20191, .F. ) ;
#26021=CARTESIAN_POINT ( 'NONE',  ( 95.54126587499995082, -1.846868145590724986, 10.50000000136559208 ) ) ;
#26024=CARTESIAN_POINT ( 'NONE',  ( 95.54126587499996504, 1.387778780781445676E-14, 11.43750000136559208 ) ) ;
#26039=CARTESIAN_POINT ( 'NONE',  ( 99.99999999999995737, 1.387778780781445676E-14, 34.79898987322334136 ) ) ;
#26048=CARTESIAN_POINT ( 'NONE',  ( 102.0710678118654329, -4.999999999999989342, 6.312499999999999112 ) ) ;
#26055=CARTESIAN_POINT ( 'NONE',  ( 102.0710678118654329, 5.000000000000018652, 6.687499999999999112 ) ) ;
#26058=CARTESIAN_POINT ( 'NONE',  ( 96.46446609406721961, -3.535533905932727539, 12.25000000273118594 ) ) ;
#26063=CARTESIAN_POINT ( 'NONE',  ( 99.99999999999995737, -4.458734124999988779, 0.9375000013655925279 ) ) ;
#26065=CARTESIAN_POINT ( 'NONE',  ( 101.8468681455907046, 4.458734125000016313, 3.125000001365592528 ) ) ;
#26068=CARTESIAN_POINT ( 'NONE',  ( 104.9999999999999716, 2.071067811865491937, 4.562500000000000000 ) ) ;
#26083=CARTESIAN_POINT ( 'NONE',  ( 95.54126587499996504, 1.387778780781445676E-14, 3.687500001365593416 ) ) ;
#26084=ORIENTED_EDGE ( 'NONE', *, *, #26446, .T. ) ;
#26097=CARTESIAN_POINT ( 'NONE',  ( 103.5355339059327093, 3.535533905932755072, 9.624999999999998224 ) ) ;
#26098=CARTESIAN_POINT ( 'NONE',  ( 104.4587341249999639, 1.442382525525748735E-14, 9.187500001365592084 ) ) ;
#26101=CARTESIAN_POINT ( 'NONE',  ( 95.54126587499995082, -1.846868145590724986, 1.500000001365591418 ) ) ;
#26103=CARTESIAN_POINT ( 'NONE',  ( 99.99999999999995737, 1.387778780781445676E-14, 0.000000000000000000 ) ) ;
#26115=CARTESIAN_POINT ( 'NONE',  ( 104.9999999999999716, 1.449011120738813565E-14, 9.625000002731184168 ) ) ;
#26117=CARTESIAN_POINT ( 'NONE',  ( 104.4587341249999639, 1.442382525525748735E-14, 14.18750000136559208 ) ) ;
#26133=CARTESIAN_POINT ( 'NONE',  ( 96.84719886470459471, -3.152801135295355994, 11.81250000136559208 ) ) ;
#26146=CARTESIAN_POINT ( 'NONE',  ( 99.99999999999995737, -4.999999999999990230, 0.3750000027311853890 ) ) ;
#26151=( NAMED_UNIT ( * ) PLANE_ANGLE_UNIT ( ) SI_UNIT ( $, .RADIAN. ) );
#26161=VECTOR ( 'NONE', #5241, 1000.000000000000000 ) ;
#26163=CARTESIAN_POINT ( 'NONE',  ( 103.1528011352953342, 3.152801135295383084, 7.062500001365592084 ) ) ;
#26166=CARTESIAN_POINT ( 'NONE',  ( 103.1528011352953342, -3.152801135295355106, 10.81250000136559208 ) ) ;
#26179=CARTESIAN_POINT ( 'NONE',  ( 104.9999999999999716, -2.071067811865452857, 8.437500000000000000 ) ) ;
#26187=CARTESIAN_POINT ( 'NONE',  ( 96.46446609406721961, 3.535533905932755072, 3.875000000000000000 ) ) ;
#26191=AXIS2_PLACEMENT_3D ( 'NONE', #17275, #10576, #8725 ) ;
#26209=CARTESIAN_POINT ( 'NONE',  ( 99.99999999999995737, 4.458734125000016313, 3.187500001365592972 ) ) ;
#26228=CARTESIAN_POINT ( 'NONE',  ( 96.84719886470459471, -3.152801135295355994, 3.812500001365591640 ) ) ;
#26229=ORIENTED_EDGE ( 'NONE', *, *, #14634, .F. ) ;
#26243=CARTESIAN_POINT ( 'NONE',  ( 99.99999999999995737, 4.458734125000016313, 12.43750000136559208 ) ) ;
#26245=CARTESIAN_POINT ( 'NONE',  ( 101.8468681455907046, 4.458734125000016313, 13.12500000136559208 ) ) ;
#26255=LINE ( 'NONE', #8717, #14966 ) ;
#26275=EDGE_CURVE ( 'NONE', #2879, #11095, #12196, .T. ) ;
#26280=CARTESIAN_POINT ( 'NONE',  ( 96.84719886470459471, -3.152801135295355994, 9.812500001365593860 ) ) ;
#26300=DIRECTION ( 'NONE',  ( -0.000000000000000000, -0.000000000000000000, -1.000000000000000000 ) ) ;
#26305=DIRECTION ( 'NONE',  ( 1.000000000000000000, 0.000000000000000000, 0.000000000000000000 ) ) ;
#26310=CARTESIAN_POINT ( 'NONE',  ( 95.54126587499996504, 1.387778780781445676E-14, 10.43750000136559208 ) ) ;
#26313=CARTESIAN_POINT ( 'NONE',  ( 104.4587341249999781, -1.846868145590721655, 11.87500000136559031 ) ) ;
#26339=CARTESIAN_POINT ( 'NONE',  ( 96.46446609406721961, -3.535533905932727539, 2.124999999999998224 ) ) ;
#26357=CARTESIAN_POINT ( 'NONE',  ( 99.99999999999995737, 4.458734125000016313, 1.187500001365592750 ) ) ;
#26360=CARTESIAN_POINT ( 'NONE',  ( 97.92893218813451028, 5.000000000000018652, 4.812500000000000000 ) ) ;
#26371=ADVANCED_BREP_SHAPE_REPRESENTATION ( '', ( #26591, #26844 ), #20877 ) ;
#26375=CARTESIAN_POINT ( 'NONE',  ( 104.9999999999999574, 2.071067811865491937, 13.56250000000000000 ) ) ;
#26381=( BOUNDED_CURVE ( )  B_SPLINE_CURVE ( 2, ( #3925, #3506, #21308, #12311, #23173, #12167, #27589, #1791, #10457 ),
 .UNSPECIFIED., .F., .F. ) 
 B_SPLINE_CURVE_WITH_KNOTS ( ( 3, 2, 2, 2, 3 ),
 ( 0.6071428571428570953, 0.6160714285714286031, 0.6250000000000000000, 0.6339285714285712858, 0.6428571428571427937 ),
 .UNSPECIFIED. ) 
 CURVE ( )  GEOMETRIC_REPRESENTATION_ITEM ( )  RATIONAL_B_SPLINE_CURVE ( ( 1.000000000000000000, 0.9238795325112867385, 1.000000000000000000, 0.9238795325112867385, 1.000000000000000000, 0.9238795325112867385, 1.000000000000000000, 0.9238795325112877377, 0.9999999999999990008 ) ) 
 REPRESENTATION_ITEM ( '' )  );
#26392=CARTESIAN_POINT ( 'NONE',  ( 103.1528011352953342, 3.152801135295383084, 10.31250000136559208 ) ) ;
#26394=CARTESIAN_POINT ( 'NONE',  ( 98.15313185440923860, -4.458734124999987891, 12.62500000136559208 ) ) ;
#26408=CARTESIAN_POINT ( 'NONE',  ( 96.84719886470459471, 3.152801135295383084, 13.56250000136559386 ) ) ;
#26423=VERTEX_POINT ( 'NONE', #26115 ) ;
#26426=CARTESIAN_POINT ( 'NONE',  ( 96.84719886470459471, 3.152801135295383084, 11.56250000136559208 ) ) ;
#26438=VERTEX_POINT ( 'NONE', #4595 ) ;
#26443=CARTESIAN_POINT ( 'NONE',  ( 99.99999999999995737, 1.387778780781445676E-14, 34.79898987322334136 ) ) ;
#26445=CARTESIAN_POINT ( 'NONE',  ( 102.0710678118654329, -4.999999999999989342, 1.437500002731185056 ) ) ;
#26446=EDGE_CURVE ( 'NONE', #26438, #25528, #10200, .T. ) ;
#26450=CARTESIAN_POINT ( 'NONE',  ( 104.9999999999999574, 2.071067811865501263, 10.56249999999999645 ) ) ;
#26454=ORIENTED_EDGE ( 'NONE', *, *, #26275, .T. ) ;
#26457=CARTESIAN_POINT ( 'NONE',  ( 101.8468681455906903, 4.458734125000016313, 4.125000001365592084 ) ) ;
#26460=CARTESIAN_POINT ( 'NONE',  ( 98.15313185440925281, 4.458734125000016313, 7.250000001365591196 ) ) ;
#26477=CARTESIAN_POINT ( 'NONE',  ( 99.99999999999995737, 5.000000000000018652, 8.875000002731184168 ) ) ;
#26490=CARTESIAN_POINT ( 'NONE',  ( 99.99999999999995737, -4.999999999999990230, 10.37500000273118594 ) ) ;
#26498=CARTESIAN_POINT ( 'NONE',  ( 98.15313185440925281, -4.458734124999987891, 0.8750000013655926390 ) ) ;
#26501=CARTESIAN_POINT ( 'NONE',  ( 98.15313185440923860, -4.458734124999987891, 1.625000001365591862 ) ) ;
#26507=EDGE_LOOP ( 'NONE', ( #22240, #11741, #12149, #14304 ) ) ;
#26517=AXIS2_PLACEMENT_3D ( 'NONE', #22458, #19885, #22172 ) ;
#26518=CARTESIAN_POINT ( 'NONE',  ( 94.99999999999995737, -2.071067811865466624, 12.06250000000000000 ) ) ;
#26531=CARTESIAN_POINT ( 'NONE',  ( 95.54126587499995082, -1.846868145590724986, 9.750000001365593860 ) ) ;
#26533=CARTESIAN_POINT ( 'NONE',  ( 98.15313185440925281, -4.458734124999987891, 1.625000001365591640 ) ) ;
#26549=CARTESIAN_POINT ( 'NONE',  ( 96.84719886470459471, 3.152801135295383084, 9.562500001365593860 ) ) ;
#26567=CARTESIAN_POINT ( 'NONE',  ( 104.4587341249999639, 1.442382525525748735E-14, 12.18750000136559208 ) ) ;
#26590=CARTESIAN_POINT ( 'NONE',  ( 103.5355339059327093, -3.535533905932726206, 5.500000002731185056 ) ) ;
#26591=MANIFOLD_SOLID_BREP ( 'Thread1', #12590 ) ;
#26598=EDGE_CURVE ( 'NONE', #27592, #9857, #20974, .T. ) ;
#26600=CARTESIAN_POINT ( 'NONE',  ( 104.4587341249999781, 1.846868145590750299, 3.000000001365592528 ) ) ;
#26603=CARTESIAN_POINT ( 'NONE',  ( 104.4587341249999781, -1.846868145590721655, 8.875000001365593860 ) ) ;
#26623=CARTESIAN_POINT ( 'NONE',  ( 94.99999999999995737, -2.071067811865466624, 8.187500002731185944 ) ) ;
#26626=CARTESIAN_POINT ( 'NONE',  ( 103.5355339059327093, 3.535533905932755072, 14.62500000000000000 ) ) ;
#26628=CARTESIAN_POINT ( 'NONE',  ( 97.92893218813451028, -4.999999999999989342, 1.187499999999999334 ) ) ;
#26637=CARTESIAN_POINT ( 'NONE',  ( 99.99999999999995737, 5.000000000000018652, 12.75000000000000000 ) ) ;
#26644=CARTESIAN_POINT ( 'NONE',  ( 102.0710678118654329, -4.999999999999989342, 4.437500002731185944 ) ) ;
#26656=CARTESIAN_POINT ( 'NONE',  ( 94.99999999999997158, 2.071067811865471953, 5.937500000000001776 ) ) ;
#26665=CARTESIAN_POINT ( 'NONE',  ( 104.9999999999999574, 2.071067811865491937, 14.56249999999999822 ) ) ;
#26678=CARTESIAN_POINT ( 'NONE',  ( 104.4587341249999781, -1.846868145590721655, 11.12500000136559386 ) ) ;
#26680=CARTESIAN_POINT ( 'NONE',  ( 96.84719886470459471, -3.152801135295355994, 13.56250000136559208 ) ) ;
#26687=ORIENTED_EDGE ( 'NONE', *, *, #5102, .F. ) ;
#26693=CARTESIAN_POINT ( 'NONE',  ( 95.54126587499995082, -1.846868145590724986, 12.75000000136559386 ) ) ;
#26709=ORIENTED_EDGE ( 'NONE', *, *, #27487, .F. ) ;
#26711=CARTESIAN_POINT ( 'NONE',  ( 95.54126587499996504, 1.846868145590750077, 5.625000001365592972 ) ) ;
#26712=( BOUNDED_CURVE ( )  B_SPLINE_CURVE ( 2, ( #11399, #22115, #20118, #596, #6704, #9276, #17689, #21838, #8709, #21974, #15245, #2451, #2168, #15392, #26680, #10830, #4445, #7128, #23824, #23966, #4303, #26245, #12960, #21694, #8996, #17541, #2314, #19546, #13097, #26394, #6848, #10971, #15537, #4728, #19683, #13388, #2595, #27111, #20404, #13962, #13681, #20255, #26970, #9703, #22687, #20691, #16109, #1174, #5297, #3157, #740, #5584, #24814, #11968, #9839, #7561, #9414, #11827, #12100, #16401, #27250, #14249, #18546, #7414, #22970, #18404, #13818, #18113, #20551, #7273, #1032, #22398, #16255, #18685, #2867, #24678, #3434, #15825, #26827, #7707, #9973, #25099, #20827, #24955, #889, #22542, #1304, #27388, #9560, #5440, #5155, #14108, #22832, #15964, #3298, #24530, #5016, #18263, #11538, #3010, #11681, #18950, #1721, #5992, #12657, #8121, #21382, #25513, #14527, #16942, #14657, #12796, #3850, #12381, #23655, #25377, #27933, #10661, #10104, #25783, #1861, #10526, #19090, #19232, #16816, #19369, #16542, #8392, #18817, #17081, #23378, #12511, #6261, #8255, #14934, #25232, #14792, #4131, #3579, #21515, #1994, #1448, #5723, #7847, #23515, #16678, #14388, #27799, #23105, #12236, #20965, #27524, #7980, #5857, #21239, #23242, #3719, #10383, #25643, #21099, #1587, #10242, #3994, #27659, #6127, #19939, #15505, #132, #22083, #2560, #11221, #418, #4410, #22223, #19792, #19512, #8961, #2703, #11081, #13065, #26209, #26065, #4267, #10938, #21944, #6671, #4694, #8818, #13355, #17507, #6534, #17649, #15357, #4842, #24072, #21802, #15652, #17369, #9104, #11362, #2134, #2422, #4549, #17798, #274, #26501, #13210, #28072, #8537, #6957, #10799, #24351, #26357, #6815, #13503, #24215, #17223, #25928, #6403, #15072, #23790, #12926, #21658, #8130, #8679 ),
 .UNSPECIFIED., .F., .F. ) 
 B_SPLINE_CURVE_WITH_KNOTS ( ( 3, 2, 2, 2, 2, 2, 2, 2, 2, 2, 2, 2, 2, 2, 2, 2, 2, 2, 2, 2, 2, 2, 2, 2, 2, 2, 2, 2, 2, 2, 2, 2, 2, 2, 2, 2, 2, 2, 2, 2, 2, 2, 2, 2, 2, 2, 2, 2, 2, 2, 2, 2, 2, 2, 2, 2, 2, 2, 2, 2, 2, 2, 2, 2, 2, 2, 2, 2, 2, 2, 2, 2, 2, 2, 2, 2, 2, 2, 2, 2, 2, 2, 2, 2, 2, 2, 2, 2, 2, 2, 2, 2, 2, 2, 2, 2, 2, 2, 2, 2, 2, 2, 2, 2, 2, 2, 2, 2, 2, 2, 2, 2, 3 ),
 ( 0.000000000000000000, 0.008928571428571428076, 0.01785714285714285615, 0.02678571428571428423, 0.03571428571428571230, 0.04464285714285714385, 0.05357142857142856845, 0.06250000000000000000, 0.07142857142857142461, 0.08035714285714286309, 0.08928571428571428770, 0.09821428571428571230, 0.1071428571428571369, 0.1160714285714285754, 0.1250000000000000000, 0.1339285714285714246, 0.1428571428571428492, 0.1517857142857142738, 0.1607142857142857262, 0.1696428571428571508, 0.1785714285714285754, 0.1875000000000000000, 0.1964285714285714246, 0.2053571428571428492, 0.2142857142857142738, 0.2232142857142857262, 0.2321428571428571508, 0.2410714285714285754, 0.2500000000000000000, 0.2589285714285714524, 0.2678571428571428492, 0.2767857142857143016, 0.2857142857142856984, 0.2946428571428571508, 0.3035714285714285476, 0.3125000000000000000, 0.3214285714285714524, 0.3303571428571428492, 0.3392857142857143016, 0.3482142857142856984, 0.3571428571428571508, 0.3660714285714285476, 0.3750000000000000000, 0.3839285714285714524, 0.3928571428571428492, 0.4017857142857143016, 0.4107142857142856984, 0.4196428571428571508, 0.4285714285714285476, 0.4375000000000000000, 0.4464285714285714524, 0.4553571428571428492, 0.4642857142857143016, 0.4732142857142856984, 0.4821428571428571508, 0.4910714285714285476, 0.5000000000000000000, 0.5089285714285713969, 0.5178571428571429047, 0.5267857142857143016, 0.5357142857142856984, 0.5446428571428570953, 0.5535714285714286031, 0.5625000000000000000, 0.5714285714285713969, 0.5803571428571429047, 0.5892857142857143016, 0.5982142857142856984, 0.6071428571428570953, 0.6160714285714286031, 0.6250000000000000000, 0.6339285714285713969, 0.6428571428571429047, 0.6517857142857143016, 0.6607142857142856984, 0.6696428571428570953, 0.6785714285714286031, 0.6875000000000000000, 0.6964285714285713969, 0.7053571428571429047, 0.7142857142857143016, 0.7232142857142856984, 0.7321428571428570953, 0.7410714285714286031, 0.7500000000000000000, 0.7589285714285713969, 0.7678571428571429047, 0.7767857142857143016, 0.7857142857142856984, 0.7946428571428570953, 0.8035714285714286031, 0.8125000000000000000, 0.8214285714285713969, 0.8303571428571429047, 0.8392857142857143016, 0.8482142857142856984, 0.8571428571428570953, 0.8660714285714286031, 0.8750000000000000000, 0.8839285714285713969, 0.8928571428571429047, 0.9017857142857143016, 0.9107142857142856984, 0.9196428571428570953, 0.9285714285714286031, 0.9375000000000000000, 0.9464285714285713969, 0.9553571428571429047, 0.9642857142857143016, 0.9732142857142856984, 0.9821428571428570953, 0.9910714285714286031, 1.000000000000000000 ),
 .UNSPECIFIED. ) 
 CURVE ( )  GEOMETRIC_REPRESENTATION_ITEM ( )  RATIONAL_B_SPLINE_CURVE ( ( 1.000000000000000000, 0.9238795325112867385, 1.000000000000000000, 0.9238795325112867385, 1.000000000000000000, 0.9238795325112867385, 1.000000000000000000, 0.9238795325112867385, 1.000000000000000000, 0.9238795325112867385, 1.000000000000000000, 0.9238795325112867385, 1.000000000000000000, 0.9238795325112867385, 1.000000000000000000, 0.9238795325112867385, 1.000000000000000000, 0.9238795325112867385, 1.000000000000000000, 0.9238795325112867385, 1.000000000000000000, 0.9238795325112867385, 1.000000000000000000, 0.9238795325112867385, 1.000000000000000000, 0.9238795325112867385, 1.000000000000000000, 0.9238795325112867385, 1.000000000000000000, 0.9238795325112867385, 1.000000000000000000, 0.9238795325112867385, 1.000000000000000000, 0.9238795325112867385, 1.000000000000000000, 0.9238795325112867385, 1.000000000000000000, 0.9238795325112867385, 1.000000000000000000, 0.9238795325112867385, 1.000000000000000000, 0.9238795325112867385, 1.000000000000000000, 0.9238795325112867385, 1.000000000000000000, 0.9238795325112867385, 1.000000000000000000, 0.9238795325112867385, 1.000000000000000000, 0.9238795325112867385, 1.000000000000000000, 0.9238795325112867385, 1.000000000000000000, 0.9238795325112867385, 1.000000000000000000, 0.9238795325112867385, 1.000000000000000000, 0.9238795325112867385, 1.000000000000000000, 0.9238795325112867385, 1.000000000000000000, 0.9238795325112867385, 1.000000000000000000, 0.9238795325112867385, 1.000000000000000000, 0.9238795325112867385, 1.000000000000000000, 0.9238795325112867385, 1.000000000000000000, 0.9238795325112867385, 1.000000000000000000, 0.9238795325112867385, 1.000000000000000000, 0.9238795325112867385, 1.000000000000000000, 0.9238795325112867385, 1.000000000000000000, 0.9238795325112867385, 1.000000000000000000, 0.9238795325112867385, 1.000000000000000000, 0.9238795325112867385, 1.000000000000000000, 0.9238795325112867385, 1.000000000000000000, 0.9238795325112867385, 1.000000000000000000, 0.9238795325112867385, 1.000000000000000000, 0.9238795325112867385, 1.000000000000000000, 0.9238795325112867385, 1.000000000000000000, 0.9238795325112867385, 1.000000000000000000, 0.9238795325112867385, 1.000000000000000000, 0.9238795325112867385, 1.000000000000000000, 0.9238795325112867385, 1.000000000000000000, 0.9238795325112867385, 1.000000000000000000, 0.9238795325112867385, 1.000000000000000000, 0.9238795325112867385, 1.000000000000000000, 0.9238795325112867385, 1.000000000000000000, 0.9238795325112867385, 1.000000000000000000, 0.9238795325112867385, 1.000000000000000000, 0.9238795325112867385, 1.000000000000000000, 0.9238795325112867385, 1.000000000000000000, 0.9238795325112867385, 1.000000000000000000, 0.9238795325112867385, 1.000000000000000000, 0.9238795325112867385, 1.000000000000000000, 0.9238795325112867385, 1.000000000000000000, 0.9238795325112867385, 1.000000000000000000, 0.9238795325112867385, 1.000000000000000000, 0.9238795325112867385, 1.000000000000000000, 0.9238795325112867385, 1.000000000000000000, 0.9238795325112867385, 1.000000000000000000, 0.9238795325112867385, 1.000000000000000000, 0.9238795325112867385, 1.000000000000000000, 0.9238795325112867385, 1.000000000000000000, 0.9238795325112867385, 1.000000000000000000, 0.9238795325112867385, 1.000000000000000000, 0.9238795325112867385, 1.000000000000000000, 0.9238795325112867385, 1.000000000000000000, 0.9238795325112867385, 1.000000000000000000, 0.9238795325112867385, 1.000000000000000000, 0.9238795325112867385, 1.000000000000000000, 0.9238795325112867385, 1.000000000000000000, 0.9238795325112867385, 1.000000000000000000, 0.9238795325112867385, 1.000000000000000000, 0.9238795325112867385, 1.000000000000000000, 0.9238795325112867385, 1.000000000000000000, 0.9238795325112867385, 1.000000000000000000, 0.9238795325112867385, 1.000000000000000000, 0.9238795325112867385, 1.000000000000000000, 0.9238795325112867385, 1.000000000000000000, 0.9238795325112867385, 1.000000000000000000, 0.9238795325112867385, 1.000000000000000000, 0.9238795325112867385, 1.000000000000000000, 0.9238795325112867385, 1.000000000000000000, 0.9238795325112867385, 1.000000000000000000, 0.9238795325112867385, 1.000000000000000000, 0.9238795325112867385, 1.000000000000000000, 0.9238795325112867385, 1.000000000000000000, 0.9238795325112867385, 1.000000000000000000, 0.9238795325112867385, 1.000000000000000000, 0.9238795325112867385, 1.000000000000000000, 0.9238795325112867385, 1.000000000000000000, 0.9238795325112867385, 1.000000000000000000, 0.9238795325112867385, 1.000000000000000000, 0.9238795325112867385, 1.000000000000000000, 0.9238795325112867385, 1.000000000000000000, 0.9238795325112867385, 1.000000000000000000, 0.9238795325112867385, 1.000000000000000000, 0.9238795325112867385, 1.000000000000000000, 0.9238795325112867385, 1.000000000000000000, 0.9238795325112867385, 1.000000000000000000, 0.9238795325112867385, 1.000000000000000000, 0.9238795325112867385, 1.000000000000000000, 0.9238795325112867385, 1.000000000000000000, 0.9238795325112867385, 1.000000000000000000, 0.9238795325112867385, 1.000000000000000000 ) ) 
 REPRESENTATION_ITEM ( '' )  );
#26723=VERTEX_POINT ( 'NONE', #17138 ) ;
#26730=VERTEX_POINT ( 'NONE', #1774 ) ;
#26732=CARTESIAN_POINT ( 'NONE',  ( 96.46446609406721961, -3.535533905932727539, 5.250000002731184168 ) ) ;
#26738=CARTESIAN_POINT ( 'NONE',  ( 94.99999999999995737, 1.387778780781445676E-14, 2.125000002731185056 ) ) ;
#26742=CARTESIAN_POINT ( 'NONE',  ( 98.15313185440925281, 4.458734125000016313, 5.250000001365592972 ) ) ;
#26745=CARTESIAN_POINT ( 'NONE',  ( 95.54126587499996504, 1.387778780781445676E-14, 8.437500001365592084 ) ) ;
#26760=CARTESIAN_POINT ( 'NONE',  ( 94.99999999999997158, -2.071067811865486608, 8.062500000000000000 ) ) ;
#26763=CARTESIAN_POINT ( 'NONE',  ( 102.0710678118654329, 5.000000000000018652, 9.812500002731184168 ) ) ;
#26788=CARTESIAN_POINT ( 'NONE',  ( 104.9999999999999716, 1.449011120738813565E-14, 4.625000002731185944 ) ) ;
#26808=CARTESIAN_POINT ( 'NONE',  ( 97.92893218813451028, -4.999999999999989342, 14.18749999999999822 ) ) ;
#26825=CARTESIAN_POINT ( 'NONE',  ( 96.84719886470459471, 3.152801135295383084, 7.562500001365592084 ) ) ;
#26827=CARTESIAN_POINT ( 'NONE',  ( 96.84719886470459471, -3.152801135295355994, 9.562500001365593860 ) ) ;
#26840=CARTESIAN_POINT ( 'NONE',  ( 99.99999999999995737, -4.458734124999988779, 9.937500001365593860 ) ) ;
#26844=AXIS2_PLACEMENT_3D ( 'NONE', #8635, #24028, #23608 ) ;
#26860=CARTESIAN_POINT ( 'NONE',  ( 98.15313185440923860, -4.458734124999987891, 5.875000001365592084 ) ) ;
#26884=( BOUNDED_CURVE ( )  B_SPLINE_CURVE ( 2, ( #17882, #24297, #651, #20028, #11306, #18020, #2918, #14015, #24583 ),
 .UNSPECIFIED., .F., .T. ) 
 B_SPLINE_CURVE_WITH_KNOTS ( ( 3, 2, 2, 2, 3 ),
 ( 0.2142857142857142183, 0.2232142857142856707, 0.2321428571428570953, 0.2410714285714285199, 0.2499999999999999445 ),
 .UNSPECIFIED. ) 
 CURVE ( )  GEOMETRIC_REPRESENTATION_ITEM ( )  RATIONAL_B_SPLINE_CURVE ( ( 1.000000000000000444, 0.9238795325112862944, 1.000000000000000000, 0.9238795325112867385, 1.000000000000000000, 0.9238795325112867385, 1.000000000000000000, 0.9238795325112871826, 0.9999999999999995559 ) ) 
 REPRESENTATION_ITEM ( '' )  );
#26886=DIRECTION ( 'NONE',  ( -1.000000000000000000, 0.000000000000000000, 0.000000000000000000 ) ) ;
#26888=CARTESIAN_POINT ( 'NONE',  ( 98.15313185440925281, -4.458734124999987891, 6.625000001365592084 ) ) ;
#26891=CARTESIAN_POINT ( 'NONE',  ( 95.54126587499995082, -1.846868145590724986, 7.500000001365592084 ) ) ;
#26895=CARTESIAN_POINT ( 'NONE',  ( 97.92893218813451028, -4.999999999999989342, 5.187500000000000000 ) ) ;
#26907=CARTESIAN_POINT ( 'NONE',  ( 103.5355339059327093, 3.535533905932755072, 8.750000002731184168 ) ) ;
#26924=FACE_OUTER_BOUND ( 'NONE', #11566, .T. ) ;
#26932=EDGE_CURVE ( 'NONE', #23574, #12833, #4928, .T. ) ;
#26933=CARTESIAN_POINT ( 'NONE',  ( 94.99999999999997158, -2.071067811865486608, 4.187500002731185944 ) ) ;
#26954=CARTESIAN_POINT ( 'NONE',  ( 97.92893218813451028, 5.000000000000018652, 14.81249999999999822 ) ) ;
#26960=CARTESIAN_POINT ( 'NONE',  ( 104.9999999999999574, 2.071067811865491937, 12.68750000273118772 ) ) ;
#26968=CARTESIAN_POINT ( 'NONE',  ( 104.4587341249999781, -1.846868145590721655, 5.125000001365592972 ) ) ;
#26970=CARTESIAN_POINT ( 'NONE',  ( 103.1528011352953342, -3.152801135295355106, 11.81250000136559208 ) ) ;
#26972=CARTESIAN_POINT ( 'NONE',  ( 104.9999999999999716, 1.449011120738813565E-14, 3.499999999999999556 ) ) ;
#26977=( BOUNDED_CURVE ( )  B_SPLINE_CURVE ( 2, ( #3571, #27380, #20819, #8246, #23233, #5577, #16934, #1578, #25634 ),
 .UNSPECIFIED., .F., .F. ) 
 B_SPLINE_CURVE_WITH_KNOTS ( ( 3, 2, 2, 2, 3 ),
 ( 0.2499999999999999445, 0.2589285714285713969, 0.2678571428571427937, 0.2767857142857143016, 0.2857142857142856984 ),
 .UNSPECIFIED. ) 
 CURVE ( )  GEOMETRIC_REPRESENTATION_ITEM ( )  RATIONAL_B_SPLINE_CURVE ( ( 1.000000000000000444, 0.9238795325112862944, 1.000000000000000000, 0.9238795325112867385, 1.000000000000000000, 0.9238795325112867385, 1.000000000000000000, 0.9238795325112867385, 1.000000000000000000 ) ) 
 REPRESENTATION_ITEM ( '' )  );
#26984=CARTESIAN_POINT ( 'NONE',  ( 95.54126587499996504, 1.387778780781445676E-14, 9.687500001365593860 ) ) ;
#26999=CARTESIAN_POINT ( 'NONE',  ( 101.8468681455907046, -4.458734124999987891, 6.000000001365592084 ) ) ;
#27023=DIRECTION ( 'NONE',  ( -0.000000000000000000, -0.000000000000000000, -1.000000000000000000 ) ) ;
#27031=CARTESIAN_POINT ( 'NONE',  ( 96.84719886470459471, -3.152801135295355994, 4.562500001365592084 ) ) ;
#27034=CARTESIAN_POINT ( 'NONE',  ( 95.54126587499996504, 1.387778780781445676E-14, 9.437500001365593860 ) ) ;
#27037=AXIS2_PLACEMENT_3D ( 'NONE', #7080, #15776, #24482 ) ;
#27048=CARTESIAN_POINT ( 'NONE',  ( 97.92893218813451028, 5.000000000000018652, 4.937500002731185056 ) ) ;
#27092=FACE_OUTER_BOUND ( 'NONE', #11052, .T. ) ;
#27093=CARTESIAN_POINT ( 'NONE',  ( 97.92893218813451028, 5.000000000000018652, 8.812499999999998224 ) ) ;
#27097=ADVANCED_FACE ( 'NONE', ( #9130 ), #13532, .F. ) ;
#27099=CARTESIAN_POINT ( 'NONE',  ( 96.46446609406721961, 3.535533905932755072, 12.00000000273118594 ) ) ;
#27108=CARTESIAN_POINT ( 'NONE',  ( 95.54126587499996504, 1.387778780781445676E-14, 5.687500001365591196 ) ) ;
#27111=CARTESIAN_POINT ( 'NONE',  ( 101.8468681455907046, 4.458734125000016313, 12.12500000136559208 ) ) ;
#27114=CARTESIAN_POINT ( 'NONE',  ( 102.0710678118654329, -4.999999999999989342, 4.312499999999999112 ) ) ;
#27125=CARTESIAN_POINT ( 'NONE',  ( 104.4587341249999639, 1.442382525525748735E-14, 10.18750000136559208 ) ) ;
#27140=EDGE_CURVE ( 'NONE', #949, #5414, #26977, .T. ) ;
#27144=CARTESIAN_POINT ( 'NONE',  ( 104.4587341249999639, 1.442382525525748735E-14, 5.187500001365592972 ) ) ;
#27145=( BOUNDED_CURVE ( )  B_SPLINE_CURVE ( 2, ( #12700, #26656, #4992, #23558, #25828, #4035, #21425, #10570, #21563 ),
 .UNSPECIFIED., .F., .F. ) 
 B_SPLINE_CURVE_WITH_KNOTS ( ( 3, 2, 2, 2, 3 ),
 ( 0.6428571428571427937, 0.6517857142857141906, 0.6607142857142855874, 0.6696428571428569843, 0.6785714285714284921 ),
 .UNSPECIFIED. ) 
 CURVE ( )  GEOMETRIC_REPRESENTATION_ITEM ( )  RATIONAL_B_SPLINE_CURVE ( ( 1.000000000000000888, 0.9238795325112857393, 1.000000000000000000, 0.9238795325112867385, 1.000000000000000000, 0.9238795325112867385, 1.000000000000000000, 0.9238795325112877377, 0.9999999999999990008 ) ) 
 REPRESENTATION_ITEM ( '' )  );
#27150=ORIENTED_EDGE ( 'NONE', *, *, #17356, .F. ) ;
#27159=VERTEX_POINT ( 'NONE', #19081 ) ;
#27176=CARTESIAN_POINT ( 'NONE',  ( 99.99999999999995737, 4.458734125000016313, 13.43750000136559386 ) ) ;
#27178=CARTESIAN_POINT ( 'NONE',  ( 104.9999999999999716, 1.449011120738813565E-14, 12.62500000273118594 ) ) ;
#27195=CARTESIAN_POINT ( 'NONE',  ( 96.46446609406721961, 3.535533905932755072, 5.000000002731185944 ) ) ;
#27200=CARTESIAN_POINT ( 'NONE',  ( 106.9999999999999716, 1.473504056721760595E-14, 34.79898987322334136 ) ) ;
#27235=CARTESIAN_POINT ( 'NONE',  ( 97.92893218813451028, 5.000000000000018652, 10.81250000000000000 ) ) ;
#27240=CARTESIAN_POINT ( 'NONE',  ( 94.99999999999995737, 2.071067811865491048, 12.06250000273118772 ) ) ;
#27241=CARTESIAN_POINT ( 'NONE',  ( 94.99999999999995737, 1.387778780781445676E-14, 2.999999999999999112 ) ) ;
#27243=CARTESIAN_POINT ( 'NONE',  ( 104.9999999999999858, 2.071067811865486608, 11.68750000273118417 ) ) ;
#27248=CARTESIAN_POINT ( 'NONE',  ( 98.15313185440925281, -4.458734124999987891, 5.875000001365591196 ) ) ;
#27250=CARTESIAN_POINT ( 'NONE',  ( 99.99999999999995737, -4.458734124999988779, 10.68750000136559208 ) ) ;
#27253=CARTESIAN_POINT ( 'NONE',  ( 104.9999999999999716, 1.449011120738813565E-14, 9.500000000000000000 ) ) ;
#27265=CARTESIAN_POINT ( 'NONE',  ( 104.4587341249999639, 1.442382525525748735E-14, 6.187500001365592084 ) ) ;
#27280=CARTESIAN_POINT ( 'NONE',  ( 95.54126587499996504, -1.846868145590724986, 5.750000001365591196 ) ) ;
#27282=CARTESIAN_POINT ( 'NONE',  ( 94.99999999999995737, 1.387778780781445676E-14, 8.125000002731185944 ) ) ;
#27289=EDGE_CURVE ( 'NONE', #16160, #18726, #25874, .T. ) ;
#27294=VERTEX_POINT ( 'NONE', #16533 ) ;
#27298=CARTESIAN_POINT ( 'NONE',  ( 99.99999999999995737, 1.387778780781445676E-14, 34.79898987322334136 ) ) ;
#27306=( BOUNDED_CURVE ( )  B_SPLINE_CURVE ( 2, ( #27253, #7983, #21102, #12104, #14111, #20694, #27527, #14392, #3301 ),
 .UNSPECIFIED., .F., .F. ) 
 B_SPLINE_CURVE_WITH_KNOTS ( ( 3, 2, 2, 2, 3 ),
 ( 0.3928571428571428492, 0.4017857142857143016, 0.4107142857142856984, 0.4196428571428571508, 0.4285714285714285476 ),
 .UNSPECIFIED. ) 
 CURVE ( )  GEOMETRIC_REPRESENTATION_ITEM ( )  RATIONAL_B_SPLINE_CURVE ( ( 1.000000000000000000, 0.9238795325112867385, 1.000000000000000000, 0.9238795325112867385, 1.000000000000000000, 0.9238795325112867385, 1.000000000000000000, 0.9238795325112867385, 1.000000000000000000 ) ) 
 REPRESENTATION_ITEM ( '' )  );
#27312=CARTESIAN_POINT ( 'NONE',  ( 95.54126587499995082, 1.846868145590750077, 1.375000001365592972 ) ) ;
#27328=CARTESIAN_POINT ( 'NONE',  ( 94.99999999999995737, -2.071067811865466624, 7.187500002731185944 ) ) ;
#27346=CARTESIAN_POINT ( 'NONE',  ( 95.54126587499996504, 1.387778780781445676E-14, 13.43750000136559386 ) ) ;
#27354=CARTESIAN_POINT ( 'NONE',  ( 96.46446609406721961, 3.535533905932755072, 3.000000002731185944 ) ) ;
#27370=ORIENTED_EDGE ( 'NONE', *, *, #24954, .T. ) ;
#27371=CARTESIAN_POINT ( 'NONE',  ( 102.0710678118654329, 5.000000000000018652, 8.687499999999998224 ) ) ;
#27376=CARTESIAN_POINT ( 'NONE',  ( 102.0710678118654329, 5.000000000000018652, 0.8125000027311859441 ) ) ;
#27380=CARTESIAN_POINT ( 'NONE',  ( 104.9999999999999716, -2.071067811865452857, 11.43749999999999822 ) ) ;
#27386=CARTESIAN_POINT ( 'NONE',  ( 101.8468681455906903, 4.458734125000016313, 7.375000001365592084 ) ) ;
#27388=CARTESIAN_POINT ( 'NONE',  ( 104.4587341249999781, 1.846868145590750521, 9.000000001365592084 ) ) ;
#27391=CARTESIAN_POINT ( 'NONE',  ( 104.9999999999999716, -2.071067811865462627, 4.437500000000000000 ) ) ;
#27400=CARTESIAN_POINT ( 'NONE',  ( 98.15313185440925281, 4.458734125000016313, 5.500000001365592972 ) ) ;
#27411=CARTESIAN_POINT ( 'NONE',  ( 95.54126587499996504, 1.387778780781445676E-14, 3.687500001365593416 ) ) ;
#27420=CARTESIAN_POINT ( 'NONE',  ( 102.0710678118654329, -4.999999999999989342, 3.437500002731184612 ) ) ;
#27427=DIRECTION ( 'NONE',  ( -0.000000000000000000, -0.000000000000000000, -1.000000000000000000 ) ) ;
#27442=CARTESIAN_POINT ( 'NONE',  ( 104.4587341249999781, 1.846868145590750299, 2.000000001365591640 ) ) ;
#27463=CARTESIAN_POINT ( 'NONE',  ( 102.0710678118654329, -4.999999999999989342, 7.437500002731186832 ) ) ;
#27473=DIRECTION ( 'NONE',  ( 0.000000000000000000, 0.000000000000000000, 1.000000000000000000 ) ) ;
#27482=CARTESIAN_POINT ( 'NONE',  ( 99.99999999999995737, -4.458734124999988779, 12.68750000136559208 ) ) ;
#27487=EDGE_CURVE ( 'NONE', #11744, #14666, #1501, .T. ) ;
#27507=CARTESIAN_POINT ( 'NONE',  ( 103.5355339059327093, -3.535533905932726206, 7.375000000000000000 ) ) ;
#27514=CYLINDRICAL_SURFACE ( 'NONE', #9952, 5.000000000000004441 ) ;
#27522=CARTESIAN_POINT ( 'NONE',  ( 95.54126587499996504, 1.387778780781445676E-14, 3.687500001365593416 ) ) ;
#27524=CARTESIAN_POINT ( 'NONE',  ( 104.4587341249999781, 1.846868145590750521, 5.000000001365592972 ) ) ;
#27527=CARTESIAN_POINT ( 'NONE',  ( 96.46446609406721961, -3.535533905932727539, 9.125000000000000000 ) ) ;
#27537=CARTESIAN_POINT ( 'NONE',  ( 104.4587341249999781, 1.846868145590750299, 8.250000001365592084 ) ) ;
#27538=ORIENTED_EDGE ( 'NONE', *, *, #15207, .T. ) ;
#27551=CARTESIAN_POINT ( 'NONE',  ( 95.54126587499995082, -1.846868145590724986, 2.500000001365592084 ) ) ;
#27552=CARTESIAN_POINT ( 'NONE',  ( 99.99999999999995737, 1.387778780781445676E-14, 34.79898987322334136 ) ) ;
#27553=CARTESIAN_POINT ( 'NONE',  ( 103.1528011352953342, 3.152801135295383084, 1.312500001365592750 ) ) ;
#27556=CARTESIAN_POINT ( 'NONE',  ( 104.9999999999999716, 1.449011120738813565E-14, 7.625000002731185056 ) ) ;
#27561=CARTESIAN_POINT ( 'NONE',  ( 96.46446609406721961, -3.535533905932727539, 3.250000002731184612 ) ) ;
#27565=CARTESIAN_POINT ( 'NONE',  ( 104.9999999999999716, 1.449011120738813565E-14, 6.625000002731185944 ) ) ;
#27566=EDGE_LOOP ( 'NONE', ( #2149, #25990 ) ) ;
#27568=FACE_OUTER_BOUND ( 'NONE', #12391, .T. ) ;
#27569=CARTESIAN_POINT ( 'NONE',  ( 99.99999999999995737, 1.387778780781445676E-14, 34.79898987322334136 ) ) ;
#27570=ORIENTED_EDGE ( 'NONE', *, *, #10878, .T. ) ;
#27578=DIRECTION ( 'NONE',  ( -0.000000000000000000, -0.000000000000000000, -1.000000000000000000 ) ) ;
#27580=ORIENTED_EDGE ( 'NONE', *, *, #5382, .T. ) ;
#27583=CARTESIAN_POINT ( 'NONE',  ( 101.8468681455907046, 4.458734125000016313, 13.37500000136559386 ) ) ;
#27589=CARTESIAN_POINT ( 'NONE',  ( 96.46446609406721961, -3.535533905932727539, 6.124999999999998224 ) ) ;
#27590=CARTESIAN_POINT ( 'NONE',  ( 104.9999999999999716, 1.449011120738813565E-14, 34.79898987322334136 ) ) ;
#27592=VERTEX_POINT ( 'NONE', #21790 ) ;
#27595=CARTESIAN_POINT ( 'NONE',  ( 103.5355339059327093, 3.535533905932755072, 6.750000002731185056 ) ) ;
#27597=EDGE_CURVE ( 'NONE', #15231, #162, #11875, .T. ) ;
#27599=EDGE_CURVE ( 'NONE', #13106, #27745, #27716, .T. ) ;
#27617=CARTESIAN_POINT ( 'NONE',  ( 101.8468681455906903, -4.458734124999987891, 11.75000000136559208 ) ) ;
#27622=CARTESIAN_POINT ( 'NONE',  ( 94.99999999999995737, 1.387778780781445676E-14, 9.000000000000000000 ) ) ;
#27633=ORIENTED_EDGE ( 'NONE', *, *, #10878, .F. ) ;
#27643=CARTESIAN_POINT ( 'NONE',  ( 104.9999999999999574, -2.071067811865462627, 10.43749999999999822 ) ) ;
#27657=CARTESIAN_POINT ( 'NONE',  ( 101.8468681455906903, -4.458734124999987891, 3.000000001365592528 ) ) ;
#27659=CARTESIAN_POINT ( 'NONE',  ( 98.15313185440923860, 4.458734125000016313, 4.250000001365592084 ) ) ;
#27673=CARTESIAN_POINT ( 'NONE',  ( 103.1528011352953342, -3.152801135295355106, 7.062500001365592972 ) ) ;
#27689=CARTESIAN_POINT ( 'NONE',  ( 98.15313185440925281, -4.458734124999987891, 3.625000001365591640 ) ) ;
#27692=CARTESIAN_POINT ( 'NONE',  ( 99.99999999999995737, -4.458734124999988779, 1.937500001365591640 ) ) ;
#27710=CARTESIAN_POINT ( 'NONE',  ( 104.9999999999999716, 1.449011120738813565E-14, 1.625000002731184834 ) ) ;
#27716=( BOUNDED_CURVE ( )  B_SPLINE_CURVE ( 2, ( #19359, #8529, #2960, #7225, #26490, #24632, #6947, #11209, #9234 ),
 .UNSPECIFIED., .F., .F. ) 
 B_SPLINE_CURVE_WITH_KNOTS ( ( 3, 2, 2, 2, 3 ),
 ( 0.2499999999999999445, 0.2589285714285713969, 0.2678571428571427937, 0.2767857142857143016, 0.2857142857142856984 ),
 .UNSPECIFIED. ) 
 CURVE ( )  GEOMETRIC_REPRESENTATION_ITEM ( )  RATIONAL_B_SPLINE_CURVE ( ( 1.000000000000000444, 0.9238795325112862944, 1.000000000000000000, 0.9238795325112867385, 1.000000000000000000, 0.9238795325112867385, 1.000000000000000000, 0.9238795325112867385, 1.000000000000000000 ) ) 
 REPRESENTATION_ITEM ( '' )  );
#27728=DIRECTION ( 'NONE',  ( -1.000000000000000000, 0.000000000000000000, 0.000000000000000000 ) ) ;
#27736=CARTESIAN_POINT ( 'NONE',  ( 103.5355339059327093, -3.535533905932726206, 0.5000000027311855000 ) ) ;
#27742=CARTESIAN_POINT ( 'NONE',  ( 103.5355339059327093, -3.535533905932726206, 9.500000002731184168 ) ) ;
#27745=VERTEX_POINT ( 'NONE', #3111 ) ;
#27752=CARTESIAN_POINT ( 'NONE',  ( 101.8468681455906903, 4.458734125000016313, 11.12500000136559386 ) ) ;
#27758=VECTOR ( 'NONE', #16451, 1000.000000000000000 ) ;
#27779=CARTESIAN_POINT ( 'NONE',  ( 104.9999999999999574, 2.071067811865491937, 3.562500000000000000 ) ) ;
#27781=EDGE_CURVE ( 'NONE', #25436, #9633, #8148, .T. ) ;
#27783=CARTESIAN_POINT ( 'NONE',  ( 96.46446609406721961, 3.535533905932755072, 14.00000000273118594 ) ) ;
#27792=ADVANCED_FACE ( 'NONE', ( #26924 ), #22211, .F. ) ;
#27796=CARTESIAN_POINT ( 'NONE',  ( 103.1528011352953342, -3.152801135295355106, 5.062500001365592972 ) ) ;
#27799=CARTESIAN_POINT ( 'NONE',  ( 98.15313185440923860, 4.458734125000016313, 5.250000001365592972 ) ) ;
#27800=CARTESIAN_POINT ( 'NONE',  ( 104.9999999999999716, 1.449011120738813565E-14, 10.62500000273118594 ) ) ;
#27802=FACE_OUTER_BOUND ( 'NONE', #21221, .T. ) ;
#27806=VERTEX_POINT ( 'NONE', #18064 ) ;
#27816=CARTESIAN_POINT ( 'NONE',  ( 104.4587341249999639, 1.442382525525748735E-14, 5.187500001365592972 ) ) ;
#27831=CARTESIAN_POINT ( 'NONE',  ( 103.1528011352953342, -3.152801135295355106, 4.812500001365592084 ) ) ;
#27833=CARTESIAN_POINT ( 'NONE',  ( 98.15313185440923860, 4.458734125000016313, 1.500000001365592972 ) ) ;
#27844=CARTESIAN_POINT ( 'NONE',  ( 97.92893218813451028, -4.999999999999989342, 6.312500002731185056 ) ) ;
#27860=( LENGTH_UNIT ( ) NAMED_UNIT ( * ) SI_UNIT ( .MILLI., .METRE. ) );
#27873=CARTESIAN_POINT ( 'NONE',  ( 94.99999999999995737, 1.387778780781445676E-14, 1.125000002731184390 ) ) ;
#27890=CARTESIAN_POINT ( 'NONE',  ( 103.1528011352953342, 3.152801135295383084, 13.06250000136559208 ) ) ;
#27894=CARTESIAN_POINT ( 'NONE',  ( 104.4587341249999639, 1.442382525525748735E-14, 10.93750000136559208 ) ) ;
#27898=CARTESIAN_POINT ( 'NONE',  ( 94.99999999999995737, 2.071067811865491493, 3.062500002731185944 ) ) ;
#27902=CARTESIAN_POINT ( 'NONE',  ( 96.46446609406721961, 3.535533905932755072, 11.87500000000000000 ) ) ;
#27918=CARTESIAN_POINT ( 'NONE',  ( 102.0710678118654329, -4.999999999999989342, 4.312500000000000000 ) ) ;
#27931=CARTESIAN_POINT ( 'NONE',  ( 104.4587341249999639, 1.442382525525748735E-14, 4.187500001365592084 ) ) ;
#27933=CARTESIAN_POINT ( 'NONE',  ( 99.99999999999995737, 4.458734125000016313, 7.187500001365592084 ) ) ;
#27947=ADVANCED_FACE ( 'NONE', ( #7803 ), #23332, .F. ) ;
#27949=CARTESIAN_POINT ( 'NONE',  ( 96.84719886470459471, 3.152801135295383084, 3.562500001365592972 ) ) ;
#27956=CYLINDRICAL_SURFACE ( 'NONE', #21292, 5.000000000000004441 ) ;
#27965=CARTESIAN_POINT ( 'NONE',  ( 104.4587341249999781, -1.846868145590721655, 1.875000001365591862 ) ) ;
#27967=CARTESIAN_POINT ( 'NONE',  ( 95.54126587499996504, 1.387778780781445676E-14, 2.437500001365592084 ) ) ;
#27969=CARTESIAN_POINT ( 'NONE',  ( 98.15313185440923860, -4.458734124999987891, 4.875000001365592084 ) ) ;
#27985=CARTESIAN_POINT ( 'NONE',  ( 95.27063293749995410, 1.387778780781445676E-14, 0.2812500020483886254 ) ) ;
#28013=CARTESIAN_POINT ( 'NONE',  ( 104.9999999999999574, -2.071067811865462627, 3.562500002731184612 ) ) ;
#28029=CARTESIAN_POINT ( 'NONE',  ( 101.8468681455906903, 4.458734125000016313, 9.125000001365592084 ) ) ;
#28033=CARTESIAN_POINT ( 'NONE',  ( 104.4587341249999639, 1.442382525525748735E-14, 11.93750000136559208 ) ) ;
#28042=CARTESIAN_POINT ( 'NONE',  ( 104.9999999999999716, 1.449011120738813565E-14, 8.499999999999998224 ) ) ;
#28055=CARTESIAN_POINT ( 'NONE',  ( 104.9999999999999574, -2.071067811865462627, 6.437499999999999112 ) ) ;
#28056=CARTESIAN_POINT ( 'NONE',  ( 97.92893218813451028, 5.000000000000018652, 1.812500000000000000 ) ) ;
#28061=CARTESIAN_POINT ( 'NONE',  ( 102.0710678118654329, 5.000000000000018652, 4.812500002731185056 ) ) ;
#28069=CARTESIAN_POINT ( 'NONE',  ( 101.8468681455906903, -4.458734124999987891, 2.000000001365591640 ) ) ;
#28071=ADVANCED_FACE ( 'NONE', ( #25469 ), #8073, .F. ) ;
#28072=CARTESIAN_POINT ( 'NONE',  ( 95.54126587499996504, -1.846868145590724986, 1.500000001365591196 ) ) ;
#28079=ORIENTED_EDGE ( 'NONE', *, *, #2181, .F. ) ;
#28089=CARTESIAN_POINT ( 'NONE',  ( 103.1528011352953342, -3.152801135295355106, 1.062500001365592528 ) ) ;
#28090=ORIENTED_EDGE ( 'NONE', *, *, #3570, .F. ) ;
#28103=CARTESIAN_POINT ( 'NONE',  ( 98.15313185440925281, -4.458734124999987891, 1.625000001365591640 ) ) ;
#28105=CARTESIAN_POINT ( 'NONE',  ( 101.8468681455906903, 4.458734125000016313, 3.125000001365592528 ) ) ;
#28121=CARTESIAN_POINT ( 'NONE',  ( 96.84719886470459471, 3.152801135295383084, 14.56250000136559208 ) ) ;
#28133=ORIENTED_EDGE ( 'NONE', *, *, #12967, .F. ) ;
#28136=CARTESIAN_POINT ( 'NONE',  ( 104.4587341249999639, 1.442382525525748735E-14, 10.18750000136559208 ) ) ;
#28137=EDGE_CURVE ( 'NONE', #7853, #23118, #13021, .T. ) ;
#28142=CARTESIAN_POINT ( 'NONE',  ( 97.92893218813451028, -4.999999999999989342, 12.18750000000000000 ) ) ;
#28150=CARTESIAN_POINT ( 'NONE',  ( 96.46446609406721961, 3.535533905932755072, 1.000000002731185944 ) ) ;
#28165=VECTOR ( 'NONE', #16559, 1000.000000000000000 ) ;
#28168=CARTESIAN_POINT ( 'NONE',  ( 104.4587341249999781, 1.846868145590750299, 9.000000001365593860 ) ) ;
#28170=CARTESIAN_POINT ( 'NONE',  ( 101.8468681455906903, 4.458734125000016313, 13.12500000136559208 ) ) ;
#28193=CARTESIAN_POINT ( 'NONE',  ( 94.99999999999995737, 2.071067811865491048, 3.937500000000000000 ) ) ;
ENDSEC;
END-ISO-10303-21;
